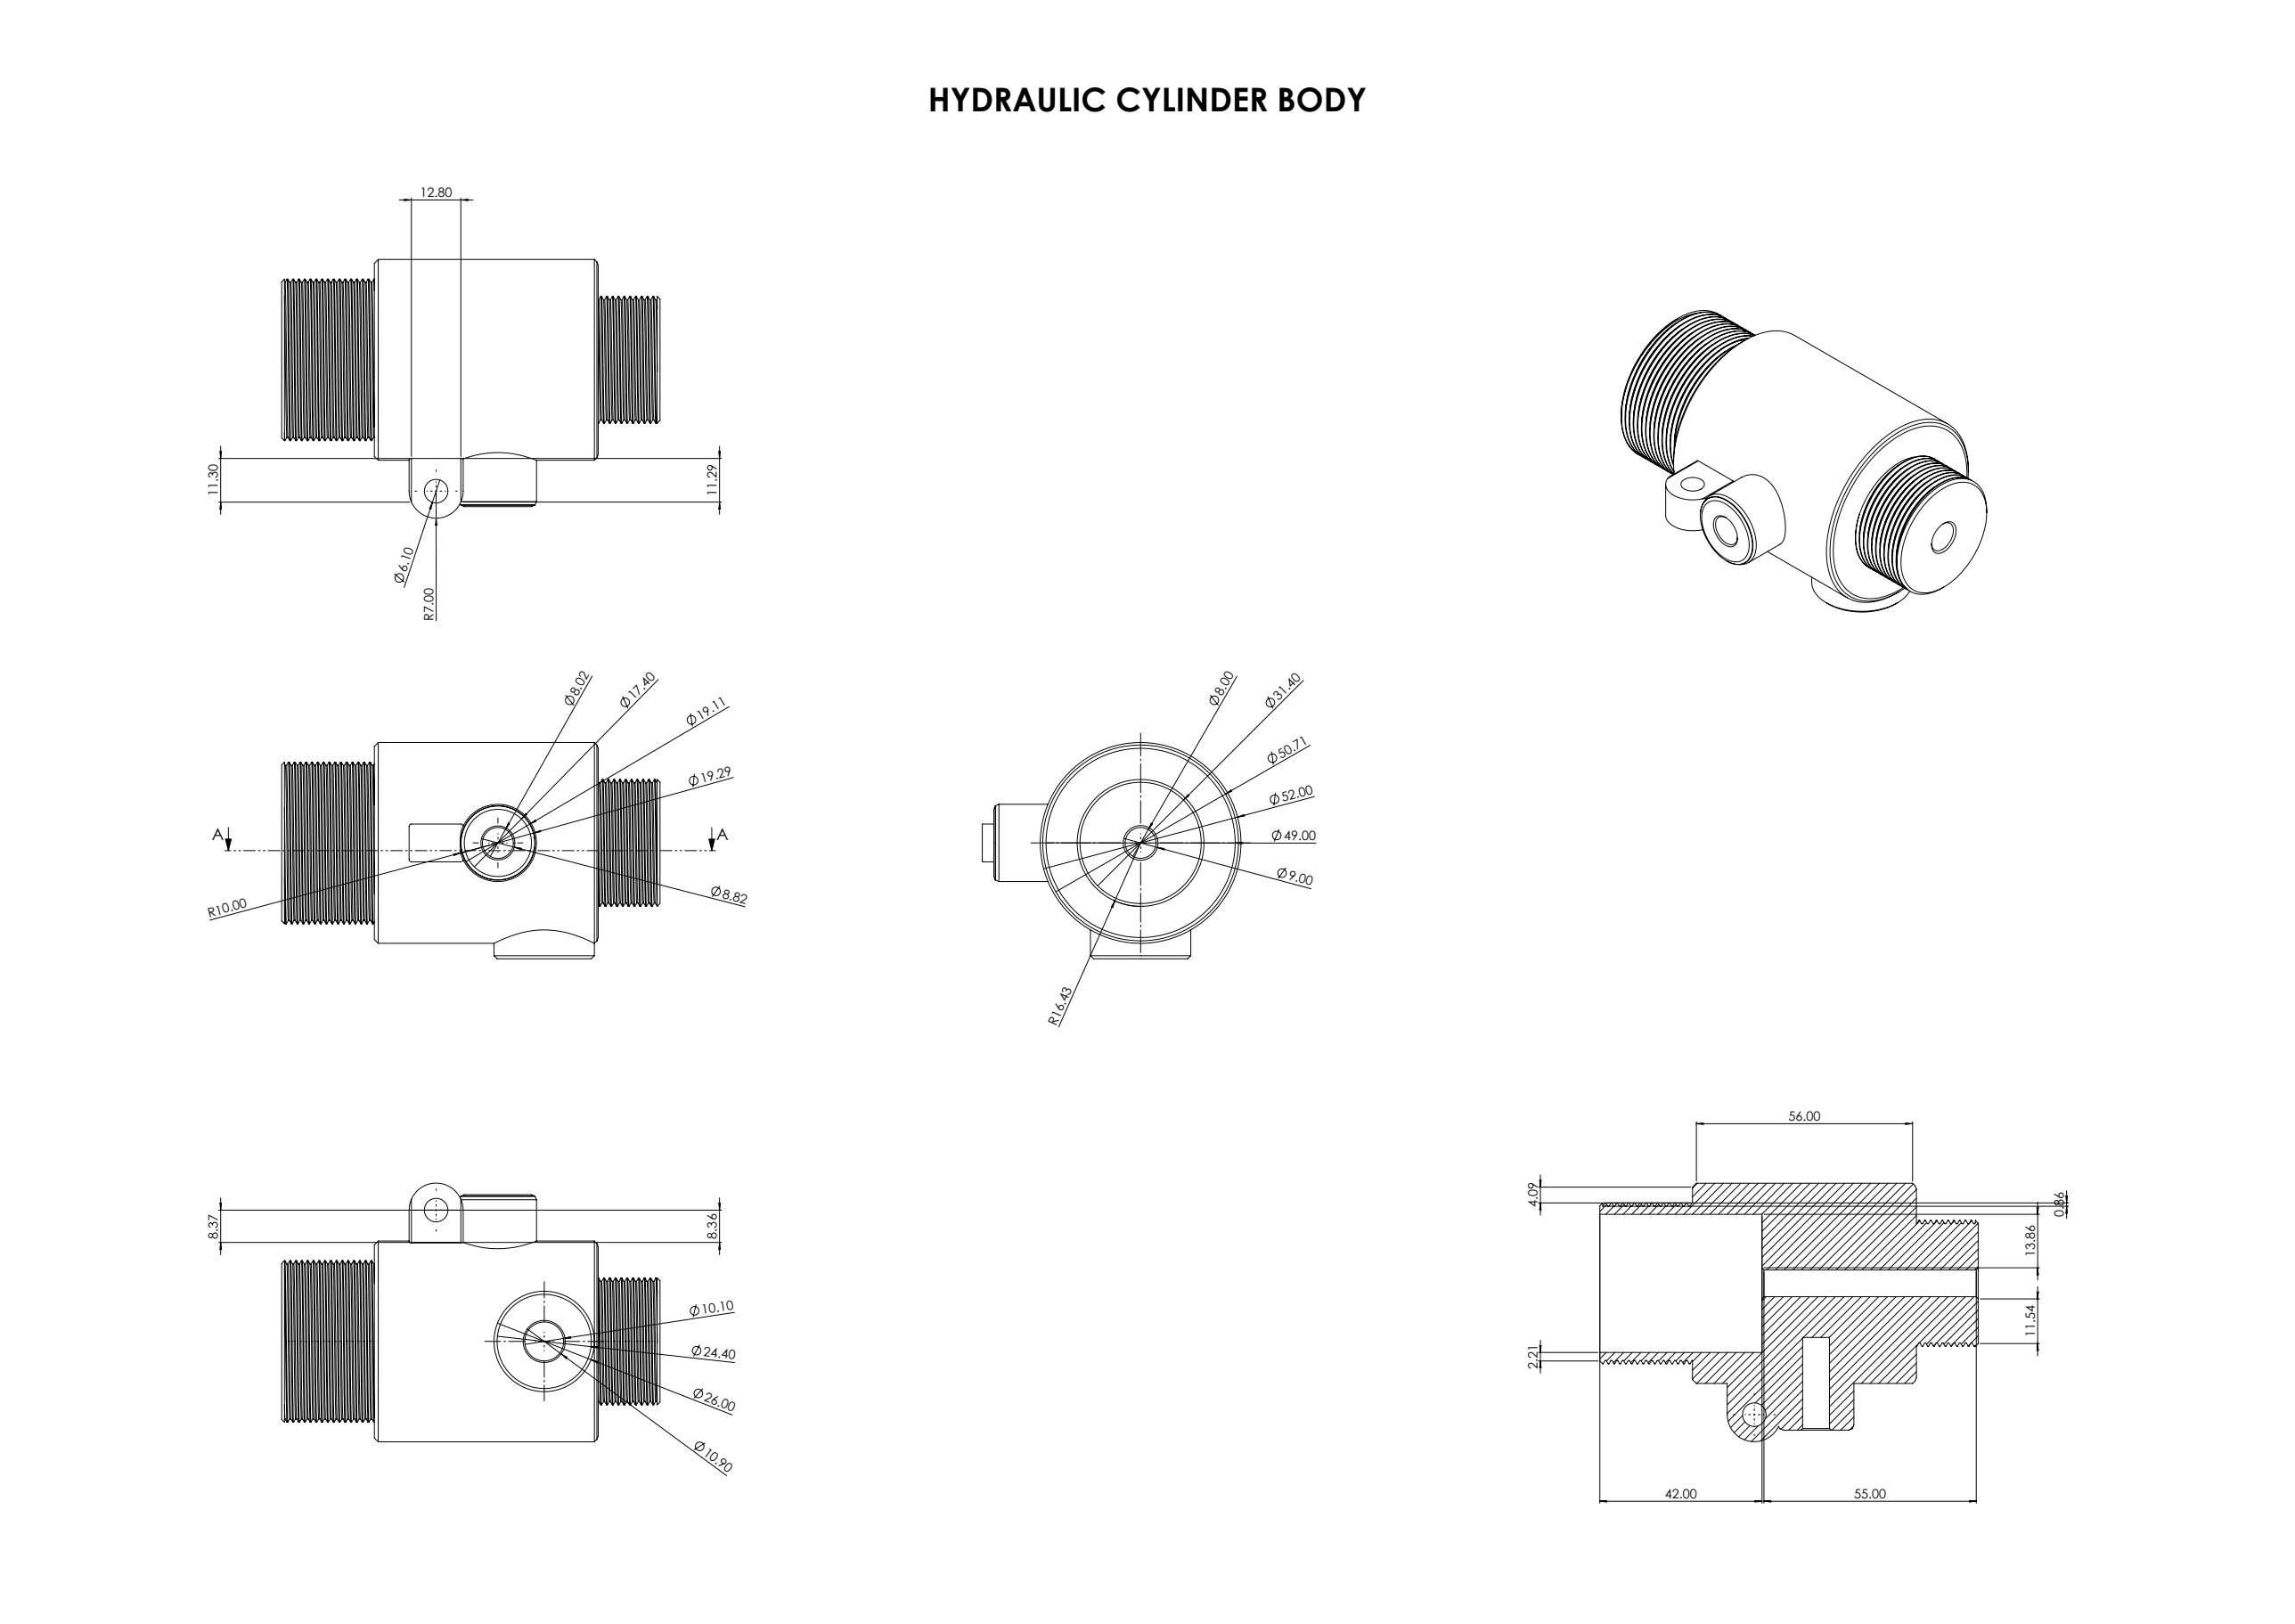
ISO-10303-21;
HEADER;
/* Generated by software containing ST-Developer
 * from STEP Tools, Inc. (www.steptools.com) 
 */

FILE_DESCRIPTION(
/* description */ (''),
/* implementation_level */ '2;1');

FILE_NAME(
/* name */ '02_Hydraulic_Cylinder_Body.step',
/* time_stamp */ '2026-10-26T03:55:20-07:00',
/* author */ (''),
/* organization */ (''),
/* preprocessor_version */ 'ST-DEVELOPER v20.2',
/* originating_system */ 'Autodesk Translation Framework v15.15.0.0',
/* authorisation */ '');

FILE_SCHEMA (('AUTOMOTIVE_DESIGN { 1 0 10303 214 3 1 1 }'));
ENDSEC;

DATA;
#10=MECHANICAL_DESIGN_GEOMETRIC_PRESENTATION_REPRESENTATION('',(#176),#45236);
#136=SHAPE_REPRESENTATION_RELATIONSHIP('SRR','None',#45315,#156);
#156=ADVANCED_BREP_SHAPE_REPRESENTATION('',(#196),#45217);
#176=STYLED_ITEM('',(#45463),#196);
#196=MANIFOLD_SOLID_BREP('Body1',#16518);
#350=B_SPLINE_CURVE_WITH_KNOTS('',3,(#23915,#23916,#23917,#23918,#23919,
#23920,#23921,#23922,#23923,#23924,#23925,#23926,#23927,#23928,#23929,#23930),
 .UNSPECIFIED.,.F.,.F.,(4,3,3,3,3,4),(-4.09299088010945,-3.98286471232789,
-3.4850066232869,-2.98714853424591,-2.48929044520493,-2.07752579179387),
 .UNSPECIFIED.);
#351=B_SPLINE_CURVE_WITH_KNOTS('',3,(#23933,#23934,#23935,#23936,#23937,
#23938,#23939,#23940,#23941,#23942),.UNSPECIFIED.,.F.,.F.,(4,3,3,4),(0.,
0.497858089040978,0.99571617808196,1.12612756527411),.UNSPECIFIED.);
#352=B_SPLINE_CURVE_WITH_KNOTS('',3,(#23947,#23948,#23949,#23950,#23951,
#23952,#23953,#23954,#23955,#23956,#23957,#23958,#23959,#23960,#23961,#23962,
#23963,#23964,#23965,#23966,#23967,#23968,#23969,#23970,#23971,#23972,#23973,
#23974,#23975,#23976,#23977,#23978,#23979,#23980,#23981,#23982,#23983,#23984,
#23985,#23986),.UNSPECIFIED.,.F.,.F.,(4,3,3,3,3,3,3,3,3,3,3,3,3,4),(-10.376176187289,
-9.95716178081971,-9.45930369177872,-8.96144560273774,-8.46358751369675,
-7.96572942465577,-7.46787133561478,-6.9700132465738,-6.47215515753281,
-5.97429706849183,-5.47643897945084,-4.97858089040986,-4.48072280136887,
-4.09299088010945),.UNSPECIFIED.);
#353=B_SPLINE_CURVE_WITH_KNOTS('',3,(#23987,#23988,#23989,#23990,#23991,
#23992,#23993,#23994,#23995,#23996,#23997,#23998,#23999,#24000,#24001,#24002,
#24003,#24004,#24005,#24006,#24007,#24008,#24009,#24010,#24011,#24012,#24013,
#24014,#24015,#24016,#24017,#24018,#24019,#24020,#24021,#24022,#24023,#24024,
#24025,#24026),.UNSPECIFIED.,.F.,.F.,(4,3,3,3,3,3,3,3,3,3,3,3,3,4),(1.12612756527411,
1.49357426712295,1.99143235616393,2.48929044520492,2.98714853424591,3.48500662328689,
3.98286471232788,4.48072280136887,4.97858089040986,5.47643897945084,5.97429706849183,
6.47215515753282,6.9700132465738,7.40931287245371),.UNSPECIFIED.);
#354=B_SPLINE_CURVE_WITH_KNOTS('',3,(#24031,#24032,#24033,#24034,#24035,
#24036,#24037,#24038,#24039,#24040,#24041,#24042,#24043,#24044,#24045,#24046,
#24047,#24048,#24049,#24050,#24051,#24052,#24053,#24054,#24055,#24056,#24057,
#24058,#24059,#24060,#24061,#24062,#24063,#24064,#24065,#24066,#24067,#24068,
#24069,#24070,#24071,#24072,#24073),.UNSPECIFIED.,.F.,.F.,(4,3,3,3,3,3,
3,3,3,3,3,3,3,3,4),(-16.6593614944686,-16.4293169383525,-15.9314588493115,
-15.4336007602705,-14.9357426712296,-14.4378845821886,-13.9400264931476,
-13.4421684041066,-12.9443103150656,-12.4464522260246,-11.9485941369836,
-11.4507360479427,-10.9528779589017,-10.4550198698607,-10.376176187289),
 .UNSPECIFIED.);
#355=B_SPLINE_CURVE_WITH_KNOTS('',3,(#24074,#24075,#24076,#24077,#24078,
#24079,#24080,#24081,#24082,#24083,#24084,#24085,#24086,#24087,#24088,#24089,
#24090,#24091,#24092,#24093,#24094,#24095,#24096,#24097,#24098,#24099,#24100,
#24101,#24102,#24103,#24104,#24105,#24106,#24107,#24108,#24109,#24110,#24111,
#24112,#24113,#24114,#24115,#24116),.UNSPECIFIED.,.F.,.F.,(4,3,3,3,3,3,
3,3,3,3,3,3,3,3,4),(7.40931287245371,7.46787133561479,7.96572942465578,
8.46358751369676,8.96144560273774,9.45930369177873,9.95716178081971,10.4550198698607,
10.9528779589017,11.4507360479427,11.9485941369836,12.4464522260246,12.9443103150656,
13.4421684041066,13.6924981796333),.UNSPECIFIED.);
#356=B_SPLINE_CURVE_WITH_KNOTS('',3,(#24121,#24122,#24123,#24124,#24125,
#24126,#24127,#24128,#24129,#24130,#24131,#24132,#24133,#24134,#24135,#24136,
#24137,#24138,#24139,#24140,#24141,#24142,#24143,#24144,#24145,#24146,#24147,
#24148,#24149,#24150,#24151,#24152,#24153,#24154,#24155,#24156,#24157,#24158,
#24159,#24160,#24161,#24162,#24163),.UNSPECIFIED.,.F.,.F.,(4,3,3,3,3,3,
3,3,3,3,3,3,3,3,4),(-22.9425468016482,-22.9014720958853,-22.4036140068443,
-21.9057559178034,-21.4078978287624,-20.9100397397214,-20.4121816506804,
-19.9143235616394,-19.4164654725984,-18.9186073835574,-18.4207492945165,
-17.9228912054755,-17.4250331164345,-16.9271750273935,-16.6593614944686),
 .UNSPECIFIED.);
#357=B_SPLINE_CURVE_WITH_KNOTS('',3,(#24164,#24165,#24166,#24167,#24168,
#24169,#24170,#24171,#24172,#24173,#24174,#24175,#24176,#24177,#24178,#24179,
#24180,#24181,#24182,#24183,#24184,#24185,#24186,#24187,#24188,#24189,#24190,
#24191,#24192,#24193,#24194,#24195,#24196,#24197,#24198,#24199,#24200,#24201,
#24202,#24203,#24204,#24205,#24206),.UNSPECIFIED.,.F.,.F.,(4,3,3,3,3,3,
3,3,3,3,3,3,3,3,4),(13.6924981796333,13.9400264931476,14.4378845821886,
14.9357426712296,15.4336007602705,15.9314588493115,16.4293169383525,16.9271750273935,
17.4250331164345,17.9228912054755,18.4207492945165,18.9186073835575,19.4164654725984,
19.9143235616394,19.9756834868129),.UNSPECIFIED.);
#358=B_SPLINE_CURVE_WITH_KNOTS('',3,(#24211,#24212,#24213,#24214,#24215,
#24216,#24217,#24218,#24219,#24220,#24221,#24222,#24223,#24224,#24225,#24226,
#24227,#24228,#24229,#24230,#24231,#24232,#24233,#24234,#24235,#24236,#24237,
#24238,#24239,#24240,#24241,#24242,#24243,#24244,#24245,#24246,#24247,#24248,
#24249,#24250),.UNSPECIFIED.,.F.,.F.,(4,3,3,3,3,3,3,3,3,3,3,3,3,4),(-29.2257321088278,
-28.8757691643771,-28.3779110753362,-27.8800529862952,-27.3821948972542,
-26.8843368082132,-26.3864787191722,-25.8886206301312,-25.3907625410903,
-24.8929044520493,-24.3950463630083,-23.8971882739673,-23.3993301849263,
-22.9425468016482),.UNSPECIFIED.);
#359=B_SPLINE_CURVE_WITH_KNOTS('',3,(#24251,#24252,#24253,#24254,#24255,
#24256,#24257,#24258,#24259,#24260,#24261,#24262,#24263,#24264,#24265,#24266,
#24267,#24268,#24269,#24270,#24271,#24272,#24273,#24274,#24275,#24276,#24277,
#24278,#24279,#24280,#24281,#24282,#24283,#24284,#24285,#24286,#24287,#24288,
#24289,#24290),.UNSPECIFIED.,.F.,.F.,(4,3,3,3,3,3,3,3,3,3,3,3,3,4),(19.9756834868129,
20.4121816506804,20.9100397397214,21.4078978287624,21.9057559178034,22.4036140068443,
22.9014720958853,23.3993301849263,23.8971882739673,24.3950463630083,24.8929044520493,
25.3907625410903,25.8886206301312,26.2588687939925),.UNSPECIFIED.);
#360=B_SPLINE_CURVE_WITH_KNOTS('',3,(#24295,#24296,#24297,#24298,#24299,
#24300,#24301,#24302,#24303,#24304,#24305,#24306,#24307,#24308,#24309,#24310,
#24311,#24312,#24313,#24314,#24315,#24316,#24317,#24318,#24319,#24320,#24321,
#24322,#24323,#24324,#24325,#24326,#24327,#24328,#24329,#24330,#24331,#24332,
#24333,#24334,#24335,#24336,#24337),.UNSPECIFIED.,.F.,.F.,(4,3,3,3,3,3,
3,3,3,3,3,3,3,3,4),(-35.5089174160074,-35.34792432191,-34.850066232869,
-34.352208143828,-33.854350054787,-33.356491965746,-32.858633876705,-32.3607757876641,
-31.8629176986231,-31.3650596095821,-30.8672015205411,-30.3693434315001,
-29.8714853424591,-29.3736272534181,-29.2257321088278),.UNSPECIFIED.);
#361=B_SPLINE_CURVE_WITH_KNOTS('',3,(#24338,#24339,#24340,#24341,#24342,
#24343,#24344,#24345,#24346,#24347,#24348,#24349,#24350,#24351,#24352,#24353,
#24354,#24355,#24356,#24357,#24358,#24359,#24360,#24361,#24362,#24363,#24364,
#24365,#24366,#24367,#24368,#24369,#24370,#24371,#24372,#24373,#24374,#24375,
#24376,#24377,#24378,#24379,#24380),.UNSPECIFIED.,.F.,.F.,(4,3,3,3,3,3,
3,3,3,3,3,3,3,3,4),(26.2588687939925,26.3864787191722,26.8843368082132,
27.3821948972542,27.8800529862952,28.3779110753362,28.8757691643771,29.3736272534181,
29.8714853424591,30.3693434315001,30.8672015205411,31.3650596095821,31.8629176986231,
32.3607757876641,32.542054101172),.UNSPECIFIED.);
#362=B_SPLINE_CURVE_WITH_KNOTS('',3,(#24385,#24386,#24387,#24388,#24389,
#24390,#24391,#24392,#24393,#24394,#24395,#24396,#24397,#24398,#24399,#24400,
#24401,#24402,#24403,#24404,#24405,#24406,#24407,#24408,#24409,#24410,#24411,
#24412,#24413,#24414,#24415,#24416,#24417,#24418,#24419,#24420,#24421,#24422,
#24423,#24424),.UNSPECIFIED.,.F.,.F.,(4,3,3,3,3,3,3,3,3,3,3,3,3,4),(-41.792102723187,
-41.3222213904018,-40.8243633013608,-40.3265052123198,-39.8286471232788,
-39.3307890342378,-38.8329309451969,-38.3350728561559,-37.8372147671149,
-37.3393566780739,-36.8414985890329,-36.3436404999919,-35.8457824109509,
-35.5089174160074),.UNSPECIFIED.);
#363=B_SPLINE_CURVE_WITH_KNOTS('',3,(#24425,#24426,#24427,#24428,#24429,
#24430,#24431,#24432,#24433,#24434,#24435,#24436,#24437,#24438,#24439,#24440,
#24441,#24442,#24443,#24444,#24445,#24446,#24447,#24448,#24449,#24450,#24451,
#24452,#24453,#24454,#24455,#24456,#24457,#24458,#24459,#24460,#24461,#24462,
#24463,#24464),.UNSPECIFIED.,.F.,.F.,(4,3,3,3,3,3,3,3,3,3,3,3,3,4),(32.542054101172,
32.858633876705,33.356491965746,33.854350054787,34.352208143828,34.850066232869,
35.34792432191,35.845782410951,36.3436404999919,36.8414985890329,37.3393566780739,
37.8372147671149,38.3350728561559,38.8252394083516),.UNSPECIFIED.);
#364=B_SPLINE_CURVE_WITH_KNOTS('',3,(#24469,#24470,#24471,#24472,#24473,
#24474,#24475,#24476,#24477,#24478,#24479,#24480,#24481,#24482,#24483,#24484,
#24485,#24486,#24487,#24488,#24489,#24490,#24491,#24492,#24493,#24494,#24495,
#24496,#24497,#24498,#24499,#24500,#24501,#24502,#24503,#24504,#24505,#24506,
#24507,#24508,#24509,#24510,#24511),.UNSPECIFIED.,.F.,.F.,(4,3,3,3,3,3,
3,3,3,3,3,3,3,3,4),(-48.0752880303665,-47.7943765479346,-47.2965184588936,
-46.7986603698526,-46.3008022808116,-45.8029441917706,-45.3050861027297,
-44.8072280136887,-44.3093699246477,-43.8115118356067,-43.3136537465657,
-42.8157956575247,-42.3179375684838,-41.8200794794428,-41.792102723187),
 .UNSPECIFIED.);
#365=B_SPLINE_CURVE_WITH_KNOTS('',3,(#24512,#24513,#24514,#24515,#24516,
#24517,#24518,#24519,#24520,#24521,#24522,#24523,#24524,#24525,#24526,#24527,
#24528,#24529,#24530,#24531,#24532,#24533,#24534,#24535,#24536,#24537,#24538,
#24539,#24540,#24541,#24542,#24543,#24544,#24545,#24546,#24547,#24548,#24549,
#24550,#24551,#24552,#24553,#24554),.UNSPECIFIED.,.F.,.F.,(4,3,3,3,3,3,
3,3,3,3,3,3,3,3,4),(38.8252394083516,38.8329309451969,39.3307890342379,
39.8286471232788,40.3265052123198,40.8243633013608,41.3222213904018,41.8200794794428,
42.3179375684838,42.8157956575247,43.3136537465657,43.8115118356067,44.3093699246477,
44.8072280136887,45.1084247155312),.UNSPECIFIED.);
#366=B_SPLINE_CURVE_WITH_KNOTS('',3,(#24559,#24560,#24561,#24562,#24563,
#24564,#24565,#24566,#24567,#24568,#24569,#24570,#24571,#24572,#24573,#24574,
#24575,#24576,#24577,#24578,#24579,#24580,#24581,#24582,#24583,#24584,#24585,
#24586,#24587,#24588,#24589,#24590,#24591,#24592,#24593,#24594,#24595,#24596,
#24597,#24598,#24599,#24600,#24601),.UNSPECIFIED.,.F.,.F.,(4,3,3,3,3,3,
3,3,3,3,3,3,3,3,4),(-54.3584733375462,-54.2665317054674,-53.7686736164264,
-53.2708155273854,-52.7729574383444,-52.2750993493035,-51.7772412602625,
-51.2793831712215,-50.7815250821805,-50.2836669931395,-49.7858089040985,
-49.2879508150576,-48.7900927260166,-48.2922346369756,-48.0752880303665),
 .UNSPECIFIED.);
#367=B_SPLINE_CURVE_WITH_KNOTS('',3,(#24602,#24603,#24604,#24605,#24606,
#24607,#24608,#24609,#24610,#24611,#24612,#24613,#24614,#24615,#24616,#24617,
#24618,#24619,#24620,#24621,#24622,#24623,#24624,#24625,#24626,#24627,#24628,
#24629,#24630,#24631,#24632,#24633,#24634,#24635,#24636,#24637,#24638,#24639,
#24640,#24641,#24642,#24643,#24644),.UNSPECIFIED.,.F.,.F.,(4,3,3,3,3,3,
3,3,3,3,3,3,3,3,4),(45.1084247155312,45.3050861027297,45.8029441917707,
46.3008022808116,46.7986603698526,47.2965184588936,47.7943765479346,48.2922346369756,
48.7900927260166,49.2879508150575,49.7858089040985,50.2836669931395,50.7815250821805,
51.2793831712215,51.3916100227108),.UNSPECIFIED.);
#368=B_SPLINE_CURVE_WITH_KNOTS('',3,(#24649,#24650,#24651,#24652,#24653,
#24654,#24655,#24656,#24657,#24658,#24659,#24660,#24661,#24662,#24663,#24664,
#24665,#24666,#24667,#24668,#24669,#24670,#24671,#24672,#24673,#24674,#24675,
#24676,#24677,#24678,#24679,#24680,#24681,#24682,#24683,#24684,#24685,#24686,
#24687,#24688),.UNSPECIFIED.,.F.,.F.,(4,3,3,3,3,3,3,3,3,3,3,3,3,4),(-60.6416586447257,
-60.2408287739593,-59.7429706849182,-59.2451125958773,-58.7472545068363,
-58.2493964177953,-57.7515383287543,-57.2536802397133,-56.7558221506723,
-56.2579640616314,-55.7601059725904,-55.2622478835494,-54.7643897945084,
-54.3584733375462),.UNSPECIFIED.);
#369=B_SPLINE_CURVE_WITH_KNOTS('',3,(#24689,#24690,#24691,#24692,#24693,
#24694,#24695,#24696,#24697,#24698,#24699,#24700,#24701,#24702,#24703,#24704,
#24705,#24706,#24707,#24708,#24709,#24710,#24711,#24712,#24713,#24714,#24715,
#24716,#24717,#24718,#24719,#24720,#24721,#24722,#24723,#24724,#24725,#24726,
#24727,#24728),.UNSPECIFIED.,.F.,.F.,(4,3,3,3,3,3,3,3,3,3,3,3,3,4),(51.3916100227108,
51.7772412602625,52.2750993493035,52.7729574383445,53.2708155273854,53.7686736164264,
54.2665317054674,54.7643897945084,55.2622478835494,55.7601059725904,56.2579640616314,
56.7558221506723,57.2536802397133,57.6747953298904),.UNSPECIFIED.);
#370=B_SPLINE_CURVE_WITH_KNOTS('',3,(#24733,#24734,#24735,#24736,#24737,
#24738,#24739,#24740,#24741,#24742,#24743,#24744,#24745,#24746,#24747,#24748,
#24749,#24750,#24751,#24752,#24753,#24754,#24755,#24756,#24757,#24758,#24759,
#24760,#24761,#24762,#24763,#24764,#24765,#24766,#24767,#24768,#24769,#24770,
#24771,#24772,#24773,#24774,#24775),.UNSPECIFIED.,.F.,.F.,(4,3,3,3,3,3,
3,3,3,3,3,3,3,3,4),(-66.9248439519053,-66.712983931492,-66.215125842451,
-65.7172677534101,-65.2194096643691,-64.7215515753281,-64.2236934862871,
-63.7258353972461,-63.2279773082051,-62.7301192191642,-62.2322611301232,
-61.7344030410822,-61.2365449520412,-60.7386868630002,-60.6416586447257),
 .UNSPECIFIED.);
#371=B_SPLINE_CURVE_WITH_KNOTS('',3,(#24776,#24777,#24778,#24779,#24780,
#24781,#24782,#24783,#24784,#24785,#24786,#24787,#24788,#24789,#24790,#24791,
#24792,#24793,#24794,#24795,#24796,#24797,#24798,#24799,#24800,#24801,#24802,
#24803,#24804,#24805,#24806,#24807,#24808,#24809,#24810,#24811,#24812,#24813,
#24814,#24815,#24816,#24817,#24818),.UNSPECIFIED.,.F.,.F.,(4,3,3,3,3,3,
3,3,3,3,3,3,3,3,4),(57.6747953298904,57.7515383287543,58.2493964177953,
58.7472545068363,59.2451125958773,59.7429706849182,60.2408287739592,60.7386868630002,
61.2365449520412,61.7344030410822,62.2322611301232,62.7301192191642,63.2279773082051,
63.7258353972461,63.95798063707),.UNSPECIFIED.);
#372=B_SPLINE_CURVE_WITH_KNOTS('',3,(#24823,#24824,#24825,#24826,#24827,
#24828,#24829,#24830,#24831,#24832,#24833,#24834,#24835,#24836,#24837,#24838,
#24839,#24840,#24841,#24842,#24843,#24844,#24845,#24846,#24847,#24848,#24849,
#24850,#24851,#24852,#24853,#24854,#24855,#24856,#24857,#24858,#24859,#24860,
#24861,#24862,#24863,#24864,#24865),.UNSPECIFIED.,.F.,.F.,(4,3,3,3,3,3,
3,3,3,3,3,3,3,3,4),(-73.2080292590849,-73.1851390890248,-72.6872809999838,
-72.1894229109429,-71.6915648219019,-71.1937067328609,-70.6958486438199,
-70.1979905547789,-69.7001324657379,-69.202274376697,-68.704416287656,-68.206558198615,
-67.708700109574,-67.210842020533,-66.9248439519053),.UNSPECIFIED.);
#373=B_SPLINE_CURVE_WITH_KNOTS('',3,(#24866,#24867,#24868,#24869,#24870,
#24871,#24872,#24873,#24874,#24875,#24876,#24877,#24878,#24879,#24880,#24881,
#24882,#24883,#24884,#24885,#24886,#24887,#24888,#24889,#24890,#24891,#24892,
#24893,#24894,#24895,#24896,#24897,#24898,#24899,#24900,#24901,#24902,#24903,
#24904,#24905,#24906,#24907,#24908),.UNSPECIFIED.,.F.,.F.,(4,3,3,3,3,3,
3,3,3,3,3,3,3,3,4),(63.95798063707,64.2236934862871,64.7215515753281,65.2194096643691,
65.7172677534101,66.2151258424511,66.712983931492,67.210842020533,67.708700109574,
68.206558198615,68.704416287656,69.202274376697,69.700132465738,70.1979905547789,
70.2411659442496),.UNSPECIFIED.);
#374=B_SPLINE_CURVE_WITH_KNOTS('',3,(#24913,#24914,#24915,#24916,#24917,
#24918,#24919,#24920,#24921,#24922,#24923,#24924,#24925,#24926,#24927,#24928,
#24929,#24930,#24931,#24932,#24933,#24934,#24935,#24936,#24937,#24938,#24939,
#24940,#24941,#24942,#24943,#24944,#24945,#24946,#24947,#24948,#24949,#24950,
#24951,#24952),.UNSPECIFIED.,.F.,.F.,(4,3,3,3,3,3,3,3,3,3,3,3,3,4),(-79.4912145662645,
-79.1594361575167,-78.6615780684757,-78.1637199794347,-77.6658618903937,
-77.1680038013527,-76.6701457123117,-76.1722876232708,-75.6744295342298,
-75.1765714451888,-74.6787133561478,-74.1808552671068,-73.6829971780658,
-73.2080292590849),.UNSPECIFIED.);
#375=B_SPLINE_CURVE_WITH_KNOTS('',3,(#24953,#24954,#24955,#24956,#24957,
#24958,#24959,#24960,#24961,#24962,#24963,#24964,#24965,#24966,#24967,#24968,
#24969,#24970,#24971,#24972,#24973,#24974,#24975,#24976,#24977,#24978,#24979,
#24980,#24981,#24982,#24983,#24984,#24985,#24986,#24987,#24988,#24989,#24990,
#24991,#24992),.UNSPECIFIED.,.F.,.F.,(4,3,3,3,3,3,3,3,3,3,3,3,3,4),(70.2411659442496,
70.6958486438199,71.1937067328609,71.6915648219019,72.1894229109429,72.6872809999839,
73.1851390890248,73.6829971780658,74.1808552671068,74.6787133561478,75.1765714451888,
75.6744295342298,76.1722876232707,76.5243512514292),.UNSPECIFIED.);
#376=B_SPLINE_CURVE_WITH_KNOTS('',3,(#24997,#24998,#24999,#25000,#25001,
#25002,#25003,#25004,#25005,#25006,#25007,#25008,#25009,#25010,#25011,#25012,
#25013,#25014,#25015,#25016,#25017,#25018,#25019,#25020,#25021,#25022,#25023,
#25024,#25025,#25026,#25027,#25028,#25029,#25030,#25031,#25032,#25033,#25034,
#25035,#25036,#25037,#25038,#25039),.UNSPECIFIED.,.F.,.F.,(4,3,3,3,3,3,
3,3,3,3,3,3,3,3,4),(-85.7743998734441,-85.6315913150495,-85.1337332260085,
-84.6358751369675,-84.1380170479265,-83.6401589588856,-83.1423008698446,
-82.6444427808036,-82.1465846917626,-81.6487266027216,-81.1508685136806,
-80.6530104246396,-80.1551523355986,-79.6572942465577,-79.4912145662645),
 .UNSPECIFIED.);
#377=B_SPLINE_CURVE_WITH_KNOTS('',3,(#25040,#25041,#25042,#25043,#25044,
#25045,#25046,#25047,#25048,#25049,#25050,#25051,#25052,#25053,#25054,#25055,
#25056,#25057,#25058,#25059,#25060,#25061,#25062,#25063,#25064,#25065,#25066,
#25067,#25068,#25069,#25070,#25071,#25072,#25073,#25074,#25075,#25076,#25077,
#25078,#25079,#25080,#25081,#25082),.UNSPECIFIED.,.F.,.F.,(4,3,3,3,3,3,
3,3,3,3,3,3,3,3,4),(76.5243512514292,76.6701457123117,77.1680038013527,
77.6658618903937,78.1637199794347,78.6615780684757,79.1594361575167,79.6572942465577,
80.1551523355986,80.6530104246396,81.1508685136806,81.6487266027216,82.1465846917626,
82.6444427808036,82.8075365586088),.UNSPECIFIED.);
#378=B_SPLINE_CURVE_WITH_KNOTS('',3,(#25087,#25088,#25089,#25090,#25091,
#25092,#25093,#25094,#25095,#25096,#25097,#25098,#25099,#25100,#25101,#25102,
#25103,#25104,#25105,#25106,#25107,#25108,#25109,#25110,#25111,#25112,#25113,
#25114,#25115,#25116,#25117,#25118,#25119,#25120,#25121,#25122,#25123,#25124,
#25125,#25126),.UNSPECIFIED.,.F.,.F.,(4,3,3,3,3,3,3,3,3,3,3,3,3,4),(-92.0575851806237,
-91.6058883835413,-91.1080302945003,-90.6101722054593,-90.1123141164184,
-89.6144560273774,-89.1165979383364,-88.6187398492954,-88.1208817602544,
-87.6230236712134,-87.1251655821724,-86.6273074931315,-86.1294494040905,
-85.7743998734441),.UNSPECIFIED.);
#379=B_SPLINE_CURVE_WITH_KNOTS('',3,(#25127,#25128,#25129,#25130,#25131,
#25132,#25133,#25134,#25135,#25136,#25137,#25138,#25139,#25140,#25141,#25142,
#25143,#25144,#25145,#25146,#25147,#25148,#25149,#25150,#25151,#25152,#25153,
#25154,#25155,#25156,#25157,#25158,#25159,#25160,#25161,#25162,#25163,#25164,
#25165,#25166),.UNSPECIFIED.,.F.,.F.,(4,3,3,3,3,3,3,3,3,3,3,3,3,4),(82.8075365586088,
83.1423008698446,83.6401589588855,84.1380170479265,84.6358751369675,85.1337332260085,
85.6315913150495,86.1294494040905,86.6273074931315,87.1251655821725,87.6230236712134,
88.1208817602544,88.6187398492954,89.0907218657884),.UNSPECIFIED.);
#380=B_SPLINE_CURVE_WITH_KNOTS('',3,(#25171,#25172,#25173,#25174,#25175,
#25176,#25177,#25178,#25179,#25180,#25181,#25182,#25183,#25184,#25185,#25186,
#25187,#25188,#25189,#25190,#25191,#25192,#25193,#25194,#25195,#25196,#25197,
#25198,#25199,#25200,#25201,#25202,#25203,#25204,#25205,#25206,#25207,#25208,
#25209,#25210,#25211,#25212,#25213),.UNSPECIFIED.,.F.,.F.,(4,3,3,3,3,3,
3,3,3,3,3,3,3,3,4),(-98.3407704878033,-98.0780435410741,-97.5801854520331,
-97.0823273629921,-96.5844692739512,-96.0866111849102,-95.5887530958692,
-95.0908950068282,-94.5930369177872,-94.0951788287462,-93.5973207397052,
-93.0994626506643,-92.6016045616233,-92.1037464725823,-92.0575851806237),
 .UNSPECIFIED.);
#381=B_SPLINE_CURVE_WITH_KNOTS('',3,(#25214,#25215,#25216,#25217,#25218,
#25219,#25220,#25221,#25222,#25223,#25224,#25225,#25226,#25227,#25228,#25229,
#25230,#25231,#25232,#25233,#25234,#25235,#25236,#25237,#25238,#25239,#25240,
#25241,#25242,#25243,#25244,#25245,#25246,#25247,#25248,#25249,#25250,#25251,
#25252,#25253,#25254,#25255,#25256),.UNSPECIFIED.,.F.,.F.,(4,3,3,3,3,3,
3,3,3,3,3,3,3,3,4),(89.0907218657884,89.1165979383364,89.6144560273774,
90.1123141164184,90.6101722054593,91.1080302945003,91.6058883835413,92.1037464725823,
92.6016045616233,93.0994626506643,93.5973207397052,94.0951788287462,94.5930369177872,
95.0908950068282,95.373907172968),.UNSPECIFIED.);
#382=B_SPLINE_CURVE_WITH_KNOTS('',3,(#25262,#25263,#25264,#25265,#25266,
#25267,#25268,#25269,#25270,#25271,#25272,#25273,#25274,#25275,#25276),
 .UNSPECIFIED.,.F.,.F.,(4,1,1,1,1,1,1,1,1,1,1,1,4),(103.672557568463,103.718718860422,
104.216576949463,104.714435038504,105.212293127545,105.710151216586,106.208009305627,
106.705867394668,107.203725483709,107.70158357275,108.199441661791,108.697299750832,
109.109064404243),.UNSPECIFIED.);
#383=B_SPLINE_CURVE_WITH_KNOTS('',3,(#25279,#25280,#25281,#25282,#25283,
#25284,#25285,#25286,#25287,#25288,#25289,#25290),.UNSPECIFIED.,.F.,.F.,
(4,1,1,1,1,1,1,1,1,4),(103.672557568463,103.887403491364,104.385261580405,
104.883119669446,105.380977758487,105.878835847528,106.376693936569,106.87455202561,
107.372410114651,107.870268203692),.UNSPECIFIED.);
#384=B_SPLINE_CURVE_WITH_KNOTS('',3,(#25295,#25296,#25297,#25298,#25299,
#25300,#25301,#25302,#25303,#25304,#25305,#25306,#25307,#25308,#25309,#25310),
 .UNSPECIFIED.,.F.,.F.,(4,1,1,1,1,1,1,1,1,1,1,1,1,4),(97.3893722612836,
97.7444217919299,98.2422798809709,98.7401379700119,99.2379960590529,99.7358541480939,
100.233712237135,100.731570326176,101.229428415217,101.727286504258,102.225144593299,
102.72300268234,103.220860771381,103.672557568463),.UNSPECIFIED.);
#385=B_SPLINE_CURVE_WITH_KNOTS('',3,(#25311,#25312,#25313,#25314,#25315,
#25316,#25317,#25318,#25319,#25320,#25321,#25322,#25323,#25324,#25325,#25326,
#25327),.UNSPECIFIED.,.F.,.F.,(4,1,1,1,1,1,1,1,1,1,1,1,1,1,4),(97.3893722612836,
97.4152483338315,97.9131064228725,98.4109645119134,98.9088226009544,99.4066806899954,
99.9045387790364,100.402396868077,100.900254957118,101.398113046159,101.8959711352,
102.393829224241,102.891687313282,103.389545402323,103.672557568463),
 .UNSPECIFIED.);
#386=B_SPLINE_CURVE_WITH_KNOTS('',3,(#25332,#25333,#25334,#25335,#25336,
#25337,#25338,#25339,#25340,#25341,#25342,#25343,#25344,#25345,#25346,#25347,
#25348),.UNSPECIFIED.,.F.,.F.,(4,1,1,1,1,1,1,1,1,1,1,1,1,1,4),(91.106186954104,
91.2722666343971,91.7701247234381,92.2679828124791,92.7658409015201,93.2636989905611,
93.761557079602,94.259415168643,94.757273257684,95.255131346725,95.752989435766,
96.250847524807,96.7487056138479,97.2465637028889,97.3893722612836),
 .UNSPECIFIED.);
#387=B_SPLINE_CURVE_WITH_KNOTS('',3,(#25349,#25350,#25351,#25352,#25353,
#25354,#25355,#25356,#25357,#25358,#25359,#25360,#25361,#25362,#25363,#25364),
 .UNSPECIFIED.,.F.,.F.,(4,1,1,1,1,1,1,1,1,1,1,1,1,4),(91.106186954104,91.4409512653396,
91.9388093543806,92.4366674434216,92.9345255324626,93.4323836215036,93.9302417105446,
94.4280997995856,94.9259578886266,95.4238159776675,95.9216740667085,96.4195321557495,
96.9173902447905,97.3893722612836),.UNSPECIFIED.);
#388=B_SPLINE_CURVE_WITH_KNOTS('',3,(#25369,#25370,#25371,#25372,#25373,
#25374,#25375,#25376,#25377,#25378,#25379,#25380,#25381,#25382,#25383,#25384),
 .UNSPECIFIED.,.F.,.F.,(4,1,1,1,1,1,1,1,1,1,1,1,1,4),(84.8230016469244,
85.2979695659053,85.7958276549463,86.2936857439873,86.7915438330282,87.2894019220692,
87.7872600111102,88.2851181001512,88.7829761891922,89.2808342782332,89.7786923672741,
90.2765504563151,90.7744085453561,91.106186954104),.UNSPECIFIED.);
#389=B_SPLINE_CURVE_WITH_KNOTS('',3,(#25385,#25386,#25387,#25388,#25389,
#25390,#25391,#25392,#25393,#25394,#25395,#25396,#25397,#25398,#25399,#25400,
#25401),.UNSPECIFIED.,.F.,.F.,(4,1,1,1,1,1,1,1,1,1,1,1,1,1,4),(84.8230016469244,
84.9687961078068,85.4666541968478,85.9645122858888,86.4623703749298,86.9602284639708,
87.4580865530118,87.9559446420528,88.4538027310937,88.9516608201347,89.4495189091757,
89.9473769982167,90.4452350872577,90.9430931762987,91.106186954104),
 .UNSPECIFIED.);
#390=B_SPLINE_CURVE_WITH_KNOTS('',3,(#25406,#25407,#25408,#25409,#25410,
#25411,#25412,#25413,#25414,#25415,#25416,#25417,#25418,#25419,#25420,#25421,
#25422),.UNSPECIFIED.,.F.,.F.,(4,1,1,1,1,1,1,1,1,1,1,1,1,1,4),(78.5398163397448,
78.8258144083725,79.3236724974135,79.8215305864545,80.3193886754954,80.8172467645364,
81.3151048535774,81.8129629426184,82.3108210316594,82.8086791207004,83.3065372097414,
83.8043952987823,84.3022533878233,84.8001114768643,84.8230016469244),
 .UNSPECIFIED.);
#391=B_SPLINE_CURVE_WITH_KNOTS('',3,(#25423,#25424,#25425,#25426,#25427,
#25428,#25429,#25430,#25431,#25432,#25433,#25434,#25435,#25436,#25437,#25438),
 .UNSPECIFIED.,.F.,.F.,(4,1,1,1,1,1,1,1,1,1,1,1,1,4),(78.5398163397448,
78.994499039315,79.492357128356,79.990215217397,80.488073306438,80.985931395479,
81.4837894845199,81.9816475735609,82.4795056626019,82.9773637516429,83.4752218406839,
83.9730799297249,84.4709380187658,84.8230016469244),.UNSPECIFIED.);
#392=B_SPLINE_CURVE_WITH_KNOTS('',3,(#25443,#25444,#25445,#25446,#25447,
#25448,#25449,#25450,#25451,#25452,#25453,#25454,#25455,#25456,#25457,#25458,
#25459),.UNSPECIFIED.,.F.,.F.,(4,1,1,1,1,1,1,1,1,1,1,1,1,1,4),(72.2566310325652,
72.3536592508397,72.8515173398807,73.3493754289216,73.8472335179626,74.3450916070036,
74.8429496960446,75.3408077850856,75.8386658741266,76.3365239631676,76.8343820522085,
77.3322401412495,77.8300982302905,78.3279563193315,78.5398163397448),
 .UNSPECIFIED.);
#393=B_SPLINE_CURVE_WITH_KNOTS('',3,(#25460,#25461,#25462,#25463,#25464,
#25465,#25466,#25467,#25468,#25469,#25470,#25471,#25472,#25473,#25474,#25475,
#25476),.UNSPECIFIED.,.F.,.F.,(4,1,1,1,1,1,1,1,1,1,1,1,1,1,4),(72.2566310325652,
72.5223438817822,73.0202019708232,73.5180600598642,74.0159181489052,74.5137762379462,
75.0116343269871,75.5094924160281,76.0073505050691,76.5052085941101,77.0030666831511,
77.5009247721921,77.9987828612331,78.496640950274,78.5398163397448),
 .UNSPECIFIED.);
#394=B_SPLINE_CURVE_WITH_KNOTS('',3,(#25481,#25482,#25483,#25484,#25485,
#25486,#25487,#25488,#25489,#25490,#25491,#25492,#25493,#25494,#25495,#25496),
 .UNSPECIFIED.,.F.,.F.,(4,1,1,1,1,1,1,1,1,1,1,1,1,4),(65.9734457253856,
66.3793621823478,66.8772202713888,67.3750783604298,67.8729364494708,68.3707945385118,
68.8686526275528,69.3665107165938,69.8643688056347,70.3622268946757,70.8600849837167,
71.3579430727577,71.8558011617987,72.2566310325652),.UNSPECIFIED.);
#395=B_SPLINE_CURVE_WITH_KNOTS('',3,(#25497,#25498,#25499,#25500,#25501,
#25502,#25503,#25504,#25505,#25506,#25507,#25508,#25509,#25510,#25511,#25512,
#25513),.UNSPECIFIED.,.F.,.F.,(4,1,1,1,1,1,1,1,1,1,1,1,1,1,4),(65.9734457253856,
66.0501887242494,66.5480468132904,67.0459049023314,67.5437629913723,68.0416210804133,
68.5394791694543,69.0373372584953,69.5351953475363,70.0330534365773,70.5309115256183,
71.0287696146593,71.5266277037002,72.0244857927412,72.2566310325652),
 .UNSPECIFIED.);
#396=B_SPLINE_CURVE_WITH_KNOTS('',3,(#25518,#25519,#25520,#25521,#25522,
#25523,#25524,#25525,#25526,#25527,#25528,#25529,#25530,#25531,#25532,#25533,
#25534),.UNSPECIFIED.,.F.,.F.,(4,1,1,1,1,1,1,1,1,1,1,1,1,1,4),(59.6902604182061,
59.907207024815,60.405065113856,60.902923202897,61.400781291938,61.898639380979,
62.39649747002,62.8943555590609,63.3922136481019,63.8900717371429,64.3879298261839,
64.8857879152249,65.3836460042659,65.8815040933069,65.9734457253856),
 .UNSPECIFIED.);
#397=B_SPLINE_CURVE_WITH_KNOTS('',3,(#25535,#25536,#25537,#25538,#25539,
#25540,#25541,#25542,#25543,#25544,#25545,#25546,#25547,#25548,#25549,#25550),
 .UNSPECIFIED.,.F.,.F.,(4,1,1,1,1,1,1,1,1,1,1,1,1,4),(59.690260418206,60.0758916557576,
60.5737497447986,61.0716078338395,61.5694659228805,62.0673240119215,62.5651821009625,
63.0630401900035,63.5608982790445,64.0587563680855,64.5566144571264,65.0544725461674,
65.5523306352084,65.9734457253856),.UNSPECIFIED.);
#398=B_SPLINE_CURVE_WITH_KNOTS('',3,(#25555,#25556,#25557,#25558,#25559,
#25560,#25561,#25562,#25563,#25564,#25565,#25566,#25567,#25568,#25569,#25570,
#25571),.UNSPECIFIED.,.F.,.F.,(4,1,1,1,1,1,1,1,1,1,1,1,1,1,4),(53.4070751110264,
53.4350518672822,53.9329099563232,54.4307680453642,54.9286261344052,55.4264842234462,
55.9243423124872,56.4222004015281,56.9200584905691,57.4179165796101,57.9157746686511,
58.4136327576921,58.9114908467331,59.409348935774,59.6902604182061),
 .UNSPECIFIED.);
#399=B_SPLINE_CURVE_WITH_KNOTS('',3,(#25572,#25573,#25574,#25575,#25576,
#25577,#25578,#25579,#25580,#25581,#25582,#25583,#25584,#25585,#25586,#25587,
#25588),.UNSPECIFIED.,.F.,.F.,(4,1,1,1,1,1,1,1,1,1,1,1,1,1,4),(53.4070751110264,
53.6037364982248,54.1015945872658,54.5994526763067,55.0973107653477,55.5951688543887,
56.0930269434297,56.5908850324707,57.0887431215117,57.5866012105526,58.0844592995936,
58.5823173886346,59.0801754776756,59.5780335667166,59.690260418206),
 .UNSPECIFIED.);
#400=B_SPLINE_CURVE_WITH_KNOTS('',3,(#25593,#25594,#25595,#25596,#25597,
#25598,#25599,#25600,#25601,#25602,#25603,#25604,#25605,#25606,#25607,#25608),
 .UNSPECIFIED.,.F.,.F.,(4,1,1,1,1,1,1,1,1,1,1,1,1,4),(47.1238898038469,
47.4607547987904,47.9586128878314,48.4564709768724,48.9543290659134,49.4521871549543,
49.9500452439953,50.4479033330363,50.9457614220773,51.4436195111183,51.9414776001593,
52.4393356892003,52.9371937782412,53.4070751110264),.UNSPECIFIED.);
#401=B_SPLINE_CURVE_WITH_KNOTS('',3,(#25609,#25610,#25611,#25612,#25613,
#25614,#25615,#25616,#25617,#25618,#25619,#25620,#25621,#25622,#25623,#25624,
#25625),.UNSPECIFIED.,.F.,.F.,(4,1,1,1,1,1,1,1,1,1,1,1,1,1,4),(47.1238898038469,
47.131581340692,47.6294394297329,48.1272975187739,48.6251556078149,49.1230136968559,
49.6208717858969,50.1187298749379,50.6165879639789,51.1144460530198,51.6123041420608,
52.1101622311018,52.6080203201428,53.1058784091838,53.4070751110264),
 .UNSPECIFIED.);
#402=B_SPLINE_CURVE_WITH_KNOTS('',3,(#25630,#25631,#25632,#25633,#25634,
#25635,#25636,#25637,#25638,#25639,#25640,#25641,#25642,#25643,#25644,#25645,
#25646),.UNSPECIFIED.,.F.,.F.,(4,1,1,1,1,1,1,1,1,1,1,1,1,1,4),(40.8407044966673,
40.9885996412576,41.4864577302986,41.9843158193396,42.4821739083806,42.9800319974215,
43.4778900864625,43.9757481755035,44.4736062645445,44.9714643535855,45.4693224426265,
45.9671805316675,46.4650386207084,46.9628967097494,47.1238898038469),
 .UNSPECIFIED.);
#403=B_SPLINE_CURVE_WITH_KNOTS('',3,(#25647,#25648,#25649,#25650,#25651,
#25652,#25653,#25654,#25655,#25656,#25657,#25658,#25659,#25660,#25661,#25662),
 .UNSPECIFIED.,.F.,.F.,(4,1,1,1,1,1,1,1,1,1,1,1,1,4),(40.8407044966673,
41.1572842722001,41.6551423612411,42.1530004502821,42.6508585393231,43.1487166283641,
43.6465747174051,44.144432806446,44.642290895487,45.140148984528,45.638007073569,
46.13586516261,46.633723251651,47.1238898038469),.UNSPECIFIED.);
#404=B_SPLINE_CURVE_WITH_KNOTS('',3,(#25667,#25668,#25669,#25670,#25671,
#25672,#25673,#25674,#25675,#25676,#25677,#25678,#25679,#25680,#25681,#25682),
 .UNSPECIFIED.,.F.,.F.,(4,1,1,1,1,1,1,1,1,1,1,1,1,4),(34.5575191894876,
35.0143025727658,35.5121606618068,36.0100187508477,36.5078768398887,37.0057349289297,
37.5035930179707,38.0014511070117,38.4993091960527,38.9971672850937,39.4950253741346,
39.9928834631756,40.4907415522166,40.8407044966673),.UNSPECIFIED.);
#405=B_SPLINE_CURVE_WITH_KNOTS('',3,(#25683,#25684,#25685,#25686,#25687,
#25688,#25689,#25690,#25691,#25692,#25693,#25694,#25695,#25696,#25697,#25698,
#25699),.UNSPECIFIED.,.F.,.F.,(4,1,1,1,1,1,1,1,1,1,1,1,1,1,4),(34.5575191894876,
34.6851291146673,35.1829872037083,35.6808452927493,36.1787033817903,36.6765614708313,
37.1744195598722,37.6722776489132,38.1701357379542,38.6679938269952,39.1658519160362,
39.6637100050772,40.1615680941182,40.6594261831592,40.8407044966673),
 .UNSPECIFIED.);
#406=B_SPLINE_CURVE_WITH_KNOTS('',3,(#25704,#25705,#25706,#25707,#25708,
#25709,#25710,#25711,#25712,#25713,#25714,#25715,#25716,#25717,#25718,#25719,
#25720),.UNSPECIFIED.,.F.,.F.,(4,1,1,1,1,1,1,1,1,1,1,1,1,1,4),(28.274333882308,
28.542147415233,29.0400055042739,29.5378635933149,30.0357216823559,30.5335797713969,
31.0314378604379,31.5292959494789,32.0271540385199,32.5250121275608,33.0228702166018,
33.5207283056428,34.0185863946838,34.5164444837248,34.5575191894876),
 .UNSPECIFIED.);
#407=B_SPLINE_CURVE_WITH_KNOTS('',3,(#25721,#25722,#25723,#25724,#25725,
#25726,#25727,#25728,#25729,#25730,#25731,#25732,#25733,#25734,#25735,#25736),
 .UNSPECIFIED.,.F.,.F.,(4,1,1,1,1,1,1,1,1,1,1,1,1,4),(28.274333882308,28.7108320461755,
29.2086901352165,29.7065482242575,30.2044063132985,30.7022644023394,31.2001224913804,
31.6979805804214,32.1958386694624,32.6936967585034,33.1915548475444,33.6894129365854,
34.1872710256263,34.5575191894876),.UNSPECIFIED.);
#408=B_SPLINE_CURVE_WITH_KNOTS('',3,(#25741,#25742,#25743,#25744,#25745,
#25746,#25747,#25748,#25749,#25750,#25751,#25752,#25753,#25754,#25755,#25756,
#25757),.UNSPECIFIED.,.F.,.F.,(4,1,1,1,1,1,1,1,1,1,1,1,1,1,4),(21.9911485751285,
22.0699922577002,22.5678503467411,23.0657084357821,23.5635665248231,24.0614246138641,
24.5592827029051,25.0571407919461,25.554998880987,26.052856970028,26.550715059069,
27.04857314811,27.546431237151,28.044289326192,28.274333882308),
 .UNSPECIFIED.);
#409=B_SPLINE_CURVE_WITH_KNOTS('',3,(#25758,#25759,#25760,#25761,#25762,
#25763,#25764,#25765,#25766,#25767,#25768,#25769,#25770,#25771,#25772,#25773,
#25774),.UNSPECIFIED.,.F.,.F.,(4,1,1,1,1,1,1,1,1,1,1,1,1,1,4),(21.9911485751285,
22.2386768886427,22.7365349776837,23.2343930667247,23.7322511557656,24.2301092448066,
24.7279673338476,25.2258254228886,25.7236835119296,26.2215416009706,26.7193996900116,
27.2172577790525,27.7151158680935,28.2129739571345,28.274333882308),
 .UNSPECIFIED.);
#410=B_SPLINE_CURVE_WITH_KNOTS('',3,(#25779,#25780,#25781,#25782,#25783,
#25784,#25785,#25786,#25787,#25788,#25789,#25790,#25791,#25792,#25793,#25794),
 .UNSPECIFIED.,.F.,.F.,(4,1,1,1,1,1,1,1,1,1,1,1,1,4),(15.7079632679489,
16.0956951892083,16.5935532782493,17.0914113672903,17.5892694563313,18.0871275453723,
18.5849856344133,19.0828437234542,19.5807018124952,20.0785599015362,20.5764179905772,
21.0742760796182,21.5721341686592,21.9911485751285),.UNSPECIFIED.);
#411=B_SPLINE_CURVE_WITH_KNOTS('',3,(#25795,#25796,#25797,#25798,#25799,
#25800,#25801,#25802,#25803,#25804,#25805,#25806,#25807,#25808,#25809,#25810,
#25811),.UNSPECIFIED.,.F.,.F.,(4,1,1,1,1,1,1,1,1,1,1,1,1,1,4),(15.7079632679489,
15.7665217311099,16.2643798201509,16.7622379091919,17.2600959982328,17.7579540872738,
18.2558121763148,18.7536702653558,19.2515283543968,19.7493864434378,20.2472445324787,
20.7451026215197,21.2429607105607,21.7408187996017,21.9911485751285),
 .UNSPECIFIED.);
#412=B_SPLINE_CURVE_WITH_KNOTS('',3,(#25817,#25818,#25819,#25820,#25821,
#25822,#25823,#25824,#25825,#25826,#25827,#25828,#25829,#25830,#25831,#25832),
 .UNSPECIFIED.,.F.,.F.,(4,3,3,3,3,4),(-4.09299088010945,-3.9439579802929,
-3.45096323275628,-2.95796848521967,-2.46497373768306,-2.07752579179387),
 .UNSPECIFIED.);
#413=B_SPLINE_CURVE_WITH_KNOTS('',3,(#25835,#25836,#25837,#25838,#25839,
#25840,#25841,#25842,#25843,#25844),.UNSPECIFIED.,.F.,.F.,(4,3,3,4),(0.,
0.492994747536612,0.985989495073225,1.12612756527419),.UNSPECIFIED.);
#414=B_SPLINE_CURVE_WITH_KNOTS('',3,(#25849,#25850,#25851,#25852,#25853,
#25854,#25855,#25856,#25857,#25858,#25859,#25860,#25861,#25862,#25863,#25864,
#25865,#25866,#25867,#25868,#25869,#25870,#25871,#25872,#25873,#25874,#25875,
#25876,#25877,#25878,#25879,#25880,#25881,#25882,#25883,#25884,#25885,#25886,
#25887,#25888,#25889,#25890,#25891),.UNSPECIFIED.,.F.,.F.,(4,3,3,3,3,3,
3,3,3,3,3,3,3,3,4),(-10.3761761872891,-10.3528896982689,-9.85989495073224,
-9.36690020319563,-8.87390545565902,-8.38091070812241,-7.88791596058579,
-7.39492121304918,-6.90192646551257,-6.40893171797596,-5.91593697043935,
-5.42294222290273,-4.92994747536612,-4.43695272782951,-4.09299088010945),
 .UNSPECIFIED.);
#415=B_SPLINE_CURVE_WITH_KNOTS('',3,(#25892,#25893,#25894,#25895,#25896,
#25897,#25898,#25899,#25900,#25901,#25902,#25903,#25904,#25905,#25906,#25907,
#25908,#25909,#25910,#25911,#25912,#25913,#25914,#25915,#25916,#25917,#25918,
#25919,#25920,#25921,#25922,#25923,#25924,#25925,#25926,#25927,#25928,#25929,
#25930,#25931,#25932,#25933,#25934),.UNSPECIFIED.,.F.,.F.,(4,3,3,3,3,3,
3,3,3,3,3,3,3,3,4),(1.12612756527419,1.47898424260984,1.97197899014645,
2.46497373768306,2.95796848521968,3.45096323275629,3.9439579802929,4.43695272782951,
4.92994747536613,5.42294222290274,5.91593697043935,6.40893171797596,6.90192646551257,
7.39492121304918,7.40931287245371),.UNSPECIFIED.);
#416=B_SPLINE_CURVE_WITH_KNOTS('',3,(#25939,#25940,#25941,#25942,#25943,
#25944,#25945,#25946,#25947,#25948,#25949,#25950,#25951,#25952,#25953,#25954,
#25955,#25956,#25957,#25958,#25959,#25960,#25961,#25962,#25963,#25964,#25965,
#25966,#25967,#25968,#25969,#25970,#25971,#25972,#25973,#25974,#25975,#25976,
#25977,#25978),.UNSPECIFIED.,.F.,.F.,(4,3,3,3,3,3,3,3,3,3,3,3,3,4),(-16.6593614944687,
-16.2688266687082,-15.7758319211716,-15.282837173635,-14.7898424260984,
-14.2968476785617,-13.8038529310251,-13.3108581834885,-12.8178634359519,
-12.3248686884153,-11.8318739408787,-11.3388791933421,-10.8458844458055,
-10.3761761872891),.UNSPECIFIED.);
#417=B_SPLINE_CURVE_WITH_KNOTS('',3,(#25979,#25980,#25981,#25982,#25983,
#25984,#25985,#25986,#25987,#25988,#25989,#25990,#25991,#25992,#25993,#25994,
#25995,#25996,#25997,#25998,#25999,#26000,#26001,#26002,#26003,#26004,#26005,
#26006,#26007,#26008,#26009,#26010,#26011,#26012,#26013,#26014,#26015,#26016,
#26017,#26018),.UNSPECIFIED.,.F.,.F.,(4,3,3,3,3,3,3,3,3,3,3,3,3,4),(7.40931287245371,
7.8879159605858,8.38091070812241,8.87390545565902,9.36690020319563,9.85989495073224,
10.3528896982689,10.8458844458055,11.3388791933421,11.8318739408787,12.3248686884153,
12.8178634359519,13.3108581834885,13.6924981796333),.UNSPECIFIED.);
#418=B_SPLINE_CURVE_WITH_KNOTS('',3,(#26023,#26024,#26025,#26026,#26027,
#26028,#26029,#26030,#26031,#26032,#26033,#26034,#26035,#26036,#26037,#26038,
#26039,#26040,#26041,#26042,#26043,#26044,#26045,#26046,#26047,#26048,#26049,
#26050,#26051,#26052,#26053,#26054,#26055,#26056,#26057,#26058,#26059,#26060,
#26061,#26062,#26063,#26064,#26065),.UNSPECIFIED.,.F.,.F.,(4,3,3,3,3,3,
3,3,3,3,3,3,3,3,4),(-22.9425468016483,-22.6777583866842,-22.1847636391475,
-21.6917688916109,-21.1987741440743,-20.7057793965377,-20.2127846490011,
-19.7197899014645,-19.2267951539279,-18.7338004063913,-18.2408056588546,
-17.747810911318,-17.2548161637814,-16.7618214162448,-16.6593614944687),
 .UNSPECIFIED.);
#419=B_SPLINE_CURVE_WITH_KNOTS('',3,(#26066,#26067,#26068,#26069,#26070,
#26071,#26072,#26073,#26074,#26075,#26076,#26077,#26078,#26079,#26080,#26081,
#26082,#26083,#26084,#26085,#26086,#26087,#26088,#26089,#26090,#26091,#26092,
#26093,#26094,#26095,#26096,#26097,#26098,#26099,#26100,#26101,#26102,#26103,
#26104,#26105,#26106,#26107,#26108),.UNSPECIFIED.,.F.,.F.,(4,3,3,3,3,3,
3,3,3,3,3,3,3,3,4),(13.6924981796333,13.8038529310251,14.2968476785617,
14.7898424260984,15.282837173635,15.7758319211716,16.2688266687082,16.7618214162448,
17.2548161637814,17.747810911318,18.2408056588546,18.7338004063913,19.2267951539279,
19.7197899014645,19.9756834868129),.UNSPECIFIED.);
#420=B_SPLINE_CURVE_WITH_KNOTS('',3,(#26113,#26114,#26115,#26116,#26117,
#26118,#26119,#26120,#26121,#26122,#26123,#26124,#26125,#26126,#26127,#26128,
#26129,#26130,#26131,#26132,#26133,#26134,#26135,#26136,#26137,#26138,#26139,
#26140,#26141,#26142,#26143,#26144,#26145,#26146,#26147,#26148,#26149,#26150,
#26151,#26152,#26153,#26154,#26155),.UNSPECIFIED.,.F.,.F.,(4,3,3,3,3,3,
3,3,3,3,3,3,3,3,4),(-29.2257321088278,-29.0866901046601,-28.5936953571235,
-28.1007006095869,-27.6077058620503,-27.1147111145137,-26.621716366977,
-26.1287216194404,-25.6357268719038,-25.1427321243672,-24.6497373768306,
-24.156742629294,-23.6637478817574,-23.1707531342208,-22.9425468016483),
 .UNSPECIFIED.);
#421=B_SPLINE_CURVE_WITH_KNOTS('',3,(#26156,#26157,#26158,#26159,#26160,
#26161,#26162,#26163,#26164,#26165,#26166,#26167,#26168,#26169,#26170,#26171,
#26172,#26173,#26174,#26175,#26176,#26177,#26178,#26179,#26180,#26181,#26182,
#26183,#26184,#26185,#26186,#26187,#26188,#26189,#26190,#26191,#26192,#26193,
#26194,#26195,#26196,#26197,#26198),.UNSPECIFIED.,.F.,.F.,(4,3,3,3,3,3,
3,3,3,3,3,3,3,3,4),(19.9756834868129,20.2127846490011,20.7057793965377,
21.1987741440743,21.6917688916109,22.1847636391475,22.6777583866842,23.1707531342208,
23.6637478817574,24.156742629294,24.6497373768306,25.1427321243672,25.6357268719038,
26.1287216194404,26.2588687939925),.UNSPECIFIED.);
#422=B_SPLINE_CURVE_WITH_KNOTS('',3,(#26203,#26204,#26205,#26206,#26207,
#26208,#26209,#26210,#26211,#26212,#26213,#26214,#26215,#26216,#26217,#26218,
#26219,#26220,#26221,#26222,#26223,#26224,#26225,#26226,#26227,#26228,#26229,
#26230,#26231,#26232,#26233,#26234,#26235,#26236,#26237,#26238,#26239,#26240,
#26241,#26242,#26243,#26244,#26245),.UNSPECIFIED.,.F.,.F.,(4,3,3,3,3,3,
3,3,3,3,3,3,3,3,4),(-35.5089174160074,-35.4956218226361,-35.0026270750994,
-34.5096323275628,-34.0166375800262,-33.5236428324896,-33.030648084953,
-32.5376533374164,-32.0446585898798,-31.5516638423432,-31.0586690948066,
-30.5656743472699,-30.0726795997333,-29.5796848521967,-29.2257321088278),
 .UNSPECIFIED.);
#423=B_SPLINE_CURVE_WITH_KNOTS('',3,(#26246,#26247,#26248,#26249,#26250,
#26251,#26252,#26253,#26254,#26255,#26256,#26257,#26258,#26259,#26260,#26261,
#26262,#26263,#26264,#26265,#26266,#26267,#26268,#26269,#26270,#26271,#26272,
#26273,#26274,#26275,#26276,#26277,#26278,#26279,#26280,#26281,#26282,#26283,
#26284,#26285,#26286,#26287,#26288),.UNSPECIFIED.,.F.,.F.,(4,3,3,3,3,3,
3,3,3,3,3,3,3,3,4),(26.2588687939925,26.621716366977,27.1147111145136,27.6077058620503,
28.1007006095869,28.5936953571235,29.0866901046601,29.5796848521967,30.0726795997333,
30.5656743472699,31.0586690948066,31.5516638423432,32.0446585898798,32.5376533374164,
32.5420541011721),.UNSPECIFIED.);
#424=B_SPLINE_CURVE_WITH_KNOTS('',3,(#26293,#26294,#26295,#26296,#26297,
#26298,#26299,#26300,#26301,#26302,#26303,#26304,#26305,#26306,#26307,#26308,
#26309,#26310,#26311,#26312,#26313,#26314,#26315,#26316,#26317,#26318,#26319,
#26320,#26321,#26322,#26323,#26324,#26325,#26326,#26327,#26328,#26329,#26330,
#26331,#26332),.UNSPECIFIED.,.F.,.F.,(4,3,3,3,3,3,3,3,3,3,3,3,3,4),(-41.792102723187,
-41.4115587930754,-40.9185640455388,-40.4255692980022,-39.9325745504656,
-39.439579802929,-38.9465850553923,-38.4535903078557,-37.9605955603191,
-37.4676008127825,-36.9746060652459,-36.4816113177093,-35.9886165701727,
-35.5089174160074),.UNSPECIFIED.);
#425=B_SPLINE_CURVE_WITH_KNOTS('',3,(#26333,#26334,#26335,#26336,#26337,
#26338,#26339,#26340,#26341,#26342,#26343,#26344,#26345,#26346,#26347,#26348,
#26349,#26350,#26351,#26352,#26353,#26354,#26355,#26356,#26357,#26358,#26359,
#26360,#26361,#26362,#26363,#26364,#26365,#26366,#26367,#26368,#26369,#26370,
#26371,#26372),.UNSPECIFIED.,.F.,.F.,(4,3,3,3,3,3,3,3,3,3,3,3,3,4),(32.5420541011721,
33.030648084953,33.5236428324896,34.0166375800262,34.5096323275628,35.0026270750995,
35.4956218226361,35.9886165701727,36.4816113177093,36.9746060652459,37.4676008127825,
37.9605955603191,38.4535903078557,38.8252394083517),.UNSPECIFIED.);
#426=B_SPLINE_CURVE_WITH_KNOTS('',3,(#26377,#26378,#26379,#26380,#26381,
#26382,#26383,#26384,#26385,#26386,#26387,#26388,#26389,#26390,#26391,#26392,
#26393,#26394,#26395,#26396,#26397,#26398,#26399,#26400,#26401,#26402,#26403,
#26404,#26405,#26406,#26407,#26408,#26409,#26410,#26411,#26412,#26413,#26414,
#26415,#26416,#26417,#26418,#26419),.UNSPECIFIED.,.F.,.F.,(4,3,3,3,3,3,
3,3,3,3,3,3,3,3,4),(-48.0752880303666,-47.8204905110514,-47.3274957635147,
-46.8345010159781,-46.3415062684415,-45.8485115209049,-45.3555167733683,
-44.8625220258317,-44.3695272782951,-43.8765325307585,-43.3835377832218,
-42.8905430356852,-42.3975482881486,-41.904553540612,-41.792102723187),
 .UNSPECIFIED.);
#427=B_SPLINE_CURVE_WITH_KNOTS('',3,(#26420,#26421,#26422,#26423,#26424,
#26425,#26426,#26427,#26428,#26429,#26430,#26431,#26432,#26433,#26434,#26435,
#26436,#26437,#26438,#26439,#26440,#26441,#26442,#26443,#26444,#26445,#26446,
#26447,#26448,#26449,#26450,#26451,#26452,#26453,#26454,#26455,#26456,#26457,
#26458,#26459,#26460,#26461,#26462),.UNSPECIFIED.,.F.,.F.,(4,3,3,3,3,3,
3,3,3,3,3,3,3,3,4),(38.8252394083517,38.9465850553923,39.439579802929,39.9325745504656,
40.4255692980022,40.9185640455388,41.4115587930754,41.904553540612,42.3975482881486,
42.8905430356852,43.3835377832219,43.8765325307585,44.3695272782951,44.8625220258317,
45.1084247155313),.UNSPECIFIED.);
#428=B_SPLINE_CURVE_WITH_KNOTS('',3,(#26467,#26468,#26469,#26470,#26471,
#26472,#26473,#26474,#26475,#26476,#26477,#26478,#26479,#26480,#26481,#26482,
#26483,#26484,#26485,#26486,#26487,#26488,#26489,#26490,#26491,#26492,#26493,
#26494,#26495,#26496,#26497,#26498,#26499,#26500,#26501,#26502,#26503,#26504,
#26505,#26506,#26507,#26508,#26509),.UNSPECIFIED.,.F.,.F.,(4,3,3,3,3,3,
3,3,3,3,3,3,3,3,4),(-54.3584733375463,-54.2294222290273,-53.7364274814907,
-53.2434327339541,-52.7504379864175,-52.2574432388809,-51.7644484913443,
-51.2714537438076,-50.778458996271,-50.2854642487344,-49.7924695011978,
-49.2994747536612,-48.8064800061246,-48.313485258588,-48.0752880303666),
 .UNSPECIFIED.);
#429=B_SPLINE_CURVE_WITH_KNOTS('',3,(#26510,#26511,#26512,#26513,#26514,
#26515,#26516,#26517,#26518,#26519,#26520,#26521,#26522,#26523,#26524,#26525,
#26526,#26527,#26528,#26529,#26530,#26531,#26532,#26533,#26534,#26535,#26536,
#26537,#26538,#26539,#26540,#26541,#26542,#26543,#26544,#26545,#26546,#26547,
#26548,#26549,#26550,#26551,#26552),.UNSPECIFIED.,.F.,.F.,(4,3,3,3,3,3,
3,3,3,3,3,3,3,3,4),(45.1084247155313,45.3555167733683,45.8485115209049,
46.3415062684415,46.8345010159781,47.3274957635147,47.8204905110514,48.313485258588,
48.8064800061246,49.2994747536612,49.7924695011978,50.2854642487344,50.778458996271,
51.2714537438076,51.3916100227108),.UNSPECIFIED.);
#430=B_SPLINE_CURVE_WITH_KNOTS('',3,(#26557,#26558,#26559,#26560,#26561,
#26562,#26563,#26564,#26565,#26566,#26567,#26568,#26569,#26570,#26571,#26572,
#26573,#26574,#26575,#26576,#26577,#26578,#26579,#26580,#26581,#26582,#26583,
#26584,#26585,#26586,#26587,#26588,#26589,#26590,#26591,#26592,#26593,#26594,
#26595,#26596,#26597,#26598,#26599),.UNSPECIFIED.,.F.,.F.,(4,3,3,3,3,3,
3,3,3,3,3,3,3,3,4),(-60.6416586447258,-60.6383539470033,-60.1453591994667,
-59.6523644519301,-59.1593697043935,-58.6663749568568,-58.1733802093202,
-57.6803854617836,-57.187390714247,-56.6943959667104,-56.2014012191738,
-55.7084064716372,-55.2154117241005,-54.7224169765639,-54.3584733375463),
 .UNSPECIFIED.);
#431=B_SPLINE_CURVE_WITH_KNOTS('',3,(#26600,#26601,#26602,#26603,#26604,
#26605,#26606,#26607,#26608,#26609,#26610,#26611,#26612,#26613,#26614,#26615,
#26616,#26617,#26618,#26619,#26620,#26621,#26622,#26623,#26624,#26625,#26626,
#26627,#26628,#26629,#26630,#26631,#26632,#26633,#26634,#26635,#26636,#26637,
#26638,#26639),.UNSPECIFIED.,.F.,.F.,(4,3,3,3,3,3,3,3,3,3,3,3,3,4),(51.3916100227108,
51.7644484913443,52.2574432388809,52.7504379864175,53.2434327339541,53.7364274814907,
54.2294222290273,54.7224169765639,55.2154117241005,55.7084064716371,56.2014012191738,
56.6943959667104,57.187390714247,57.6747953298905),.UNSPECIFIED.);
#432=B_SPLINE_CURVE_WITH_KNOTS('',3,(#26646,#26647,#26648,#26649,#26650,
#26651,#26652,#26653,#26654,#26655,#26656,#26657,#26658,#26659,#26660,#26661,
#26662,#26663,#26664,#26665,#26666,#26667,#26668,#26669,#26670,#26671,#26672,
#26673,#26674,#26675,#26676,#26677,#26678,#26679),.UNSPECIFIED.,.F.,.F.,
(4,3,3,3,3,3,3,3,3,3,3,4),(-66.061296169906,-65.5683014223694,-65.0753066748328,
-64.5823119272962,-64.0893171797595,-63.5963224322229,-63.1033276846864,
-62.6103329371497,-62.1173381896131,-61.6243434420765,-61.1313486945399,
-60.6416586447258),.UNSPECIFIED.);
#433=B_SPLINE_CURVE_WITH_KNOTS('',3,(#26680,#26681,#26682,#26683,#26684,
#26685,#26686,#26687,#26688,#26689,#26690,#26691,#26692,#26693,#26694,#26695,
#26696,#26697,#26698,#26699,#26700,#26701,#26702,#26703,#26704,#26705,#26706,
#26707,#26708,#26709,#26710,#26711,#26712,#26713,#26714,#26715,#26716,#26717,
#26718,#26719,#26720,#26721,#26722),.UNSPECIFIED.,.F.,.F.,(4,3,3,3,3,3,
3,3,3,3,3,3,3,3,4),(57.6747953298905,57.6803854617836,58.1733802093202,
58.6663749568568,59.1593697043934,59.65236445193,60.1453591994666,60.6383539470033,
61.1313486945399,61.6243434420765,62.1173381896131,62.6103329371497,63.1033276846863,
63.5963224322229,63.95798063707),.UNSPECIFIED.);
#434=B_SPLINE_CURVE_WITH_KNOTS('',3,(#26728,#26729,#26730,#26731,#26732,
#26733,#26734,#26735,#26736,#26737),.UNSPECIFIED.,.F.,.F.,(4,1,1,1,1,1,
1,4),(72.2566310325652,72.7463210823793,73.2393158299159,73.7323105774525,
74.2253053249892,74.7183000725258,75.2112948200624,75.5987427659515),
 .UNSPECIFIED.);
#435=B_SPLINE_CURVE_WITH_KNOTS('',3,(#26740,#26741,#26742,#26743,#26744,
#26745,#26746,#26747),.UNSPECIFIED.,.F.,.F.,(4,1,1,1,1,4),(72.2566310325652,
72.3879675752547,72.8809623227913,73.3739570703279,73.8669518178645,74.3599465654011),
 .UNSPECIFIED.);
#436=B_SPLINE_CURVE_WITH_KNOTS('',3,(#26752,#26753,#26754,#26755,#26756,
#26757,#26758,#26759,#26760,#26761,#26762,#26763,#26764,#26765,#26766,#26767,
#26768),.UNSPECIFIED.,.F.,.F.,(4,1,1,1,1,1,1,1,1,1,1,1,1,1,4),(65.9734457253857,
66.3373893644034,66.83038411194,67.3233788594766,67.8163736070132,68.3093683545498,
68.8023631020864,69.295357849623,69.7883525971596,70.2813473446963,70.7743420922329,
71.2673368397695,71.7603315873061,72.2533263348427,72.2566310325652),
 .UNSPECIFIED.);
#437=B_SPLINE_CURVE_WITH_KNOTS('',3,(#26769,#26770,#26771,#26772,#26773,
#26774,#26775,#26776,#26777,#26778,#26779,#26780,#26781,#26782,#26783,#26784,
#26785),.UNSPECIFIED.,.F.,.F.,(4,1,1,1,1,1,1,1,1,1,1,1,1,1,4),(65.9734457253857,
65.9790358572787,66.4720306048154,66.965025352352,67.4580200998886,67.9510148474252,
68.4440095949618,68.9370043424984,69.429999090035,69.9229938375716,70.4159885851083,
70.9089833326449,71.4019780801815,71.8949728277181,72.2566310325652),
 .UNSPECIFIED.);
#438=B_SPLINE_CURVE_WITH_KNOTS('',3,(#26790,#26791,#26792,#26793,#26794,
#26795,#26796,#26797,#26798,#26799,#26800,#26801,#26802,#26803,#26804,#26805,
#26806),.UNSPECIFIED.,.F.,.F.,(4,1,1,1,1,1,1,1,1,1,1,1,1,1,4),(59.690260418206,
59.9284576464274,60.421452393964,60.9144471415006,61.4074418890372,61.9004366365738,
62.3934313841105,62.8864261316471,63.3794208791837,63.8724156267203,64.3654103742569,
64.8584051217935,65.3513998693301,65.8443946168668,65.9734457253857),
 .UNSPECIFIED.);
#439=B_SPLINE_CURVE_WITH_KNOTS('',3,(#26807,#26808,#26809,#26810,#26811,
#26812,#26813,#26814,#26815,#26816,#26817,#26818,#26819,#26820,#26821,#26822),
 .UNSPECIFIED.,.F.,.F.,(4,1,1,1,1,1,1,1,1,1,1,1,1,4),(59.690260418206,60.0630988868394,
60.556093634376,61.0490883819126,61.5420831294492,62.0350778769859,62.5280726245225,
63.0210673720591,63.5140621195957,64.0070568671323,64.5000516146689,64.9930463622055,
65.4860411097421,65.9734457253857),.UNSPECIFIED.);
#440=B_SPLINE_CURVE_WITH_KNOTS('',3,(#26827,#26828,#26829,#26830,#26831,
#26832,#26833,#26834,#26835,#26836,#26837,#26838,#26839,#26840,#26841,#26842,
#26843),.UNSPECIFIED.,.F.,.F.,(4,1,1,1,1,1,1,1,1,1,1,1,1,1,4),(53.4070751110265,
53.5195259284514,54.0125206759881,54.5055154235247,54.9985101710613,55.4915049185979,
55.9844996661345,56.4774944136711,56.9704891612077,57.4634839087443,57.956478656281,
58.4494734038176,58.9424681513542,59.4354628988908,59.690260418206),
 .UNSPECIFIED.);
#441=B_SPLINE_CURVE_WITH_KNOTS('',3,(#26844,#26845,#26846,#26847,#26848,
#26849,#26850,#26851,#26852,#26853,#26854,#26855,#26856,#26857,#26858,#26859,
#26860),.UNSPECIFIED.,.F.,.F.,(4,1,1,1,1,1,1,1,1,1,1,1,1,1,4),(53.4070751110265,
53.6541671688635,54.1471619164001,54.6401566639367,55.1331514114733,55.6261461590099,
56.1191409065465,56.6121356540831,57.1051304016197,57.5981251491563,58.091119896693,
58.5841146442296,59.0771093917662,59.5701041393028,59.690260418206),
 .UNSPECIFIED.);
#442=B_SPLINE_CURVE_WITH_KNOTS('',3,(#26865,#26866,#26867,#26868,#26869,
#26870,#26871,#26872,#26873,#26874,#26875,#26876,#26877,#26878,#26879,#26880),
 .UNSPECIFIED.,.F.,.F.,(4,1,1,1,1,1,1,1,1,1,1,1,1,4),(47.1238898038469,
47.6035889580121,48.0965837055487,48.5895784530853,49.0825732006219,49.5755679481586,
50.0685626956952,50.5615574432318,51.0545521907684,51.547546938305,52.0405416858416,
52.5335364333782,53.0265311809148,53.4070751110265),.UNSPECIFIED.);
#443=B_SPLINE_CURVE_WITH_KNOTS('',3,(#26881,#26882,#26883,#26884,#26885,
#26886,#26887,#26888,#26889,#26890,#26891,#26892,#26893,#26894,#26895,#26896,
#26897),.UNSPECIFIED.,.F.,.F.,(4,1,1,1,1,1,1,1,1,1,1,1,1,1,4),(47.1238898038469,
47.2452354508875,47.7382301984241,48.2312249459607,48.7242196934973,49.2172144410339,
49.7102091885705,50.2032039361072,50.6961986836438,51.1891934311804,51.682188178717,
52.1751829262536,52.6681776737902,53.1611724213268,53.4070751110265),
 .UNSPECIFIED.);
#444=B_SPLINE_CURVE_WITH_KNOTS('',3,(#26902,#26903,#26904,#26905,#26906,
#26907,#26908,#26909,#26910,#26911,#26912,#26913,#26914,#26915,#26916,#26917,
#26918),.UNSPECIFIED.,.F.,.F.,(4,1,1,1,1,1,1,1,1,1,1,1,1,1,4),(40.8407044966673,
41.1946572400362,41.6876519875728,42.1806467351094,42.673641482646,43.1666362301826,
43.6596309777192,44.1526257252558,44.6456204727924,45.138615220329,45.6316099678657,
46.1246047154023,46.6175994629389,47.1105942104755,47.1238898038469),
 .UNSPECIFIED.);
#445=B_SPLINE_CURVE_WITH_KNOTS('',3,(#26919,#26920,#26921,#26922,#26923,
#26924,#26925,#26926,#26927,#26928,#26929,#26930,#26931,#26932,#26933,#26934),
 .UNSPECIFIED.,.F.,.F.,(4,1,1,1,1,1,1,1,1,1,1,1,1,4),(40.8407044966673,
41.3292984804481,41.8222932279848,42.3152879755214,42.808282723058,43.3012774705946,
43.7942722181312,44.2872669656678,44.7802617132044,45.273256460741,45.7662512082777,
46.2592459558143,46.7522407033509,47.1238898038469),.UNSPECIFIED.);
#446=B_SPLINE_CURVE_WITH_KNOTS('',3,(#26939,#26940,#26941,#26942,#26943,
#26944,#26945,#26946,#26947,#26948,#26949,#26950,#26951,#26952,#26953,#26954,
#26955),.UNSPECIFIED.,.F.,.F.,(4,1,1,1,1,1,1,1,1,1,1,1,1,1,4),(34.5575191894877,
34.7857255220602,35.2787202695968,35.7717150171334,36.26470976467,36.7577045122066,
37.2506992597433,37.7436940072799,38.2366887548165,38.7296835023531,39.2226782498897,
39.7156729974263,40.2086677449629,40.7016624924995,40.8407044966673),
 .UNSPECIFIED.);
#447=B_SPLINE_CURVE_WITH_KNOTS('',3,(#26956,#26957,#26958,#26959,#26960,
#26961,#26962,#26963,#26964,#26965,#26966,#26967,#26968,#26969,#26970,#26971,
#26972),.UNSPECIFIED.,.F.,.F.,(4,1,1,1,1,1,1,1,1,1,1,1,1,1,4),(34.5575191894877,
34.9203667624722,35.4133615100088,35.9063562575454,36.399351005082,36.8923457526186,
37.3853405001553,37.8783352476919,38.3713299952285,38.8643247427651,39.3573194903017,
39.8503142378383,40.3433089853749,40.8363037329115,40.8407044966673),
 .UNSPECIFIED.);
#448=B_SPLINE_CURVE_WITH_KNOTS('',3,(#26977,#26978,#26979,#26980,#26981,
#26982,#26983,#26984,#26985,#26986,#26987,#26988,#26989,#26990,#26991,#26992,
#26993),.UNSPECIFIED.,.F.,.F.,(4,1,1,1,1,1,1,1,1,1,1,1,1,1,4),(28.2743338823081,
28.3767938040842,28.8697885516209,29.3627832991575,29.8557780466941,30.3487727942307,
30.8417675417673,31.3347622893039,31.8277570368405,32.3207517843771,32.8137465319137,
33.3067412794504,33.799736026987,34.2927307745236,34.5575191894877),
 .UNSPECIFIED.);
#449=B_SPLINE_CURVE_WITH_KNOTS('',3,(#26994,#26995,#26996,#26997,#26998,
#26999,#27000,#27001,#27002,#27003,#27004,#27005,#27006,#27007,#27008,#27009,
#27010),.UNSPECIFIED.,.F.,.F.,(4,1,1,1,1,1,1,1,1,1,1,1,1,1,4),(28.2743338823081,
28.5114350444962,29.0044297920328,29.4974245395695,29.9904192871061,30.4834140346427,
30.9764087821793,31.4694035297159,31.9623982772525,32.4553930247891,32.9483877723257,
33.4413825198624,33.934377267399,34.4273720149356,34.5575191894877),
 .UNSPECIFIED.);
#450=B_SPLINE_CURVE_WITH_KNOTS('',3,(#27015,#27016,#27017,#27018,#27019,
#27020,#27021,#27022,#27023,#27024,#27025,#27026,#27027,#27028,#27029,#27030),
 .UNSPECIFIED.,.F.,.F.,(4,1,1,1,1,1,1,1,1,1,1,1,1,4),(21.9911485751285,
22.4608568336449,22.9538515811815,23.4468463287181,23.9398410762547,24.4328358237913,
24.925830571328,25.4188253188646,25.9118200664012,26.4048148139378,26.8978095614744,
27.390804309011,27.8837990565476,28.2743338823081),.UNSPECIFIED.);
#451=B_SPLINE_CURVE_WITH_KNOTS('',3,(#27031,#27032,#27033,#27034,#27035,
#27036,#27037,#27038,#27039,#27040,#27041,#27042,#27043,#27044,#27045,#27046,
#27047),.UNSPECIFIED.,.F.,.F.,(4,1,1,1,1,1,1,1,1,1,1,1,1,1,4),(21.9911485751285,
22.1025033265203,22.5954980740569,23.0884928215935,23.5814875691301,24.0744823166667,
24.5674770642033,25.06047181174,25.5534665592766,26.0464613068132,26.5394560543498,
27.0324508018864,27.525445549423,28.0184402969596,28.2743338823081),
 .UNSPECIFIED.);
#452=B_SPLINE_CURVE_WITH_KNOTS('',3,(#27052,#27053,#27054,#27055,#27056,
#27057,#27058,#27059,#27060,#27061,#27062,#27063,#27064,#27065,#27066,#27067,
#27068),.UNSPECIFIED.,.F.,.F.,(4,1,1,1,1,1,1,1,1,1,1,1,1,1,4),(15.7079632679489,
16.0519251156689,16.5449198632055,17.0379146107422,17.5309093582788,18.0239041058154,
18.516898853352,19.0098936008886,19.5028883484252,19.9958830959618,20.4888778434984,
20.9818725910351,21.4748673385717,21.9678620861083,21.9911485751285),
 .UNSPECIFIED.);
#453=B_SPLINE_CURVE_WITH_KNOTS('',3,(#27069,#27070,#27071,#27072,#27073,
#27074,#27075,#27076,#27077,#27078,#27079,#27080,#27081,#27082,#27083,#27084),
 .UNSPECIFIED.,.F.,.F.,(4,1,1,1,1,1,1,1,1,1,1,1,1,4),(15.7079632679489,
16.1865663560809,16.6795611036176,17.1725558511542,17.6655505986908,18.1585453462274,
18.651540093764,19.1445348413006,19.6375295888372,20.1305243363738,20.6235190839104,
21.1165138314471,21.6095085789837,21.9911485751285),.UNSPECIFIED.);
#454=B_SPLINE_CURVE_WITH_KNOTS('',3,(#27123,#27124,#27125,#27126,#27127,
#27128,#27129,#27130,#27131,#27132,#27133,#27134,#27135,#27136,#27137,#27138,
#27139,#27140,#27141,#27142,#27143,#27144,#27145,#27146,#27147,#27148,#27149,
#27150,#27151,#27152,#27153,#27154,#27155,#27156,#27157,#27158,#27159,#27160,
#27161,#27162,#27163,#27164,#27165,#27166,#27167,#27168,#27169,#27170,#27171,
#27172,#27173,#27174,#27175,#27176,#27177,#27178,#27179,#27180,#27181,#27182,
#27183,#27184,#27185,#27186,#27187,#27188,#27189,#27190,#27191,#27192,#27193,
#27194,#27195,#27196,#27197,#27198,#27199,#27200,#27201,#27202,#27203,#27204,
#27205,#27206,#27207,#27208,#27209,#27210,#27211,#27212,#27213,#27214,#27215,
#27216,#27217,#27218,#27219,#27220,#27221,#27222,#27223,#27224,#27225,#27226,
#27227,#27228,#27229,#27230,#27231,#27232,#27233,#27234,#27235,#27236,#27237,
#27238,#27239,#27240,#27241,#27242,#27243,#27244,#27245,#27246,#27247,#27248,
#27249,#27250,#27251,#27252,#27253,#27254,#27255,#27256,#27257,#27258,#27259,
#27260,#27261),.UNSPECIFIED.,.F.,.F.,(4,3,3,3,3,3,3,3,3,3,3,3,3,3,3,3,3,
3,3,3,3,3,3,3,3,3,3,3,3,3,3,3,3,3,3,3,3,3,3,3,3,3,3,3,3,3,4),(-3.33140537618017,
-3.22326787461695,-3.15817079917648,-3.049853301467,-2.96298085620029,-2.9249741613961,
-2.90862147149683,-2.89605517458874,-2.78842365923039,-2.68003617925612,
-2.57290868632918,-2.51839994958021,-2.48953284996429,-2.47285249228237,
-2.36566522894994,-2.35487373933332,-2.24815410350468,-2.14082940646807,
-2.03352875005321,-1.92687843487524,-1.88101360087459,-1.8578477981616,
-1.84418934496722,-1.73779564851565,-1.63148467619083,-1.55995976287002,
-1.45341767338637,-1.34699981245266,-1.27548160451177,-1.24419238853763,
-1.23174198713026,-1.22128582434211,-1.1161023209359,-1.01033276551643,
-0.904839743637061,-0.80044976709345,-0.774854148925534,-0.677997380309842,
-0.635622544040477,-0.618977051328633,-0.603748925809969,-0.49973180882737,
-0.394912479224905,-0.290040790477003,-0.18575703861591,-0.0831547939216665,
0.),.UNSPECIFIED.);
#455=B_SPLINE_CURVE_WITH_KNOTS('',3,(#27264,#27265,#27266,#27267,#27268,
#27269,#27270,#27271,#27272,#27273,#27274,#27275,#27276,#27277,#27278,#27279,
#27280,#27281,#27282,#27283,#27284,#27285,#27286,#27287,#27288,#27289,#27290,
#27291,#27292,#27293,#27294,#27295,#27296,#27297,#27298,#27299,#27300,#27301,
#27302,#27303,#27304,#27305,#27306,#27307,#27308,#27309,#27310,#27311,#27312,
#27313,#27314,#27315,#27316,#27317,#27318,#27319,#27320,#27321,#27322,#27323,
#27324,#27325,#27326,#27327,#27328,#27329,#27330,#27331,#27332,#27333,#27334,
#27335,#27336,#27337,#27338,#27339,#27340,#27341,#27342,#27343,#27344,#27345,
#27346,#27347,#27348,#27349,#27350,#27351,#27352,#27353,#27354,#27355,#27356,
#27357,#27358,#27359,#27360,#27361,#27362,#27363,#27364,#27365,#27366,#27367,
#27368,#27369,#27370,#27371,#27372,#27373,#27374,#27375,#27376,#27377,#27378,
#27379,#27380,#27381,#27382,#27383,#27384,#27385,#27386,#27387,#27388,#27389,
#27390,#27391,#27392,#27393,#27394,#27395,#27396,#27397,#27398,#27399,#27400,
#27401,#27402),.UNSPECIFIED.,.F.,.F.,(4,3,3,3,3,3,3,3,3,3,3,3,3,3,3,3,3,
3,3,3,3,3,3,3,3,3,3,3,3,3,3,3,3,3,3,3,3,3,3,3,3,3,3,3,3,3,4),(-3.3351521949513,
-3.23035412220627,-3.17020330978756,-3.06579909218576,-2.98176387938634,
-2.9449984737866,-2.92915657616349,-2.91720620520155,-2.81251162890031,
-2.7071228788428,-2.60200290909517,-2.54988152926899,-2.52416540839213,
-2.50878246245602,-2.40282819474695,-2.39351738979045,-2.28862560733202,
-2.18281471664314,-2.07663992389392,-1.97072839078126,-1.92506933135162,
-1.90124417079794,-1.8893117349777,-1.78281482245468,-1.67586957667813,
-1.60545591534413,-1.49883052806521,-1.39193067774417,-1.31887193544069,
-1.28690873568292,-1.27388989384833,-1.26361386894611,-1.15708585888843,
-1.04940938788384,-0.941663866948425,-0.834628763436338,-0.807460739316361,
-0.706528146901816,-0.662370137720452,-0.64258228962385,-0.631550073319128,
-0.524780997969994,-0.416884173936585,-0.308312901558949,-0.200010753330189,
-0.0930669769078746,0.),.UNSPECIFIED.);
#456=B_SPLINE_CURVE_WITH_KNOTS('',3,(#27409,#27410,#27411,#27412,#27413,
#27414),.UNSPECIFIED.,.F.,.F.,(4,2,4),(2.90070768857401,3.00706665159486,
3.1886726077324),.UNSPECIFIED.);
#457=B_SPLINE_CURVE_WITH_KNOTS('',3,(#27417,#27418,#27419,#27420,#27421,
#27422),.UNSPECIFIED.,.F.,.F.,(4,2,4),(3.1886726077324,3.37027856386994,
3.4766375268908),.UNSPECIFIED.);
#458=B_SPLINE_CURVE_WITH_KNOTS('',3,(#27435,#27436,#27437,#27438,#27439,
#27440,#27441,#27442,#27443,#27444,#27445,#27446,#27447,#27448,#27449,#27450,
#27451,#27452,#27453,#27454,#27455,#27456,#27457,#27458,#27459,#27460,#27461,
#27462,#27463,#27464,#27465,#27466,#27467,#27468,#27469,#27470,#27471,#27472,
#27473,#27474,#27475,#27476,#27477,#27478,#27479,#27480,#27481,#27482,#27483,
#27484,#27485,#27486,#27487,#27488,#27489,#27490,#27491,#27492,#27493,#27494,
#27495,#27496,#27497,#27498,#27499,#27500,#27501,#27502,#27503,#27504,#27505,
#27506,#27507,#27508,#27509,#27510,#27511,#27512,#27513,#27514,#27515,#27516,
#27517,#27518,#27519,#27520,#27521,#27522,#27523,#27524,#27525,#27526,#27527,
#27528,#27529,#27530,#27531,#27532,#27533,#27534,#27535,#27536,#27537,#27538,
#27539,#27540,#27541,#27542,#27543,#27544,#27545,#27546,#27547,#27548,#27549,
#27550,#27551,#27552,#27553,#27554,#27555,#27556,#27557,#27558,#27559,#27560,
#27561,#27562,#27563,#27564,#27565,#27566,#27567,#27568,#27569,#27570,#27571,
#27572,#27573),.UNSPECIFIED.,.F.,.F.,(4,3,3,3,3,3,3,3,3,3,3,3,3,3,3,3,3,
3,3,3,3,3,3,3,3,3,3,3,3,3,3,3,3,3,3,3,3,3,3,3,3,3,3,3,3,3,4),(-3.3351521949513,
-3.23035412240041,-3.17020330978753,-3.06579909250646,-2.98176387966696,
-2.94499847404967,-2.92915657746123,-2.9172062091037,-2.81251163327298,
-2.70712288308388,-2.60200291309312,-2.54988153226745,-2.52416540972209,
-2.50878246249469,-2.40282819474078,-2.39351738979045,-2.28862560698356,
-2.18281471621706,-2.07663992322332,-1.97072838921362,-1.92506932997993,
-1.90124416858194,-1.88931173446478,-1.78281482187671,-1.67586957561123,
-1.60545591534413,-1.49883052685415,-1.39193067699312,-1.31887193478353,
-1.28690873506683,-1.27388989154254,-1.26361386703925,-1.15708585497168,
-1.04940938370439,-0.941663864345138,-0.834628765543497,-0.807460739316348,
-0.706528146901805,-0.662370137720442,-0.642582289491659,-0.631550074280081,
-0.524781005409625,-0.41688418584941,-0.308312912995514,-0.200010761086136,
-0.0930669761911965,0.),.UNSPECIFIED.);
#459=B_SPLINE_CURVE_WITH_KNOTS('',3,(#27576,#27577,#27578,#27579,#27580,
#27581,#27582,#27583,#27584,#27585,#27586,#27587,#27588,#27589,#27590,#27591,
#27592,#27593,#27594,#27595,#27596,#27597,#27598,#27599,#27600,#27601,#27602,
#27603,#27604,#27605,#27606,#27607,#27608,#27609,#27610,#27611,#27612,#27613,
#27614,#27615,#27616,#27617,#27618,#27619,#27620,#27621,#27622,#27623,#27624,
#27625,#27626,#27627,#27628,#27629,#27630,#27631,#27632,#27633,#27634,#27635,
#27636,#27637,#27638,#27639,#27640,#27641,#27642,#27643,#27644,#27645,#27646,
#27647,#27648,#27649,#27650,#27651,#27652,#27653,#27654,#27655,#27656,#27657,
#27658,#27659,#27660,#27661,#27662,#27663,#27664,#27665,#27666,#27667,#27668,
#27669,#27670,#27671,#27672,#27673,#27674,#27675,#27676,#27677,#27678,#27679,
#27680,#27681,#27682,#27683,#27684,#27685,#27686,#27687,#27688,#27689,#27690,
#27691,#27692,#27693,#27694,#27695,#27696,#27697,#27698,#27699,#27700,#27701,
#27702,#27703,#27704,#27705,#27706,#27707,#27708,#27709,#27710,#27711,#27712,
#27713,#27714),.UNSPECIFIED.,.F.,.F.,(4,3,3,3,3,3,3,3,3,3,3,3,3,3,3,3,3,
3,3,3,3,3,3,3,3,3,3,3,3,3,3,3,3,3,3,3,3,3,3,3,3,3,3,3,3,3,4),(-3.33140537617985,
-3.22326787425814,-3.15817079917634,-3.0498533014283,-2.96298085616642,
-2.92497416136434,-2.90862147116675,-2.8960551743525,-2.78842365887399,
-2.6800361789888,-2.5729086860616,-2.51839994937951,-2.48953284992468,-2.47285249229225,
-2.36566522904863,-2.35487373933324,-2.24815410347614,-2.14082940659152,
-2.03352875103554,-1.92687843770874,-1.88101360335389,-1.85784780192153,
-1.84418934498894,-1.73779564875492,-1.63148467770906,-1.55995976286992,
-1.45341767352125,-1.34699981034086,-1.27548160266394,-1.24419238680529,
-1.23174197960383,-1.22128582242241,-1.11610232056299,-1.01033276385257,
-0.904839738472552,-0.800449755260466,-0.774854148925471,-0.677997380309787,
-0.635622544040425,-0.618977051412567,-0.603748926550004,-0.49973180431923,
-0.394912472330862,-0.290040786684448,-0.18575704090222,-0.0831548060731709,
0.),.UNSPECIFIED.);
#460=B_SPLINE_CURVE_WITH_KNOTS('',3,(#28263,#28264,#28265,#28266),
 .UNSPECIFIED.,.F.,.F.,(4,4),(63.95798063707,63.9837703781121),
 .UNSPECIFIED.);
#461=B_SPLINE_CURVE_WITH_KNOTS('',3,(#28267,#28268,#28269,#28270,#28271,
#28272,#28273,#28274,#28275,#28276,#28277,#28278,#28279,#28280,#28281),
 .UNSPECIFIED.,.F.,.F.,(4,1,1,1,1,1,1,1,1,1,1,1,4),(10.376176187289,10.7636241331782,
11.2566188807148,11.7496136282514,12.242608375788,12.7356031233247,13.2285978708613,
13.7215926183979,14.2145873659345,14.7075821134711,15.2005768610077,15.6935716085443,
15.7079632679489),.UNSPECIFIED.);
#462=B_SPLINE_CURVE_WITH_KNOTS('',3,(#28283,#28284,#28285,#28286,#28287,
#28288,#28289,#28290,#28291,#28292,#28293,#28294),.UNSPECIFIED.,.F.,.F.,
(4,1,1,1,1,1,1,1,1,4),(11.6149723878394,12.107967135376,12.6009618829127,
13.0939566304493,13.5869513779859,14.0799461255225,14.5729408730591,15.0659356205957,
15.5589303681323,15.7079632679489),.UNSPECIFIED.);
#463=B_SPLINE_CURVE_WITH_KNOTS('',3,(#29658,#29659,#29660,#29661,#29662,
#29663,#29664,#29665,#29666,#29667,#29668,#29669,#29670,#29671,#29672,#29673,
#29674,#29675,#29676,#29677,#29678,#29679,#29680,#29681,#29682,#29683,#29684,
#29685,#29686,#29687,#29688,#29689,#29690,#29691,#29692,#29693,#29694,#29695,
#29696,#29697,#29698,#29699,#29700,#29701,#29702,#29703,#29704,#29705,#29706,
#29707,#29708,#29709,#29710,#29711,#29712,#29713,#29714,#29715,#29716,#29717,
#29718,#29719,#29720,#29721,#29722,#29723,#29724,#29725,#29726,#29727,#29728,
#29729,#29730,#29731,#29732,#29733,#29734,#29735,#29736,#29737,#29738,#29739,
#29740,#29741,#29742,#29743,#29744,#29745,#29746,#29747,#29748,#29749,#29750,
#29751,#29752,#29753,#29754,#29755,#29756,#29757,#29758,#29759,#29760,#29761,
#29762,#29763,#29764,#29765,#29766,#29767,#29768,#29769,#29770,#29771,#29772,
#29773,#29774,#29775,#29776,#29777,#29778,#29779,#29780,#29781,#29782,#29783,
#29784,#29785,#29786,#29787,#29788,#29789,#29790,#29791,#29792,#29793),
 .UNSPECIFIED.,.F.,.F.,(4,3,3,3,3,3,3,3,3,3,3,3,3,3,3,3,3,3,3,3,3,3,3,3,
3,3,3,3,3,3,3,3,3,3,3,3,3,3,3,3,3,3,3,3,3,4),(-4.26859401472304,-4.13873007688789,
-4.08850162055165,-3.95858584619281,-3.82847709951256,-3.73149748136453,
-3.71631594412289,-3.58696529636488,-3.45338401085574,-3.32450556188697,
-3.19666996642904,-3.18303474098074,-3.05264015432834,-2.92417890259064,
-2.79512825168043,-2.6658735005123,-2.53709505709189,-2.4090588279256,-2.39050563042798,
-2.3791326398393,-2.36740010056182,-2.23913691627976,-2.11091291541336,
-2.0249501404267,-1.89655785726426,-1.76815488394767,-1.67303375966788,
-1.58980277592306,-1.57904949215431,-1.45212314108153,-1.32439228312005,
-1.19687411471462,-1.07054011091882,-1.00718588970934,-0.881287653495677,
-0.826207175152197,-0.798981472708049,-0.78720874403541,-0.775317236286388,
-0.649547843460037,-0.522822362146257,-0.392116771609693,-0.26578478676463,
-0.140456274469436,-0.0170309231504542,0.),.UNSPECIFIED.);
#464=B_SPLINE_CURVE_WITH_KNOTS('',3,(#29794,#29795,#29796,#29797,#29798,
#29799,#29800,#29801,#29802,#29803,#29804,#29805,#29806,#29807,#29808,#29809),
 .UNSPECIFIED.,.F.,.F.,(4,3,3,3,3,4),(95.373907172968,95.5887530958692,
96.0866111849102,96.5844692739512,97.0823273629921,97.4940920164032),
 .UNSPECIFIED.);
#465=B_SPLINE_CURVE_WITH_KNOTS('',3,(#29811,#29812,#29813,#29814,#29815,
#29816,#29817,#29818,#29819,#29820,#29821,#29822,#29823,#29824,#29825,#29826,
#29827,#29828,#29829,#29830,#29831,#29832,#29833,#29834,#29835,#29836,#29837,
#29838,#29839,#29840,#29841,#29842,#29843,#29844,#29845,#29846,#29847,#29848,
#29849,#29850,#29851,#29852,#29853,#29854,#29855,#29856,#29857,#29858,#29859,
#29860,#29861,#29862,#29863,#29864,#29865,#29866,#29867,#29868,#29869,#29870,
#29871,#29872,#29873,#29874,#29875,#29876,#29877,#29878,#29879,#29880,#29881,
#29882,#29883,#29884,#29885,#29886,#29887,#29888,#29889,#29890,#29891,#29892,
#29893,#29894,#29895,#29896,#29897,#29898,#29899,#29900,#29901,#29902,#29903,
#29904,#29905,#29906,#29907,#29908,#29909,#29910,#29911,#29912,#29913,#29914,
#29915,#29916,#29917,#29918,#29919,#29920,#29921,#29922,#29923,#29924,#29925,
#29926,#29927,#29928,#29929,#29930,#29931,#29932,#29933,#29934,#29935,#29936,
#29937,#29938,#29939,#29940),.UNSPECIFIED.,.F.,.F.,(4,3,3,3,3,3,3,3,3,3,
3,3,3,3,3,3,3,3,3,3,3,3,3,3,3,3,3,3,3,3,3,3,3,3,3,3,3,3,3,3,3,3,3,4),(-4.27233968854161,
-4.14561602726014,-4.09907448469013,-3.97290709741126,-3.84621089191813,
-3.749773654366,-3.73627839431146,-3.60966162132612,-3.47994220953063,-3.35296282839602,
-3.22187340127008,-3.20970027001722,-3.09078397414414,-2.96324940449412,
-2.83568998921265,-2.70759606171859,-2.57963130546553,-2.45235033333514,
-2.43126259133011,-2.41607773241749,-2.28771734257599,-2.15890271920814,
-2.07050741694398,-1.94169654380679,-1.81290382296933,-1.71629339907897,
-1.63175927817491,-1.62010485283798,-1.49191166190089,-1.36241267866765,
-1.23282152109643,-1.10403428197821,-1.04002043184644,-0.910017877865636,
-0.853141760499034,-0.824352398485974,-0.813502334414714,-0.685266483128497,
-0.555745255190819,-0.425490911420356,-0.295356067993986,-0.165943780746531,
-0.0382708826685432,0.),.UNSPECIFIED.);
#466=B_SPLINE_CURVE_WITH_KNOTS('',3,(#29941,#29942,#29943,#29944,#29945,
#29946,#29947,#29948,#29949,#29950,#29951,#29952,#29953,#29954),
 .UNSPECIFIED.,.F.,.F.,(4,1,1,1,1,1,1,1,1,1,1,4),(10.376176187289,10.7879408407,
11.285798929741,11.783657018782,12.281515107823,12.779373196864,13.277231285905,
13.7750893749459,14.2729474639869,14.7708055530279,15.2686636420689,15.7079632679489),
 .UNSPECIFIED.);
#467=B_SPLINE_CURVE_WITH_KNOTS('',3,(#29960,#29961,#29962,#29963,#29964,
#29965,#29966,#29967,#29968,#29969,#29970,#29971,#29972,#29973,#29974,#29975,
#29976,#29977,#29978,#29979,#29980,#29981,#29982,#29983,#29984,#29985,#29986,
#29987,#29988,#29989,#29990,#29991,#29992,#29993,#29994,#29995,#29996,#29997,
#29998,#29999,#30000,#30001,#30002,#30003,#30004,#30005,#30006,#30007,#30008,
#30009,#30010,#30011,#30012,#30013,#30014,#30015,#30016,#30017,#30018,#30019,
#30020,#30021,#30022,#30023,#30024,#30025,#30026,#30027,#30028,#30029,#30030,
#30031,#30032,#30033,#30034,#30035,#30036,#30037,#30038,#30039,#30040,#30041,
#30042,#30043,#30044,#30045,#30046,#30047,#30048,#30049,#30050,#30051,#30052,
#30053,#30054,#30055,#30056,#30057,#30058,#30059,#30060,#30061,#30062,#30063,
#30064,#30065,#30066,#30067,#30068,#30069,#30070,#30071,#30072,#30073,#30074,
#30075,#30076,#30077,#30078,#30079,#30080,#30081,#30082,#30083,#30084,#30085,
#30086,#30087,#30088,#30089,#30090,#30091,#30092,#30093,#30094,#30095),
 .UNSPECIFIED.,.F.,.F.,(4,3,3,3,3,3,3,3,3,3,3,3,3,3,3,3,3,3,3,3,3,3,3,3,
3,3,3,3,3,3,3,3,3,3,3,3,3,3,3,3,3,3,3,3,3,4),(-4.26859401472303,-4.13873007862848,
-4.08850162055171,-3.95858584686358,-3.82847709974972,-3.73149748157205,
-3.71631594239557,-3.58696529527702,-3.45338401003986,-3.32450556087226,
-3.19666996624169,-3.18303474029221,-3.05264015432835,-2.92417890259064,
-2.7951282517208,-2.66587349878086,-2.53709505009457,-2.4090588226776,-2.39050561977311,
-2.37913262630794,-2.36740009695194,-2.23913691213895,-2.11091290702005,
-2.02495014042667,-1.89655785461699,-1.76815488608368,-1.67303376153689,
-1.58980277755845,-1.57904949311201,-1.4521231353151,-1.32439227972488,
-1.19687412089341,-1.07054013824695,-1.00718588970937,-0.881287653495698,
-0.826207175152217,-0.798981472541323,-0.78720874864497,-0.775317237411105,
-0.64954786276476,-0.522822391081097,-0.392116793310822,-0.265784790792495,
-0.140456252484584,-0.0170308663221606,0.),.UNSPECIFIED.);
#468=B_SPLINE_CURVE_WITH_KNOTS('',3,(#30098,#30099,#30100,#30101,#30102,
#30103,#30104,#30105,#30106,#30107,#30108,#30109),.UNSPECIFIED.,.F.,.F.,
(4,1,1,1,1,1,1,1,1,4),(11.6149723878395,12.1128304768804,12.6106885659214,
13.1085466549624,13.6064047440034,14.1042628330444,14.6021209220854,15.0999790111264,
15.5978371001673,15.7079632679489),.UNSPECIFIED.);
#469=B_SPLINE_CURVE_WITH_KNOTS('',3,(#30923,#30924,#30925,#30926,#30927,
#30928,#30929,#30930,#30931,#30932,#30933,#30934,#30935,#30936,#30937,#30938,
#30939,#30940,#30941,#30942,#30943,#30944,#30945,#30946,#30947,#30948,#30949,
#30950,#30951,#30952,#30953,#30954,#30955,#30956,#30957,#30958,#30959,#30960,
#30961,#30962,#30963,#30964,#30965,#30966,#30967,#30968,#30969,#30970,#30971,
#30972,#30973,#30974,#30975,#30976,#30977,#30978,#30979,#30980,#30981,#30982,
#30983,#30984,#30985,#30986,#30987,#30988,#30989,#30990,#30991,#30992,#30993,
#30994,#30995,#30996,#30997,#30998,#30999,#31000,#31001,#31002,#31003,#31004,
#31005,#31006,#31007,#31008,#31009,#31010,#31011,#31012,#31013,#31014,#31015,
#31016,#31017,#31018,#31019,#31020,#31021,#31022,#31023,#31024,#31025,#31026,
#31027,#31028,#31029,#31030,#31031,#31032,#31033,#31034,#31035,#31036,#31037,
#31038,#31039,#31040,#31041,#31042,#31043,#31044,#31045,#31046,#31047,#31048,
#31049,#31050,#31051,#31052),.UNSPECIFIED.,.F.,.F.,(4,3,3,3,3,3,3,3,3,3,
3,3,3,3,3,3,3,3,3,3,3,3,3,3,3,3,3,3,3,3,3,3,3,3,3,3,3,3,3,3,3,3,3,4),(-4.27233968854153,
-4.14561602839147,-4.09907448469005,-3.97290709931656,-3.84621089389475,
-3.74977366118721,-3.73627840644343,-3.60966163550516,-3.47994222016488,
-3.35296283800287,-3.22187340607345,-3.2097002822526,-3.09078397414404,
-2.96324940449404,-2.83568998898437,-2.70759606104771,-2.57963130228954,
-2.45235033095315,-2.43126258472487,-2.41607773095023,-2.28771734093045,
-2.15890271577605,-2.07050741694398,-1.94169654380679,-1.81290382315168,
-1.71629339923853,-1.63175927831451,-1.62010485805667,-1.49191165955653,
-1.36241267466591,-1.2328215214719,-1.10403429784844,-1.04002043184644,
-0.910017877865632,-0.85314176049903,-0.824352398286953,-0.813502334914016,
-0.685266505329869,-0.555745292861926,-0.425490955509816,-0.295356101878412,
-0.165943794724452,-0.0382708649850161,0.),.UNSPECIFIED.);
#470=B_SPLINE_CURVE_WITH_KNOTS('',3,(#31053,#31054,#31055,#31056,#31057,
#31058,#31059,#31060,#31061,#31062),.UNSPECIFIED.,.F.,.F.,(4,3,3,4),(-99.571617808197,
-99.0737597191561,-98.5759016301151,-98.3407704878033),.UNSPECIFIED.);
#471=B_SPLINE_CURVE_WITH_KNOTS('',3,(#31066,#31067,#31068,#31069,#31070,
#31071),.UNSPECIFIED.,.F.,.F.,(4,2,4),(0.,0.152964636529855,0.281059164612023),
 .UNSPECIFIED.);
#472=B_SPLINE_CURVE_WITH_KNOTS('',3,(#31075,#31076,#31077,#31078,#31079,
#31080,#31081,#31082,#31083,#31084),.UNSPECIFIED.,.F.,.F.,(4,2,2,2,4),(0.0909639115113299,
0.113933562624914,0.136903213738499,0.159492703061009,0.182082192383519),
 .UNSPECIFIED.);
#473=B_SPLINE_CURVE_WITH_KNOTS('',3,(#31090,#31091,#31092,#31093,#31094,
#31095),.UNSPECIFIED.,.F.,.F.,(4,2,4),(0.57279622617395,0.700890754256119,
0.853855390785973),.UNSPECIFIED.);
#474=B_SPLINE_CURVE_WITH_KNOTS('',3,(#31099,#31100,#31101,#31102,#31103,
#31104,#31105,#31106,#31107,#31108),.UNSPECIFIED.,.F.,.F.,(4,2,2,2,4),(0.,
0.036890778159456,0.073781556318912,0.147563112637824,0.287928080070797),
 .UNSPECIFIED.);
#475=B_SPLINE_CURVE_WITH_KNOTS('',3,(#31109,#31110,#31111,#31112,#31113,
#31114,#31115,#31116),.UNSPECIFIED.,.F.,.F.,(4,2,2,4),(-1.22072109304768,
-1.09399903701061,-0.96727698097355,-0.914517589488587),.UNSPECIFIED.);
#476=B_SPLINE_CURVE_WITH_KNOTS('',3,(#31118,#31119,#31120,#31121,#31122,
#31123,#31124,#31125),.UNSPECIFIED.,.F.,.F.,(4,2,2,4),(-0.306203503559089,
-0.253444112074126,-0.126722056037063,0.),.UNSPECIFIED.);
#477=B_SPLINE_CURVE_WITH_KNOTS('',3,(#31127,#31128,#31129,#31130,#31131,
#31132,#31133,#31134,#31135,#31136),.UNSPECIFIED.,.F.,.F.,(4,2,2,2,4),(-0.287928080070797,
-0.147563112637824,-0.0737815563189121,-0.0368907781594561,0.),
 .UNSPECIFIED.);
#478=B_SPLINE_CURVE_WITH_KNOTS('',3,(#31144,#31145,#31146,#31147,#31148,
#31149,#31150,#31151,#31152,#31153),.UNSPECIFIED.,.F.,.F.,(4,2,2,2,4),(0.182082136548056,
0.204671625870566,0.227261115193076,0.25023076630666,0.273200417420245),
 .UNSPECIFIED.);
#479=B_SPLINE_CURVE_WITH_KNOTS('',3,(#31158,#31159,#31160,#31161,#31162,
#31163,#31164,#31165,#31166,#31167),.UNSPECIFIED.,.F.,.F.,(4,2,2,2,4),(0.182082136548057,
0.204766091123424,0.22745004569879,0.250325299199413,0.267311238580278),
 .UNSPECIFIED.);
#480=B_SPLINE_CURVE_WITH_KNOTS('',3,(#31174,#31175,#31176,#31177,#31178,
#31179,#31180,#31181,#31182,#31183),.UNSPECIFIED.,.F.,.F.,(4,2,2,2,4),(0.0968538675768226,
0.113933506789453,0.136903157903037,0.159492647225547,0.182082136548057),
 .UNSPECIFIED.);
#481=B_SPLINE_CURVE_WITH_KNOTS('',3,(#31213,#31214,#31215,#31216,#31217,
#31218,#31219,#31220,#31221,#31222,#31223,#31224,#31225,#31226,#31227,#31228,
#31229,#31230,#31231,#31232,#31233,#31234,#31235,#31236,#31237,#31238,#31239),
 .UNSPECIFIED.,.F.,.F.,(4,2,2,2,2,2,3,2,2,2,2,2,4),(5.99649261281881,6.24600544998076,
6.4955182871427,6.99454396146659,7.4949337226125,7.74512860318546,7.99532348375842,
8.24551836433138,8.49571324490433,8.99610300605025,9.49512868037414,9.74464151753608,
9.99415435469802),.UNSPECIFIED.);
#482=B_SPLINE_CURVE_WITH_KNOTS('',3,(#31240,#31241,#31242,#31243,#31244,
#31245,#31246,#31247,#31248,#31249,#31250,#31251,#31252,#31253,#31254,#31255,
#31256,#31257,#31258,#31259,#31260,#31261,#31262,#31263,#31264,#31265),
 .UNSPECIFIED.,.F.,.F.,(4,2,2,2,2,2,2,2,2,2,2,2,4),(9.99415435469802,10.24366719186,
10.4931800290219,10.9922057033458,11.4925954644917,11.7427903450647,11.9929852256376,
12.2431801062106,12.4933749867835,12.9937647479295,13.4927904222533,13.7423032594153,
13.9918160965772),.UNSPECIFIED.);
#483=B_SPLINE_CURVE_WITH_KNOTS('',3,(#31267,#31268,#31269,#31270,#31271,
#31272,#31273,#31274,#31275,#31276,#31277,#31278,#31279,#31280,#31281,#31282,
#31283,#31284,#31285,#31286,#31287,#31288,#31289,#31290,#31291,#31292,#31293,
#31294,#31295,#31296,#31297),.UNSPECIFIED.,.F.,.F.,(4,2,2,2,2,2,2,2,2,2,
2,3,2,2,4),(1.95850633937799,2.2855721728953,2.6667178301167,3.04786348733809,
3.42900914455948,3.81015480178088,4.19097501639401,4.57179523100713,4.95261544562026,
5.33343566023339,5.71458131745479,6.09572697467618,6.47687263189757,6.85801828911897,
7.18508412263628),.UNSPECIFIED.);
#853=B_SPLINE_SURFACE_WITH_KNOTS('',3,3,((#27715,#27716,#27717,#27718,#27719,
#27720,#27721,#27722,#27723,#27724,#27725,#27726,#27727,#27728,#27729,#27730,
#27731,#27732,#27733,#27734,#27735,#27736,#27737,#27738,#27739,#27740,#27741,
#27742,#27743,#27744,#27745,#27746,#27747,#27748,#27749,#27750,#27751,#27752,
#27753,#27754,#27755,#27756,#27757,#27758,#27759,#27760,#27761,#27762,#27763,
#27764,#27765,#27766,#27767,#27768,#27769,#27770,#27771,#27772,#27773,#27774,
#27775,#27776,#27777,#27778,#27779,#27780,#27781,#27782,#27783,#27784,#27785,
#27786,#27787,#27788,#27789,#27790,#27791,#27792,#27793,#27794,#27795,#27796,
#27797,#27798,#27799,#27800,#27801,#27802,#27803,#27804,#27805,#27806,#27807,
#27808,#27809,#27810,#27811,#27812,#27813,#27814,#27815,#27816,#27817,#27818,
#27819,#27820,#27821,#27822,#27823,#27824,#27825,#27826,#27827,#27828,#27829,
#27830,#27831,#27832,#27833,#27834,#27835,#27836,#27837,#27838,#27839,#27840,
#27841,#27842,#27843,#27844,#27845,#27846,#27847,#27848,#27849,#27850,#27851),
(#27852,#27853,#27854,#27855,#27856,#27857,#27858,#27859,#27860,#27861,
#27862,#27863,#27864,#27865,#27866,#27867,#27868,#27869,#27870,#27871,#27872,
#27873,#27874,#27875,#27876,#27877,#27878,#27879,#27880,#27881,#27882,#27883,
#27884,#27885,#27886,#27887,#27888,#27889,#27890,#27891,#27892,#27893,#27894,
#27895,#27896,#27897,#27898,#27899,#27900,#27901,#27902,#27903,#27904,#27905,
#27906,#27907,#27908,#27909,#27910,#27911,#27912,#27913,#27914,#27915,#27916,
#27917,#27918,#27919,#27920,#27921,#27922,#27923,#27924,#27925,#27926,#27927,
#27928,#27929,#27930,#27931,#27932,#27933,#27934,#27935,#27936,#27937,#27938,
#27939,#27940,#27941,#27942,#27943,#27944,#27945,#27946,#27947,#27948,#27949,
#27950,#27951,#27952,#27953,#27954,#27955,#27956,#27957,#27958,#27959,#27960,
#27961,#27962,#27963,#27964,#27965,#27966,#27967,#27968,#27969,#27970,#27971,
#27972,#27973,#27974,#27975,#27976,#27977,#27978,#27979,#27980,#27981,#27982,
#27983,#27984,#27985,#27986,#27987,#27988),(#27989,#27990,#27991,#27992,
#27993,#27994,#27995,#27996,#27997,#27998,#27999,#28000,#28001,#28002,#28003,
#28004,#28005,#28006,#28007,#28008,#28009,#28010,#28011,#28012,#28013,#28014,
#28015,#28016,#28017,#28018,#28019,#28020,#28021,#28022,#28023,#28024,#28025,
#28026,#28027,#28028,#28029,#28030,#28031,#28032,#28033,#28034,#28035,#28036,
#28037,#28038,#28039,#28040,#28041,#28042,#28043,#28044,#28045,#28046,#28047,
#28048,#28049,#28050,#28051,#28052,#28053,#28054,#28055,#28056,#28057,#28058,
#28059,#28060,#28061,#28062,#28063,#28064,#28065,#28066,#28067,#28068,#28069,
#28070,#28071,#28072,#28073,#28074,#28075,#28076,#28077,#28078,#28079,#28080,
#28081,#28082,#28083,#28084,#28085,#28086,#28087,#28088,#28089,#28090,#28091,
#28092,#28093,#28094,#28095,#28096,#28097,#28098,#28099,#28100,#28101,#28102,
#28103,#28104,#28105,#28106,#28107,#28108,#28109,#28110,#28111,#28112,#28113,
#28114,#28115,#28116,#28117,#28118,#28119,#28120,#28121,#28122,#28123,#28124,
#28125),(#28126,#28127,#28128,#28129,#28130,#28131,#28132,#28133,#28134,
#28135,#28136,#28137,#28138,#28139,#28140,#28141,#28142,#28143,#28144,#28145,
#28146,#28147,#28148,#28149,#28150,#28151,#28152,#28153,#28154,#28155,#28156,
#28157,#28158,#28159,#28160,#28161,#28162,#28163,#28164,#28165,#28166,#28167,
#28168,#28169,#28170,#28171,#28172,#28173,#28174,#28175,#28176,#28177,#28178,
#28179,#28180,#28181,#28182,#28183,#28184,#28185,#28186,#28187,#28188,#28189,
#28190,#28191,#28192,#28193,#28194,#28195,#28196,#28197,#28198,#28199,#28200,
#28201,#28202,#28203,#28204,#28205,#28206,#28207,#28208,#28209,#28210,#28211,
#28212,#28213,#28214,#28215,#28216,#28217,#28218,#28219,#28220,#28221,#28222,
#28223,#28224,#28225,#28226,#28227,#28228,#28229,#28230,#28231,#28232,#28233,
#28234,#28235,#28236,#28237,#28238,#28239,#28240,#28241,#28242,#28243,#28244,
#28245,#28246,#28247,#28248,#28249,#28250,#28251,#28252,#28253,#28254,#28255,
#28256,#28257,#28258,#28259,#28260,#28261,#28262)),.UNSPECIFIED.,.F.,.F.,
 .F.,(4,4),(4,1,1,1,1,1,1,1,1,1,1,1,1,1,1,1,1,1,1,1,1,1,1,1,1,1,1,1,1,1,
1,1,1,1,1,1,1,1,1,1,1,1,1,1,1,1,1,1,1,1,1,1,1,1,1,1,1,1,1,1,1,1,1,1,1,1,
1,1,1,1,1,1,1,1,1,1,1,1,1,1,1,1,1,1,1,1,1,1,1,1,1,1,1,1,1,1,1,1,1,1,1,1,
1,1,1,1,1,1,1,1,1,1,1,1,1,1,1,1,1,1,1,1,1,1,1,1,1,1,1,1,1,1,1,1,4),(0.,
0.0991945497494695),(8.29865039549515,8.79164514303176,9.28463989056837,
9.77763463810498,10.2706293856416,10.7636241331782,11.2566188807148,11.7496136282514,
12.242608375788,12.7356031233247,13.2285978708613,13.7215926183979,14.2145873659345,
14.7075821134711,15.2005768610077,15.6935716085443,16.1865663560809,16.6795611036176,
17.1725558511542,17.6655505986908,18.1585453462274,18.651540093764,19.1445348413006,
19.6375295888372,20.1305243363738,20.6235190839104,21.1165138314471,21.6095085789837,
22.1025033265203,22.5954980740569,23.0884928215935,23.5814875691301,24.0744823166667,
24.5674770642033,25.06047181174,25.5534665592766,26.0464613068132,26.5394560543498,
27.0324508018864,27.525445549423,28.0184402969596,28.5114350444962,29.0044297920328,
29.4974245395695,29.9904192871061,30.4834140346427,30.9764087821793,31.4694035297159,
31.9623982772525,32.4553930247891,32.9483877723257,33.4413825198624,33.934377267399,
34.4273720149356,34.9203667624722,35.4133615100088,35.9063562575454,36.399351005082,
36.8923457526186,37.3853405001553,37.8783352476919,38.3713299952285,38.8643247427651,
39.3573194903017,39.8503142378383,40.3433089853749,40.8363037329115,41.3292984804481,
41.8222932279848,42.3152879755214,42.808282723058,43.3012774705946,43.7942722181312,
44.2872669656678,44.7802617132044,45.273256460741,45.7662512082777,46.2592459558143,
46.7522407033509,47.2452354508875,47.7382301984241,48.2312249459607,48.7242196934973,
49.2172144410339,49.7102091885705,50.2032039361072,50.6961986836438,51.1891934311804,
51.682188178717,52.1751829262536,52.6681776737902,53.1611724213268,53.6541671688635,
54.1471619164001,54.6401566639367,55.1331514114733,55.6261461590099,56.1191409065465,
56.6121356540831,57.1051304016197,57.5981251491563,58.091119896693,58.5841146442296,
59.0771093917662,59.5701041393028,60.0630988868394,60.556093634376,61.0490883819126,
61.5420831294492,62.0350778769859,62.5280726245225,63.0210673720591,63.5140621195957,
64.0070568671323,64.5000516146689,64.9930463622055,65.4860411097421,65.9790358572787,
66.4720306048154,66.965025352352,67.4580200998886,67.9510148474252,68.4440095949618,
68.9370043424984,69.429999090035,69.9229938375716,70.4159885851083,70.9089833326449,
71.4019780801815,71.8949728277181,72.3879675752547,72.8809623227913,73.3739570703279,
73.8669518178645,74.3599465654011),.UNSPECIFIED.);
#854=B_SPLINE_SURFACE_WITH_KNOTS('',3,3,((#28295,#28296,#28297,#28298,#28299,
#28300,#28301,#28302,#28303,#28304,#28305,#28306,#28307,#28308,#28309,#28310,
#28311,#28312,#28313,#28314,#28315,#28316,#28317,#28318,#28319,#28320,#28321,
#28322,#28323,#28324,#28325,#28326,#28327,#28328,#28329,#28330,#28331,#28332,
#28333,#28334,#28335,#28336,#28337,#28338,#28339,#28340,#28341,#28342,#28343,
#28344,#28345,#28346,#28347,#28348,#28349,#28350,#28351,#28352,#28353,#28354,
#28355,#28356,#28357,#28358,#28359,#28360,#28361,#28362,#28363,#28364,#28365,
#28366,#28367,#28368,#28369,#28370,#28371,#28372,#28373,#28374,#28375,#28376,
#28377,#28378,#28379,#28380,#28381,#28382,#28383,#28384,#28385,#28386,#28387,
#28388,#28389,#28390,#28391,#28392,#28393,#28394,#28395,#28396,#28397,#28398,
#28399,#28400,#28401,#28402,#28403,#28404,#28405,#28406,#28407,#28408,#28409,
#28410,#28411,#28412,#28413,#28414,#28415,#28416,#28417,#28418,#28419,#28420,
#28421,#28422,#28423,#28424,#28425,#28426,#28427,#28428,#28429,#28430,#28431),
(#28432,#28433,#28434,#28435,#28436,#28437,#28438,#28439,#28440,#28441,
#28442,#28443,#28444,#28445,#28446,#28447,#28448,#28449,#28450,#28451,#28452,
#28453,#28454,#28455,#28456,#28457,#28458,#28459,#28460,#28461,#28462,#28463,
#28464,#28465,#28466,#28467,#28468,#28469,#28470,#28471,#28472,#28473,#28474,
#28475,#28476,#28477,#28478,#28479,#28480,#28481,#28482,#28483,#28484,#28485,
#28486,#28487,#28488,#28489,#28490,#28491,#28492,#28493,#28494,#28495,#28496,
#28497,#28498,#28499,#28500,#28501,#28502,#28503,#28504,#28505,#28506,#28507,
#28508,#28509,#28510,#28511,#28512,#28513,#28514,#28515,#28516,#28517,#28518,
#28519,#28520,#28521,#28522,#28523,#28524,#28525,#28526,#28527,#28528,#28529,
#28530,#28531,#28532,#28533,#28534,#28535,#28536,#28537,#28538,#28539,#28540,
#28541,#28542,#28543,#28544,#28545,#28546,#28547,#28548,#28549,#28550,#28551,
#28552,#28553,#28554,#28555,#28556,#28557,#28558,#28559,#28560,#28561,#28562,
#28563,#28564,#28565,#28566,#28567,#28568),(#28569,#28570,#28571,#28572,
#28573,#28574,#28575,#28576,#28577,#28578,#28579,#28580,#28581,#28582,#28583,
#28584,#28585,#28586,#28587,#28588,#28589,#28590,#28591,#28592,#28593,#28594,
#28595,#28596,#28597,#28598,#28599,#28600,#28601,#28602,#28603,#28604,#28605,
#28606,#28607,#28608,#28609,#28610,#28611,#28612,#28613,#28614,#28615,#28616,
#28617,#28618,#28619,#28620,#28621,#28622,#28623,#28624,#28625,#28626,#28627,
#28628,#28629,#28630,#28631,#28632,#28633,#28634,#28635,#28636,#28637,#28638,
#28639,#28640,#28641,#28642,#28643,#28644,#28645,#28646,#28647,#28648,#28649,
#28650,#28651,#28652,#28653,#28654,#28655,#28656,#28657,#28658,#28659,#28660,
#28661,#28662,#28663,#28664,#28665,#28666,#28667,#28668,#28669,#28670,#28671,
#28672,#28673,#28674,#28675,#28676,#28677,#28678,#28679,#28680,#28681,#28682,
#28683,#28684,#28685,#28686,#28687,#28688,#28689,#28690,#28691,#28692,#28693,
#28694,#28695,#28696,#28697,#28698,#28699,#28700,#28701,#28702,#28703,#28704,
#28705),(#28706,#28707,#28708,#28709,#28710,#28711,#28712,#28713,#28714,
#28715,#28716,#28717,#28718,#28719,#28720,#28721,#28722,#28723,#28724,#28725,
#28726,#28727,#28728,#28729,#28730,#28731,#28732,#28733,#28734,#28735,#28736,
#28737,#28738,#28739,#28740,#28741,#28742,#28743,#28744,#28745,#28746,#28747,
#28748,#28749,#28750,#28751,#28752,#28753,#28754,#28755,#28756,#28757,#28758,
#28759,#28760,#28761,#28762,#28763,#28764,#28765,#28766,#28767,#28768,#28769,
#28770,#28771,#28772,#28773,#28774,#28775,#28776,#28777,#28778,#28779,#28780,
#28781,#28782,#28783,#28784,#28785,#28786,#28787,#28788,#28789,#28790,#28791,
#28792,#28793,#28794,#28795,#28796,#28797,#28798,#28799,#28800,#28801,#28802,
#28803,#28804,#28805,#28806,#28807,#28808,#28809,#28810,#28811,#28812,#28813,
#28814,#28815,#28816,#28817,#28818,#28819,#28820,#28821,#28822,#28823,#28824,
#28825,#28826,#28827,#28828,#28829,#28830,#28831,#28832,#28833,#28834,#28835,
#28836,#28837,#28838,#28839,#28840,#28841,#28842)),.UNSPECIFIED.,.F.,.F.,
 .F.,(4,4),(4,1,1,1,1,1,1,1,1,1,1,1,1,1,1,1,1,1,1,1,1,1,1,1,1,1,1,1,1,1,
1,1,1,1,1,1,1,1,1,1,1,1,1,1,1,1,1,1,1,1,1,1,1,1,1,1,1,1,1,1,1,1,1,1,1,1,
1,1,1,1,1,1,1,1,1,1,1,1,1,1,1,1,1,1,1,1,1,1,1,1,1,1,1,1,1,1,1,1,1,1,1,1,
1,1,1,1,1,1,1,1,1,1,1,1,1,1,1,1,1,1,1,1,1,1,1,1,1,1,1,1,1,1,1,1,4),(0.,
0.0991945497494695),(11.6149723878394,12.107967135376,12.6009618829127,
13.0939566304493,13.5869513779859,14.0799461255225,14.5729408730591,15.0659356205957,
15.5589303681323,16.0519251156689,16.5449198632055,17.0379146107422,17.5309093582788,
18.0239041058154,18.516898853352,19.0098936008886,19.5028883484252,19.9958830959618,
20.4888778434984,20.9818725910351,21.4748673385717,21.9678620861083,22.4608568336449,
22.9538515811815,23.4468463287181,23.9398410762547,24.4328358237913,24.925830571328,
25.4188253188646,25.9118200664012,26.4048148139378,26.8978095614744,27.390804309011,
27.8837990565476,28.3767938040842,28.8697885516209,29.3627832991575,29.8557780466941,
30.3487727942307,30.8417675417673,31.3347622893039,31.8277570368405,32.3207517843771,
32.8137465319137,33.3067412794504,33.799736026987,34.2927307745236,34.7857255220602,
35.2787202695968,35.7717150171334,36.26470976467,36.7577045122066,37.2506992597433,
37.7436940072799,38.2366887548165,38.7296835023531,39.2226782498897,39.7156729974263,
40.2086677449629,40.7016624924995,41.1946572400362,41.6876519875728,42.1806467351094,
42.673641482646,43.1666362301826,43.6596309777192,44.1526257252558,44.6456204727924,
45.138615220329,45.6316099678657,46.1246047154023,46.6175994629389,47.1105942104755,
47.6035889580121,48.0965837055487,48.5895784530853,49.0825732006219,49.5755679481586,
50.0685626956952,50.5615574432318,51.0545521907684,51.547546938305,52.0405416858416,
52.5335364333782,53.0265311809148,53.5195259284514,54.0125206759881,54.5055154235247,
54.9985101710613,55.4915049185979,55.9844996661345,56.4774944136711,56.9704891612077,
57.4634839087443,57.956478656281,58.4494734038176,58.9424681513542,59.4354628988908,
59.9284576464274,60.421452393964,60.9144471415006,61.4074418890372,61.9004366365738,
62.3934313841105,62.8864261316471,63.3794208791837,63.8724156267203,64.3654103742569,
64.8584051217935,65.3513998693301,65.8443946168668,66.3373893644034,66.83038411194,
67.3233788594766,67.8163736070132,68.3093683545498,68.8023631020864,69.295357849623,
69.7883525971596,70.2813473446963,70.7743420922329,71.2673368397695,71.7603315873061,
72.2533263348427,72.7463210823793,73.2393158299159,73.7323105774525,74.2253053249892,
74.7183000725258,75.2112948200624,75.704289567599,76.1972843151356,76.6902790626722,
77.1832738102088,77.6762685577454),.UNSPECIFIED.);
#855=B_SPLINE_SURFACE_WITH_KNOTS('',3,3,((#28845,#28846,#28847,#28848,#28849,
#28850,#28851,#28852,#28853,#28854,#28855,#28856,#28857,#28858,#28859,#28860,
#28861,#28862,#28863,#28864,#28865,#28866,#28867,#28868,#28869,#28870,#28871,
#28872,#28873,#28874,#28875,#28876,#28877,#28878,#28879,#28880,#28881,#28882,
#28883,#28884,#28885,#28886,#28887,#28888,#28889,#28890,#28891,#28892,#28893,
#28894,#28895,#28896,#28897,#28898,#28899,#28900,#28901,#28902,#28903,#28904,
#28905,#28906,#28907,#28908,#28909,#28910,#28911,#28912,#28913,#28914,#28915,
#28916,#28917,#28918,#28919,#28920,#28921,#28922,#28923,#28924,#28925,#28926,
#28927,#28928,#28929,#28930,#28931,#28932,#28933,#28934,#28935,#28936,#28937,
#28938,#28939,#28940,#28941,#28942,#28943,#28944,#28945,#28946,#28947,#28948,
#28949,#28950,#28951,#28952,#28953,#28954,#28955,#28956,#28957,#28958,#28959,
#28960,#28961,#28962,#28963,#28964,#28965,#28966,#28967,#28968,#28969,#28970,
#28971,#28972,#28973,#28974,#28975,#28976,#28977,#28978,#28979,#28980,#28981,
#28982,#28983,#28984,#28985,#28986,#28987,#28988,#28989,#28990,#28991,#28992,
#28993,#28994,#28995,#28996,#28997,#28998,#28999,#29000,#29001,#29002,#29003,
#29004,#29005,#29006,#29007,#29008,#29009,#29010,#29011,#29012,#29013,#29014,
#29015,#29016,#29017,#29018,#29019,#29020,#29021,#29022,#29023,#29024,#29025,
#29026,#29027,#29028,#29029,#29030,#29031,#29032,#29033,#29034,#29035,#29036,
#29037,#29038,#29039,#29040,#29041,#29042,#29043,#29044,#29045,#29046,#29047),
(#29048,#29049,#29050,#29051,#29052,#29053,#29054,#29055,#29056,#29057,
#29058,#29059,#29060,#29061,#29062,#29063,#29064,#29065,#29066,#29067,#29068,
#29069,#29070,#29071,#29072,#29073,#29074,#29075,#29076,#29077,#29078,#29079,
#29080,#29081,#29082,#29083,#29084,#29085,#29086,#29087,#29088,#29089,#29090,
#29091,#29092,#29093,#29094,#29095,#29096,#29097,#29098,#29099,#29100,#29101,
#29102,#29103,#29104,#29105,#29106,#29107,#29108,#29109,#29110,#29111,#29112,
#29113,#29114,#29115,#29116,#29117,#29118,#29119,#29120,#29121,#29122,#29123,
#29124,#29125,#29126,#29127,#29128,#29129,#29130,#29131,#29132,#29133,#29134,
#29135,#29136,#29137,#29138,#29139,#29140,#29141,#29142,#29143,#29144,#29145,
#29146,#29147,#29148,#29149,#29150,#29151,#29152,#29153,#29154,#29155,#29156,
#29157,#29158,#29159,#29160,#29161,#29162,#29163,#29164,#29165,#29166,#29167,
#29168,#29169,#29170,#29171,#29172,#29173,#29174,#29175,#29176,#29177,#29178,
#29179,#29180,#29181,#29182,#29183,#29184,#29185,#29186,#29187,#29188,#29189,
#29190,#29191,#29192,#29193,#29194,#29195,#29196,#29197,#29198,#29199,#29200,
#29201,#29202,#29203,#29204,#29205,#29206,#29207,#29208,#29209,#29210,#29211,
#29212,#29213,#29214,#29215,#29216,#29217,#29218,#29219,#29220,#29221,#29222,
#29223,#29224,#29225,#29226,#29227,#29228,#29229,#29230,#29231,#29232,#29233,
#29234,#29235,#29236,#29237,#29238,#29239,#29240,#29241,#29242,#29243,#29244,
#29245,#29246,#29247,#29248,#29249,#29250),(#29251,#29252,#29253,#29254,
#29255,#29256,#29257,#29258,#29259,#29260,#29261,#29262,#29263,#29264,#29265,
#29266,#29267,#29268,#29269,#29270,#29271,#29272,#29273,#29274,#29275,#29276,
#29277,#29278,#29279,#29280,#29281,#29282,#29283,#29284,#29285,#29286,#29287,
#29288,#29289,#29290,#29291,#29292,#29293,#29294,#29295,#29296,#29297,#29298,
#29299,#29300,#29301,#29302,#29303,#29304,#29305,#29306,#29307,#29308,#29309,
#29310,#29311,#29312,#29313,#29314,#29315,#29316,#29317,#29318,#29319,#29320,
#29321,#29322,#29323,#29324,#29325,#29326,#29327,#29328,#29329,#29330,#29331,
#29332,#29333,#29334,#29335,#29336,#29337,#29338,#29339,#29340,#29341,#29342,
#29343,#29344,#29345,#29346,#29347,#29348,#29349,#29350,#29351,#29352,#29353,
#29354,#29355,#29356,#29357,#29358,#29359,#29360,#29361,#29362,#29363,#29364,
#29365,#29366,#29367,#29368,#29369,#29370,#29371,#29372,#29373,#29374,#29375,
#29376,#29377,#29378,#29379,#29380,#29381,#29382,#29383,#29384,#29385,#29386,
#29387,#29388,#29389,#29390,#29391,#29392,#29393,#29394,#29395,#29396,#29397,
#29398,#29399,#29400,#29401,#29402,#29403,#29404,#29405,#29406,#29407,#29408,
#29409,#29410,#29411,#29412,#29413,#29414,#29415,#29416,#29417,#29418,#29419,
#29420,#29421,#29422,#29423,#29424,#29425,#29426,#29427,#29428,#29429,#29430,
#29431,#29432,#29433,#29434,#29435,#29436,#29437,#29438,#29439,#29440,#29441,
#29442,#29443,#29444,#29445,#29446,#29447,#29448,#29449,#29450,#29451,#29452,
#29453),(#29454,#29455,#29456,#29457,#29458,#29459,#29460,#29461,#29462,
#29463,#29464,#29465,#29466,#29467,#29468,#29469,#29470,#29471,#29472,#29473,
#29474,#29475,#29476,#29477,#29478,#29479,#29480,#29481,#29482,#29483,#29484,
#29485,#29486,#29487,#29488,#29489,#29490,#29491,#29492,#29493,#29494,#29495,
#29496,#29497,#29498,#29499,#29500,#29501,#29502,#29503,#29504,#29505,#29506,
#29507,#29508,#29509,#29510,#29511,#29512,#29513,#29514,#29515,#29516,#29517,
#29518,#29519,#29520,#29521,#29522,#29523,#29524,#29525,#29526,#29527,#29528,
#29529,#29530,#29531,#29532,#29533,#29534,#29535,#29536,#29537,#29538,#29539,
#29540,#29541,#29542,#29543,#29544,#29545,#29546,#29547,#29548,#29549,#29550,
#29551,#29552,#29553,#29554,#29555,#29556,#29557,#29558,#29559,#29560,#29561,
#29562,#29563,#29564,#29565,#29566,#29567,#29568,#29569,#29570,#29571,#29572,
#29573,#29574,#29575,#29576,#29577,#29578,#29579,#29580,#29581,#29582,#29583,
#29584,#29585,#29586,#29587,#29588,#29589,#29590,#29591,#29592,#29593,#29594,
#29595,#29596,#29597,#29598,#29599,#29600,#29601,#29602,#29603,#29604,#29605,
#29606,#29607,#29608,#29609,#29610,#29611,#29612,#29613,#29614,#29615,#29616,
#29617,#29618,#29619,#29620,#29621,#29622,#29623,#29624,#29625,#29626,#29627,
#29628,#29629,#29630,#29631,#29632,#29633,#29634,#29635,#29636,#29637,#29638,
#29639,#29640,#29641,#29642,#29643,#29644,#29645,#29646,#29647,#29648,#29649,
#29650,#29651,#29652,#29653,#29654,#29655,#29656)),.UNSPECIFIED.,.F.,.F.,
 .F.,(4,4),(4,1,1,1,1,1,1,1,1,1,1,1,1,1,1,1,1,1,1,1,1,1,1,1,1,1,1,1,1,1,
1,1,1,1,1,1,1,1,1,1,1,1,1,1,1,1,1,1,1,1,1,1,1,1,1,1,1,1,1,1,1,1,1,1,1,1,
1,1,1,1,1,1,1,1,1,1,1,1,1,1,1,1,1,1,1,1,1,1,1,1,1,1,1,1,1,1,1,1,1,1,1,1,
1,1,1,1,1,1,1,1,1,1,1,1,1,1,1,1,1,1,1,1,1,1,1,1,1,1,1,1,1,1,1,1,1,1,1,1,
1,1,1,1,1,1,1,1,1,1,1,1,1,1,1,1,1,1,1,1,1,1,1,1,1,1,1,1,1,1,1,1,1,1,1,1,
1,1,1,1,1,1,1,1,1,1,1,1,1,1,1,1,1,1,1,1,1,1,1,1,1,1,4),(0.,0.0991945497494695),
(8.2986503954951,8.79650848453609,9.29436657357707,9.79222466261806,10.290082751659,
10.7879408407,11.285798929741,11.783657018782,12.281515107823,12.779373196864,
13.277231285905,13.7750893749459,14.2729474639869,14.7708055530279,15.2686636420689,
15.7665217311099,16.2643798201509,16.7622379091919,17.2600959982328,17.7579540872738,
18.2558121763148,18.7536702653558,19.2515283543968,19.7493864434378,20.2472445324787,
20.7451026215197,21.2429607105607,21.7408187996017,22.2386768886427,22.7365349776837,
23.2343930667247,23.7322511557656,24.2301092448066,24.7279673338476,25.2258254228886,
25.7236835119296,26.2215416009706,26.7193996900116,27.2172577790525,27.7151158680935,
28.2129739571345,28.7108320461755,29.2086901352165,29.7065482242575,30.2044063132985,
30.7022644023394,31.2001224913804,31.6979805804214,32.1958386694624,32.6936967585034,
33.1915548475444,33.6894129365854,34.1872710256263,34.6851291146673,35.1829872037083,
35.6808452927493,36.1787033817903,36.6765614708313,37.1744195598722,37.6722776489132,
38.1701357379542,38.6679938269952,39.1658519160362,39.6637100050772,40.1615680941182,
40.6594261831592,41.1572842722001,41.6551423612411,42.1530004502821,42.6508585393231,
43.1487166283641,43.6465747174051,44.144432806446,44.642290895487,45.140148984528,
45.638007073569,46.13586516261,46.633723251651,47.131581340692,47.6294394297329,
48.1272975187739,48.6251556078149,49.1230136968559,49.6208717858969,50.1187298749379,
50.6165879639789,51.1144460530198,51.6123041420608,52.1101622311018,52.6080203201428,
53.1058784091838,53.6037364982248,54.1015945872658,54.5994526763067,55.0973107653477,
55.5951688543887,56.0930269434297,56.5908850324707,57.0887431215117,57.5866012105526,
58.0844592995936,58.5823173886346,59.0801754776756,59.5780335667166,60.0758916557576,
60.5737497447986,61.0716078338395,61.5694659228805,62.0673240119215,62.5651821009625,
63.0630401900035,63.5608982790445,64.0587563680855,64.5566144571264,65.0544725461674,
65.5523306352084,66.0501887242494,66.5480468132904,67.0459049023314,67.5437629913723,
68.0416210804133,68.5394791694543,69.0373372584953,69.5351953475363,70.0330534365773,
70.5309115256183,71.0287696146593,71.5266277037002,72.0244857927412,72.5223438817822,
73.0202019708232,73.5180600598642,74.0159181489052,74.5137762379462,75.0116343269871,
75.5094924160281,76.0073505050691,76.5052085941101,77.0030666831511,77.5009247721921,
77.9987828612331,78.496640950274,78.994499039315,79.492357128356,79.990215217397,
80.488073306438,80.985931395479,81.4837894845199,81.9816475735609,82.4795056626019,
82.9773637516429,83.4752218406839,83.9730799297249,84.4709380187658,84.9687961078068,
85.4666541968478,85.9645122858888,86.4623703749298,86.9602284639708,87.4580865530118,
87.9559446420528,88.4538027310937,88.9516608201347,89.4495189091757,89.9473769982167,
90.4452350872577,90.9430931762987,91.4409512653396,91.9388093543806,92.4366674434216,
92.9345255324626,93.4323836215036,93.9302417105446,94.4280997995856,94.9259578886266,
95.4238159776675,95.9216740667085,96.4195321557495,96.9173902447905,97.4152483338315,
97.9131064228725,98.4109645119134,98.9088226009544,99.4066806899954,99.9045387790364,
100.402396868077,100.900254957118,101.398113046159,101.8959711352,102.393829224241,
102.891687313282,103.389545402323,103.887403491364,104.385261580405,104.883119669446,
105.380977758487,105.878835847528,106.376693936569,106.87455202561,107.372410114651,
107.870268203692),.UNSPECIFIED.);
#856=B_SPLINE_SURFACE_WITH_KNOTS('',3,3,((#30110,#30111,#30112,#30113,#30114,
#30115,#30116,#30117,#30118,#30119,#30120,#30121,#30122,#30123,#30124,#30125,
#30126,#30127,#30128,#30129,#30130,#30131,#30132,#30133,#30134,#30135,#30136,
#30137,#30138,#30139,#30140,#30141,#30142,#30143,#30144,#30145,#30146,#30147,
#30148,#30149,#30150,#30151,#30152,#30153,#30154,#30155,#30156,#30157,#30158,
#30159,#30160,#30161,#30162,#30163,#30164,#30165,#30166,#30167,#30168,#30169,
#30170,#30171,#30172,#30173,#30174,#30175,#30176,#30177,#30178,#30179,#30180,
#30181,#30182,#30183,#30184,#30185,#30186,#30187,#30188,#30189,#30190,#30191,
#30192,#30193,#30194,#30195,#30196,#30197,#30198,#30199,#30200,#30201,#30202,
#30203,#30204,#30205,#30206,#30207,#30208,#30209,#30210,#30211,#30212,#30213,
#30214,#30215,#30216,#30217,#30218,#30219,#30220,#30221,#30222,#30223,#30224,
#30225,#30226,#30227,#30228,#30229,#30230,#30231,#30232,#30233,#30234,#30235,
#30236,#30237,#30238,#30239,#30240,#30241,#30242,#30243,#30244,#30245,#30246,
#30247,#30248,#30249,#30250,#30251,#30252,#30253,#30254,#30255,#30256,#30257,
#30258,#30259,#30260,#30261,#30262,#30263,#30264,#30265,#30266,#30267,#30268,
#30269,#30270,#30271,#30272,#30273,#30274,#30275,#30276,#30277,#30278,#30279,
#30280,#30281,#30282,#30283,#30284,#30285,#30286,#30287,#30288,#30289,#30290,
#30291,#30292,#30293,#30294,#30295,#30296,#30297,#30298,#30299,#30300,#30301,
#30302,#30303,#30304,#30305,#30306,#30307,#30308,#30309,#30310,#30311,#30312),
(#30313,#30314,#30315,#30316,#30317,#30318,#30319,#30320,#30321,#30322,
#30323,#30324,#30325,#30326,#30327,#30328,#30329,#30330,#30331,#30332,#30333,
#30334,#30335,#30336,#30337,#30338,#30339,#30340,#30341,#30342,#30343,#30344,
#30345,#30346,#30347,#30348,#30349,#30350,#30351,#30352,#30353,#30354,#30355,
#30356,#30357,#30358,#30359,#30360,#30361,#30362,#30363,#30364,#30365,#30366,
#30367,#30368,#30369,#30370,#30371,#30372,#30373,#30374,#30375,#30376,#30377,
#30378,#30379,#30380,#30381,#30382,#30383,#30384,#30385,#30386,#30387,#30388,
#30389,#30390,#30391,#30392,#30393,#30394,#30395,#30396,#30397,#30398,#30399,
#30400,#30401,#30402,#30403,#30404,#30405,#30406,#30407,#30408,#30409,#30410,
#30411,#30412,#30413,#30414,#30415,#30416,#30417,#30418,#30419,#30420,#30421,
#30422,#30423,#30424,#30425,#30426,#30427,#30428,#30429,#30430,#30431,#30432,
#30433,#30434,#30435,#30436,#30437,#30438,#30439,#30440,#30441,#30442,#30443,
#30444,#30445,#30446,#30447,#30448,#30449,#30450,#30451,#30452,#30453,#30454,
#30455,#30456,#30457,#30458,#30459,#30460,#30461,#30462,#30463,#30464,#30465,
#30466,#30467,#30468,#30469,#30470,#30471,#30472,#30473,#30474,#30475,#30476,
#30477,#30478,#30479,#30480,#30481,#30482,#30483,#30484,#30485,#30486,#30487,
#30488,#30489,#30490,#30491,#30492,#30493,#30494,#30495,#30496,#30497,#30498,
#30499,#30500,#30501,#30502,#30503,#30504,#30505,#30506,#30507,#30508,#30509,
#30510,#30511,#30512,#30513,#30514,#30515),(#30516,#30517,#30518,#30519,
#30520,#30521,#30522,#30523,#30524,#30525,#30526,#30527,#30528,#30529,#30530,
#30531,#30532,#30533,#30534,#30535,#30536,#30537,#30538,#30539,#30540,#30541,
#30542,#30543,#30544,#30545,#30546,#30547,#30548,#30549,#30550,#30551,#30552,
#30553,#30554,#30555,#30556,#30557,#30558,#30559,#30560,#30561,#30562,#30563,
#30564,#30565,#30566,#30567,#30568,#30569,#30570,#30571,#30572,#30573,#30574,
#30575,#30576,#30577,#30578,#30579,#30580,#30581,#30582,#30583,#30584,#30585,
#30586,#30587,#30588,#30589,#30590,#30591,#30592,#30593,#30594,#30595,#30596,
#30597,#30598,#30599,#30600,#30601,#30602,#30603,#30604,#30605,#30606,#30607,
#30608,#30609,#30610,#30611,#30612,#30613,#30614,#30615,#30616,#30617,#30618,
#30619,#30620,#30621,#30622,#30623,#30624,#30625,#30626,#30627,#30628,#30629,
#30630,#30631,#30632,#30633,#30634,#30635,#30636,#30637,#30638,#30639,#30640,
#30641,#30642,#30643,#30644,#30645,#30646,#30647,#30648,#30649,#30650,#30651,
#30652,#30653,#30654,#30655,#30656,#30657,#30658,#30659,#30660,#30661,#30662,
#30663,#30664,#30665,#30666,#30667,#30668,#30669,#30670,#30671,#30672,#30673,
#30674,#30675,#30676,#30677,#30678,#30679,#30680,#30681,#30682,#30683,#30684,
#30685,#30686,#30687,#30688,#30689,#30690,#30691,#30692,#30693,#30694,#30695,
#30696,#30697,#30698,#30699,#30700,#30701,#30702,#30703,#30704,#30705,#30706,
#30707,#30708,#30709,#30710,#30711,#30712,#30713,#30714,#30715,#30716,#30717,
#30718),(#30719,#30720,#30721,#30722,#30723,#30724,#30725,#30726,#30727,
#30728,#30729,#30730,#30731,#30732,#30733,#30734,#30735,#30736,#30737,#30738,
#30739,#30740,#30741,#30742,#30743,#30744,#30745,#30746,#30747,#30748,#30749,
#30750,#30751,#30752,#30753,#30754,#30755,#30756,#30757,#30758,#30759,#30760,
#30761,#30762,#30763,#30764,#30765,#30766,#30767,#30768,#30769,#30770,#30771,
#30772,#30773,#30774,#30775,#30776,#30777,#30778,#30779,#30780,#30781,#30782,
#30783,#30784,#30785,#30786,#30787,#30788,#30789,#30790,#30791,#30792,#30793,
#30794,#30795,#30796,#30797,#30798,#30799,#30800,#30801,#30802,#30803,#30804,
#30805,#30806,#30807,#30808,#30809,#30810,#30811,#30812,#30813,#30814,#30815,
#30816,#30817,#30818,#30819,#30820,#30821,#30822,#30823,#30824,#30825,#30826,
#30827,#30828,#30829,#30830,#30831,#30832,#30833,#30834,#30835,#30836,#30837,
#30838,#30839,#30840,#30841,#30842,#30843,#30844,#30845,#30846,#30847,#30848,
#30849,#30850,#30851,#30852,#30853,#30854,#30855,#30856,#30857,#30858,#30859,
#30860,#30861,#30862,#30863,#30864,#30865,#30866,#30867,#30868,#30869,#30870,
#30871,#30872,#30873,#30874,#30875,#30876,#30877,#30878,#30879,#30880,#30881,
#30882,#30883,#30884,#30885,#30886,#30887,#30888,#30889,#30890,#30891,#30892,
#30893,#30894,#30895,#30896,#30897,#30898,#30899,#30900,#30901,#30902,#30903,
#30904,#30905,#30906,#30907,#30908,#30909,#30910,#30911,#30912,#30913,#30914,
#30915,#30916,#30917,#30918,#30919,#30920,#30921)),.UNSPECIFIED.,.F.,.F.,
 .F.,(4,4),(4,1,1,1,1,1,1,1,1,1,1,1,1,1,1,1,1,1,1,1,1,1,1,1,1,1,1,1,1,1,
1,1,1,1,1,1,1,1,1,1,1,1,1,1,1,1,1,1,1,1,1,1,1,1,1,1,1,1,1,1,1,1,1,1,1,1,
1,1,1,1,1,1,1,1,1,1,1,1,1,1,1,1,1,1,1,1,1,1,1,1,1,1,1,1,1,1,1,1,1,1,1,1,
1,1,1,1,1,1,1,1,1,1,1,1,1,1,1,1,1,1,1,1,1,1,1,1,1,1,1,1,1,1,1,1,1,1,1,1,
1,1,1,1,1,1,1,1,1,1,1,1,1,1,1,1,1,1,1,1,1,1,1,1,1,1,1,1,1,1,1,1,1,1,1,1,
1,1,1,1,1,1,1,1,1,1,1,1,1,1,1,1,1,1,1,1,1,1,1,1,1,1,4),(0.,0.0991945497494695),
(11.6149723878395,12.1128304768804,12.6106885659214,13.1085466549624,13.6064047440034,
14.1042628330444,14.6021209220854,15.0999790111264,15.5978371001673,16.0956951892083,
16.5935532782493,17.0914113672903,17.5892694563313,18.0871275453723,18.5849856344133,
19.0828437234542,19.5807018124952,20.0785599015362,20.5764179905772,21.0742760796182,
21.5721341686592,22.0699922577002,22.5678503467411,23.0657084357821,23.5635665248231,
24.0614246138641,24.5592827029051,25.0571407919461,25.554998880987,26.052856970028,
26.550715059069,27.04857314811,27.546431237151,28.044289326192,28.542147415233,
29.0400055042739,29.5378635933149,30.0357216823559,30.5335797713969,31.0314378604379,
31.5292959494789,32.0271540385199,32.5250121275608,33.0228702166018,33.5207283056428,
34.0185863946838,34.5164444837248,35.0143025727658,35.5121606618068,36.0100187508477,
36.5078768398887,37.0057349289297,37.5035930179707,38.0014511070117,38.4993091960527,
38.9971672850937,39.4950253741346,39.9928834631756,40.4907415522166,40.9885996412576,
41.4864577302986,41.9843158193396,42.4821739083806,42.9800319974215,43.4778900864625,
43.9757481755035,44.4736062645445,44.9714643535855,45.4693224426265,45.9671805316675,
46.4650386207084,46.9628967097494,47.4607547987904,47.9586128878314,48.4564709768724,
48.9543290659134,49.4521871549543,49.9500452439953,50.4479033330363,50.9457614220773,
51.4436195111183,51.9414776001593,52.4393356892003,52.9371937782412,53.4350518672822,
53.9329099563232,54.4307680453642,54.9286261344052,55.4264842234462,55.9243423124872,
56.4222004015281,56.9200584905691,57.4179165796101,57.9157746686511,58.4136327576921,
58.9114908467331,59.409348935774,59.907207024815,60.405065113856,60.902923202897,
61.400781291938,61.898639380979,62.39649747002,62.8943555590609,63.3922136481019,
63.8900717371429,64.3879298261839,64.8857879152249,65.3836460042659,65.8815040933069,
66.3793621823478,66.8772202713888,67.3750783604298,67.8729364494708,68.3707945385118,
68.8686526275528,69.3665107165938,69.8643688056347,70.3622268946757,70.8600849837167,
71.3579430727577,71.8558011617987,72.3536592508397,72.8515173398807,73.3493754289216,
73.8472335179626,74.3450916070036,74.8429496960446,75.3408077850856,75.8386658741266,
76.3365239631676,76.8343820522085,77.3322401412495,77.8300982302905,78.3279563193315,
78.8258144083725,79.3236724974135,79.8215305864545,80.3193886754954,80.8172467645364,
81.3151048535774,81.8129629426184,82.3108210316594,82.8086791207004,83.3065372097414,
83.8043952987823,84.3022533878233,84.8001114768643,85.2979695659053,85.7958276549463,
86.2936857439873,86.7915438330282,87.2894019220692,87.7872600111102,88.2851181001512,
88.7829761891922,89.2808342782332,89.7786923672741,90.2765504563151,90.7744085453561,
91.2722666343971,91.7701247234381,92.2679828124791,92.7658409015201,93.2636989905611,
93.761557079602,94.259415168643,94.757273257684,95.255131346725,95.752989435766,
96.250847524807,96.7487056138479,97.2465637028889,97.7444217919299,98.2422798809709,
98.7401379700119,99.2379960590529,99.7358541480939,100.233712237135,100.731570326176,
101.229428415217,101.727286504258,102.225144593299,102.72300268234,103.220860771381,
103.718718860422,104.216576949463,104.714435038504,105.212293127545,105.710151216586,
106.208009305627,106.705867394668,107.203725483709,107.70158357275,108.199441661791,
108.697299750832,109.195157839873,109.693015928914,110.190874017955,110.688732106996,
111.186590196037),.UNSPECIFIED.);
#947=FACE_BOUND('',#3007,.T.);
#948=FACE_BOUND('',#3010,.T.);
#949=FACE_BOUND('',#3014,.T.);
#950=FACE_BOUND('',#3019,.T.);
#951=FACE_BOUND('',#3037,.T.);
#952=FACE_BOUND('',#3048,.T.);
#953=FACE_BOUND('',#3050,.T.);
#954=FACE_BOUND('',#3052,.T.);
#955=FACE_BOUND('',#3055,.T.);
#956=FACE_BOUND('',#3059,.T.);
#1108=PLANE('',#17034);
#1109=PLANE('',#17038);
#1110=PLANE('',#17046);
#1111=PLANE('',#17055);
#1112=PLANE('',#17057);
#1113=PLANE('',#17062);
#1114=PLANE('',#17071);
#1115=PLANE('',#17079);
#1116=PLANE('',#17091);
#1117=PLANE('',#17092);
#1118=PLANE('',#17098);
#1119=PLANE('',#17099);
#1120=PLANE('',#17102);
#1121=PLANE('',#17107);
#1605=CYLINDRICAL_SURFACE('',#16970,20.925);
#1606=CYLINDRICAL_SURFACE('',#16972,20.925);
#1607=CYLINDRICAL_SURFACE('',#16973,20.925);
#1608=CYLINDRICAL_SURFACE('',#16974,20.925);
#1609=CYLINDRICAL_SURFACE('',#16975,20.925);
#1610=CYLINDRICAL_SURFACE('',#16976,20.925);
#1611=CYLINDRICAL_SURFACE('',#16977,20.925);
#1612=CYLINDRICAL_SURFACE('',#16978,20.925);
#1613=CYLINDRICAL_SURFACE('',#16979,20.925);
#1614=CYLINDRICAL_SURFACE('',#16980,20.925);
#1615=CYLINDRICAL_SURFACE('',#16981,20.925);
#1616=CYLINDRICAL_SURFACE('',#16982,20.925);
#1617=CYLINDRICAL_SURFACE('',#16983,20.925);
#1618=CYLINDRICAL_SURFACE('',#16984,20.925);
#1619=CYLINDRICAL_SURFACE('',#16985,20.925);
#1620=CYLINDRICAL_SURFACE('',#16986,20.925);
#1621=CYLINDRICAL_SURFACE('',#16987,20.06595);
#1622=CYLINDRICAL_SURFACE('',#16989,20.06595);
#1623=CYLINDRICAL_SURFACE('',#16990,20.06595);
#1624=CYLINDRICAL_SURFACE('',#16991,20.06595);
#1625=CYLINDRICAL_SURFACE('',#16992,20.06595);
#1626=CYLINDRICAL_SURFACE('',#16993,20.06595);
#1627=CYLINDRICAL_SURFACE('',#16994,20.06595);
#1628=CYLINDRICAL_SURFACE('',#16995,20.06595);
#1629=CYLINDRICAL_SURFACE('',#16996,20.06595);
#1630=CYLINDRICAL_SURFACE('',#16997,20.06595);
#1631=CYLINDRICAL_SURFACE('',#16998,20.06595);
#1632=CYLINDRICAL_SURFACE('',#16999,20.06595);
#1633=CYLINDRICAL_SURFACE('',#17000,20.06595);
#1634=CYLINDRICAL_SURFACE('',#17001,20.06595);
#1635=CYLINDRICAL_SURFACE('',#17002,20.06595);
#1636=CYLINDRICAL_SURFACE('',#17003,16.425);
#1637=CYLINDRICAL_SURFACE('',#17005,16.425);
#1638=CYLINDRICAL_SURFACE('',#17006,16.425);
#1639=CYLINDRICAL_SURFACE('',#17007,16.425);
#1640=CYLINDRICAL_SURFACE('',#17008,16.425);
#1641=CYLINDRICAL_SURFACE('',#17009,16.425);
#1642=CYLINDRICAL_SURFACE('',#17010,16.425);
#1643=CYLINDRICAL_SURFACE('',#17011,16.425);
#1644=CYLINDRICAL_SURFACE('',#17012,16.425);
#1645=CYLINDRICAL_SURFACE('',#17013,16.425);
#1646=CYLINDRICAL_SURFACE('',#17014,16.425);
#1647=CYLINDRICAL_SURFACE('',#17016,15.56595);
#1648=CYLINDRICAL_SURFACE('',#17018,15.56595);
#1649=CYLINDRICAL_SURFACE('',#17019,15.56595);
#1650=CYLINDRICAL_SURFACE('',#17020,15.56595);
#1651=CYLINDRICAL_SURFACE('',#17021,15.56595);
#1652=CYLINDRICAL_SURFACE('',#17022,15.56595);
#1653=CYLINDRICAL_SURFACE('',#17023,15.56595);
#1654=CYLINDRICAL_SURFACE('',#17024,15.56595);
#1655=CYLINDRICAL_SURFACE('',#17025,15.56595);
#1656=CYLINDRICAL_SURFACE('',#17026,15.56595);
#1657=CYLINDRICAL_SURFACE('',#17031,4.);
#1658=CYLINDRICAL_SURFACE('',#17059,15.56595);
#1659=CYLINDRICAL_SURFACE('',#17060,16.425);
#1660=CYLINDRICAL_SURFACE('',#17066,20.06595);
#1661=CYLINDRICAL_SURFACE('',#17067,0.6);
#1662=CYLINDRICAL_SURFACE('',#17068,6.99999999999999);
#1663=CYLINDRICAL_SURFACE('',#17073,0.6);
#1664=CYLINDRICAL_SURFACE('',#17074,0.600000000000005);
#1665=CYLINDRICAL_SURFACE('',#17075,0.600000000000005);
#1666=CYLINDRICAL_SURFACE('',#17081,5.05000000000001);
#1667=CYLINDRICAL_SURFACE('',#17085,4.01);
#1668=CYLINDRICAL_SURFACE('',#17089,13.);
#1669=CYLINDRICAL_SURFACE('',#17090,10.);
#1670=CYLINDRICAL_SURFACE('',#17093,3.05);
#1671=CYLINDRICAL_SURFACE('',#17096,26.);
#1672=CYLINDRICAL_SURFACE('',#17100,18.);
#1673=CYLINDRICAL_SURFACE('',#17105,20.925);
#1970=FACE_OUTER_BOUND('',#2952,.T.);
#1971=FACE_OUTER_BOUND('',#2953,.T.);
#1972=FACE_OUTER_BOUND('',#2954,.T.);
#1973=FACE_OUTER_BOUND('',#2955,.T.);
#1974=FACE_OUTER_BOUND('',#2956,.T.);
#1975=FACE_OUTER_BOUND('',#2957,.T.);
#1976=FACE_OUTER_BOUND('',#2958,.T.);
#1977=FACE_OUTER_BOUND('',#2959,.T.);
#1978=FACE_OUTER_BOUND('',#2960,.T.);
#1979=FACE_OUTER_BOUND('',#2961,.T.);
#1980=FACE_OUTER_BOUND('',#2962,.T.);
#1981=FACE_OUTER_BOUND('',#2963,.T.);
#1982=FACE_OUTER_BOUND('',#2964,.T.);
#1983=FACE_OUTER_BOUND('',#2965,.T.);
#1984=FACE_OUTER_BOUND('',#2966,.T.);
#1985=FACE_OUTER_BOUND('',#2967,.T.);
#1986=FACE_OUTER_BOUND('',#2968,.T.);
#1987=FACE_OUTER_BOUND('',#2969,.T.);
#1988=FACE_OUTER_BOUND('',#2970,.T.);
#1989=FACE_OUTER_BOUND('',#2971,.T.);
#1990=FACE_OUTER_BOUND('',#2972,.T.);
#1991=FACE_OUTER_BOUND('',#2973,.T.);
#1992=FACE_OUTER_BOUND('',#2974,.T.);
#1993=FACE_OUTER_BOUND('',#2975,.T.);
#1994=FACE_OUTER_BOUND('',#2976,.T.);
#1995=FACE_OUTER_BOUND('',#2977,.T.);
#1996=FACE_OUTER_BOUND('',#2978,.T.);
#1997=FACE_OUTER_BOUND('',#2979,.T.);
#1998=FACE_OUTER_BOUND('',#2980,.T.);
#1999=FACE_OUTER_BOUND('',#2981,.T.);
#2000=FACE_OUTER_BOUND('',#2982,.T.);
#2001=FACE_OUTER_BOUND('',#2983,.T.);
#2002=FACE_OUTER_BOUND('',#2984,.T.);
#2003=FACE_OUTER_BOUND('',#2985,.T.);
#2004=FACE_OUTER_BOUND('',#2986,.T.);
#2005=FACE_OUTER_BOUND('',#2987,.T.);
#2006=FACE_OUTER_BOUND('',#2988,.T.);
#2007=FACE_OUTER_BOUND('',#2989,.T.);
#2008=FACE_OUTER_BOUND('',#2990,.T.);
#2009=FACE_OUTER_BOUND('',#2991,.T.);
#2010=FACE_OUTER_BOUND('',#2992,.T.);
#2011=FACE_OUTER_BOUND('',#2993,.T.);
#2012=FACE_OUTER_BOUND('',#2994,.T.);
#2013=FACE_OUTER_BOUND('',#2995,.T.);
#2014=FACE_OUTER_BOUND('',#2996,.T.);
#2015=FACE_OUTER_BOUND('',#2997,.T.);
#2016=FACE_OUTER_BOUND('',#2998,.T.);
#2017=FACE_OUTER_BOUND('',#2999,.T.);
#2018=FACE_OUTER_BOUND('',#3000,.T.);
#2019=FACE_OUTER_BOUND('',#3001,.T.);
#2020=FACE_OUTER_BOUND('',#3002,.T.);
#2021=FACE_OUTER_BOUND('',#3003,.T.);
#2022=FACE_OUTER_BOUND('',#3004,.T.);
#2023=FACE_OUTER_BOUND('',#3005,.T.);
#2024=FACE_OUTER_BOUND('',#3006,.T.);
#2025=FACE_OUTER_BOUND('',#3008,.T.);
#2026=FACE_OUTER_BOUND('',#3009,.T.);
#2027=FACE_OUTER_BOUND('',#3011,.T.);
#2028=FACE_OUTER_BOUND('',#3012,.T.);
#2029=FACE_OUTER_BOUND('',#3013,.T.);
#2030=FACE_OUTER_BOUND('',#3015,.T.);
#2031=FACE_OUTER_BOUND('',#3016,.T.);
#2032=FACE_OUTER_BOUND('',#3017,.T.);
#2033=FACE_OUTER_BOUND('',#3018,.T.);
#2034=FACE_OUTER_BOUND('',#3020,.T.);
#2035=FACE_OUTER_BOUND('',#3021,.T.);
#2036=FACE_OUTER_BOUND('',#3022,.T.);
#2037=FACE_OUTER_BOUND('',#3023,.T.);
#2038=FACE_OUTER_BOUND('',#3024,.T.);
#2039=FACE_OUTER_BOUND('',#3025,.T.);
#2040=FACE_OUTER_BOUND('',#3026,.T.);
#2041=FACE_OUTER_BOUND('',#3027,.T.);
#2042=FACE_OUTER_BOUND('',#3028,.T.);
#2043=FACE_OUTER_BOUND('',#3029,.T.);
#2044=FACE_OUTER_BOUND('',#3030,.T.);
#2045=FACE_OUTER_BOUND('',#3031,.T.);
#2046=FACE_OUTER_BOUND('',#3032,.T.);
#2047=FACE_OUTER_BOUND('',#3033,.T.);
#2048=FACE_OUTER_BOUND('',#3034,.T.);
#2049=FACE_OUTER_BOUND('',#3035,.T.);
#2050=FACE_OUTER_BOUND('',#3036,.T.);
#2051=FACE_OUTER_BOUND('',#3038,.T.);
#2052=FACE_OUTER_BOUND('',#3039,.T.);
#2053=FACE_OUTER_BOUND('',#3040,.T.);
#2054=FACE_OUTER_BOUND('',#3041,.T.);
#2055=FACE_OUTER_BOUND('',#3042,.T.);
#2056=FACE_OUTER_BOUND('',#3043,.T.);
#2057=FACE_OUTER_BOUND('',#3044,.T.);
#2058=FACE_OUTER_BOUND('',#3045,.T.);
#2059=FACE_OUTER_BOUND('',#3046,.T.);
#2060=FACE_OUTER_BOUND('',#3047,.T.);
#2061=FACE_OUTER_BOUND('',#3049,.T.);
#2062=FACE_OUTER_BOUND('',#3051,.T.);
#2063=FACE_OUTER_BOUND('',#3053,.T.);
#2064=FACE_OUTER_BOUND('',#3054,.T.);
#2065=FACE_OUTER_BOUND('',#3056,.T.);
#2066=FACE_OUTER_BOUND('',#3057,.T.);
#2067=FACE_OUTER_BOUND('',#3058,.T.);
#2068=FACE_OUTER_BOUND('',#3060,.T.);
#2069=FACE_OUTER_BOUND('',#3061,.T.);
#2952=EDGE_LOOP('',(#11550,#11551,#11552,#11553));
#2953=EDGE_LOOP('',(#11554,#11555,#11556,#11557));
#2954=EDGE_LOOP('',(#11558,#11559,#11560,#11561));
#2955=EDGE_LOOP('',(#11562,#11563,#11564,#11565));
#2956=EDGE_LOOP('',(#11566,#11567,#11568,#11569));
#2957=EDGE_LOOP('',(#11570,#11571,#11572,#11573));
#2958=EDGE_LOOP('',(#11574,#11575,#11576,#11577));
#2959=EDGE_LOOP('',(#11578,#11579,#11580,#11581));
#2960=EDGE_LOOP('',(#11582,#11583,#11584,#11585));
#2961=EDGE_LOOP('',(#11586,#11587,#11588,#11589));
#2962=EDGE_LOOP('',(#11590,#11591,#11592,#11593));
#2963=EDGE_LOOP('',(#11594,#11595,#11596,#11597));
#2964=EDGE_LOOP('',(#11598,#11599,#11600,#11601));
#2965=EDGE_LOOP('',(#11602,#11603,#11604,#11605));
#2966=EDGE_LOOP('',(#11606,#11607,#11608,#11609));
#2967=EDGE_LOOP('',(#11610,#11611,#11612,#11613));
#2968=EDGE_LOOP('',(#11614,#11615,#11616,#11617));
#2969=EDGE_LOOP('',(#11618,#11619,#11620,#11621));
#2970=EDGE_LOOP('',(#11622,#11623,#11624,#11625));
#2971=EDGE_LOOP('',(#11626,#11627,#11628,#11629));
#2972=EDGE_LOOP('',(#11630,#11631,#11632,#11633));
#2973=EDGE_LOOP('',(#11634,#11635,#11636,#11637));
#2974=EDGE_LOOP('',(#11638,#11639,#11640,#11641));
#2975=EDGE_LOOP('',(#11642,#11643,#11644,#11645));
#2976=EDGE_LOOP('',(#11646,#11647,#11648,#11649));
#2977=EDGE_LOOP('',(#11650,#11651,#11652,#11653));
#2978=EDGE_LOOP('',(#11654,#11655,#11656,#11657));
#2979=EDGE_LOOP('',(#11658,#11659,#11660,#11661));
#2980=EDGE_LOOP('',(#11662,#11663,#11664,#11665));
#2981=EDGE_LOOP('',(#11666,#11667,#11668,#11669));
#2982=EDGE_LOOP('',(#11670,#11671,#11672,#11673));
#2983=EDGE_LOOP('',(#11674,#11675,#11676,#11677));
#2984=EDGE_LOOP('',(#11678,#11679,#11680,#11681));
#2985=EDGE_LOOP('',(#11682,#11683,#11684,#11685));
#2986=EDGE_LOOP('',(#11686,#11687,#11688,#11689));
#2987=EDGE_LOOP('',(#11690,#11691,#11692,#11693));
#2988=EDGE_LOOP('',(#11694,#11695,#11696,#11697));
#2989=EDGE_LOOP('',(#11698,#11699,#11700,#11701));
#2990=EDGE_LOOP('',(#11702,#11703,#11704,#11705));
#2991=EDGE_LOOP('',(#11706,#11707,#11708,#11709));
#2992=EDGE_LOOP('',(#11710,#11711,#11712,#11713));
#2993=EDGE_LOOP('',(#11714,#11715,#11716,#11717,#11718));
#2994=EDGE_LOOP('',(#11719,#11720,#11721,#11722));
#2995=EDGE_LOOP('',(#11723,#11724,#11725,#11726));
#2996=EDGE_LOOP('',(#11727,#11728,#11729,#11730));
#2997=EDGE_LOOP('',(#11731,#11732,#11733,#11734));
#2998=EDGE_LOOP('',(#11735,#11736,#11737,#11738));
#2999=EDGE_LOOP('',(#11739,#11740,#11741,#11742));
#3000=EDGE_LOOP('',(#11743,#11744,#11745,#11746));
#3001=EDGE_LOOP('',(#11747,#11748,#11749,#11750));
#3002=EDGE_LOOP('',(#11751,#11752,#11753,#11754));
#3003=EDGE_LOOP('',(#11755,#11756,#11757,#11758));
#3004=EDGE_LOOP('',(#11759,#11760,#11761,#11762,#11763));
#3005=EDGE_LOOP('',(#11764,#11765,#11766,#11767,#11768,#11769));
#3006=EDGE_LOOP('',(#11770));
#3007=EDGE_LOOP('',(#11771));
#3008=EDGE_LOOP('',(#11772,#11773,#11774,#11775,#11776));
#3009=EDGE_LOOP('',(#11777));
#3010=EDGE_LOOP('',(#11778));
#3011=EDGE_LOOP('',(#11779,#11780,#11781,#11782,#11783));
#3012=EDGE_LOOP('',(#11784,#11785,#11786,#11787,#11788));
#3013=EDGE_LOOP('',(#11789));
#3014=EDGE_LOOP('',(#11790,#11791,#11792,#11793));
#3015=EDGE_LOOP('',(#11794,#11795,#11796,#11797,#11798,#11799));
#3016=EDGE_LOOP('',(#11800,#11801,#11802,#11803));
#3017=EDGE_LOOP('',(#11804,#11805,#11806,#11807));
#3018=EDGE_LOOP('',(#11808));
#3019=EDGE_LOOP('',(#11809));
#3020=EDGE_LOOP('',(#11810,#11811,#11812,#11813));
#3021=EDGE_LOOP('',(#11814,#11815,#11816,#11817,#11818,#11819,#11820,#11821,
#11822,#11823,#11824,#11825,#11826,#11827,#11828,#11829,#11830,#11831,#11832,
#11833,#11834,#11835,#11836,#11837,#11838));
#3022=EDGE_LOOP('',(#11839,#11840,#11841,#11842));
#3023=EDGE_LOOP('',(#11843,#11844,#11845,#11846,#11847,#11848,#11849,#11850,
#11851,#11852,#11853,#11854,#11855,#11856,#11857,#11858,#11859,#11860,#11861,
#11862,#11863,#11864,#11865,#11866));
#3024=EDGE_LOOP('',(#11867,#11868,#11869));
#3025=EDGE_LOOP('',(#11870,#11871,#11872,#11873,#11874,#11875,#11876,#11877,
#11878,#11879,#11880,#11881,#11882,#11883,#11884,#11885,#11886,#11887,#11888,
#11889,#11890,#11891,#11892,#11893,#11894,#11895,#11896,#11897,#11898,#11899,
#11900,#11901,#11902,#11903,#11904));
#3026=EDGE_LOOP('',(#11905,#11906,#11907,#11908,#11909));
#3027=EDGE_LOOP('',(#11910,#11911,#11912,#11913));
#3028=EDGE_LOOP('',(#11914,#11915,#11916,#11917,#11918,#11919,#11920,#11921,
#11922,#11923,#11924,#11925,#11926,#11927,#11928,#11929,#11930,#11931,#11932,
#11933,#11934,#11935,#11936,#11937,#11938,#11939,#11940,#11941,#11942,#11943,
#11944,#11945,#11946,#11947,#11948));
#3029=EDGE_LOOP('',(#11949,#11950,#11951,#11952));
#3030=EDGE_LOOP('',(#11953,#11954,#11955,#11956,#11957,#11958,#11959,#11960,
#11961,#11962,#11963));
#3031=EDGE_LOOP('',(#11964,#11965,#11966,#11967));
#3032=EDGE_LOOP('',(#11968,#11969,#11970,#11971));
#3033=EDGE_LOOP('',(#11972,#11973,#11974,#11975));
#3034=EDGE_LOOP('',(#11976,#11977,#11978,#11979));
#3035=EDGE_LOOP('',(#11980,#11981,#11982,#11983));
#3036=EDGE_LOOP('',(#11984));
#3037=EDGE_LOOP('',(#11985));
#3038=EDGE_LOOP('',(#11986,#11987,#11988,#11989));
#3039=EDGE_LOOP('',(#11990,#11991,#11992,#11993));
#3040=EDGE_LOOP('',(#11994,#11995,#11996,#11997));
#3041=EDGE_LOOP('',(#11998,#11999,#12000,#12001));
#3042=EDGE_LOOP('',(#12002,#12003,#12004,#12005,#12006));
#3043=EDGE_LOOP('',(#12007,#12008,#12009,#12010,#12011,#12012));
#3044=EDGE_LOOP('',(#12013));
#3045=EDGE_LOOP('',(#12014));
#3046=EDGE_LOOP('',(#12015,#12016,#12017,#12018));
#3047=EDGE_LOOP('',(#12019,#12020,#12021,#12022,#12023,#12024));
#3048=EDGE_LOOP('',(#12025,#12026,#12027,#12028,#12029,#12030,#12031,#12032));
#3049=EDGE_LOOP('',(#12033,#12034,#12035,#12036));
#3050=EDGE_LOOP('',(#12037));
#3051=EDGE_LOOP('',(#12038,#12039,#12040,#12041));
#3052=EDGE_LOOP('',(#12042));
#3053=EDGE_LOOP('',(#12043,#12044,#12045,#12046));
#3054=EDGE_LOOP('',(#12047));
#3055=EDGE_LOOP('',(#12048));
#3056=EDGE_LOOP('',(#12049,#12050,#12051,#12052,#12053,#12054));
#3057=EDGE_LOOP('',(#12055,#12056,#12057,#12058));
#3058=EDGE_LOOP('',(#12059));
#3059=EDGE_LOOP('',(#12060,#12061,#12062,#12063));
#3060=EDGE_LOOP('',(#12064,#12065,#12066,#12067));
#3061=EDGE_LOOP('',(#12068,#12069,#12070,#12071,#12072,#12073));
#4073=LINE('',#23913,#5384);
#4074=LINE('',#23946,#5385);
#4075=LINE('',#24030,#5386);
#4076=LINE('',#24120,#5387);
#4077=LINE('',#24210,#5388);
#4078=LINE('',#24294,#5389);
#4079=LINE('',#24384,#5390);
#4080=LINE('',#24468,#5391);
#4081=LINE('',#24558,#5392);
#4082=LINE('',#24648,#5393);
#4083=LINE('',#24732,#5394);
#4084=LINE('',#24822,#5395);
#4085=LINE('',#24912,#5396);
#4086=LINE('',#24996,#5397);
#4087=LINE('',#25086,#5398);
#4088=LINE('',#25170,#5399);
#4089=LINE('',#25260,#5400);
#4090=LINE('',#25294,#5401);
#4091=LINE('',#25331,#5402);
#4092=LINE('',#25368,#5403);
#4093=LINE('',#25405,#5404);
#4094=LINE('',#25442,#5405);
#4095=LINE('',#25480,#5406);
#4096=LINE('',#25517,#5407);
#4097=LINE('',#25554,#5408);
#4098=LINE('',#25592,#5409);
#4099=LINE('',#25629,#5410);
#4100=LINE('',#25666,#5411);
#4101=LINE('',#25703,#5412);
#4102=LINE('',#25740,#5413);
#4103=LINE('',#25778,#5414);
#4104=LINE('',#25815,#5415);
#4105=LINE('',#25848,#5416);
#4106=LINE('',#25938,#5417);
#4107=LINE('',#26022,#5418);
#4108=LINE('',#26112,#5419);
#4109=LINE('',#26202,#5420);
#4110=LINE('',#26292,#5421);
#4111=LINE('',#26376,#5422);
#4112=LINE('',#26466,#5423);
#4113=LINE('',#26556,#5424);
#4114=LINE('',#26643,#5425);
#4115=LINE('',#26726,#5426);
#4116=LINE('',#26751,#5427);
#4117=LINE('',#26789,#5428);
#4118=LINE('',#26826,#5429);
#4119=LINE('',#26864,#5430);
#4120=LINE('',#26901,#5431);
#4121=LINE('',#26938,#5432);
#4122=LINE('',#26976,#5433);
#4123=LINE('',#27014,#5434);
#4124=LINE('',#27051,#5435);
#4125=LINE('',#27089,#5436);
#4126=LINE('',#27098,#5437);
#4127=LINE('',#27104,#5438);
#4128=LINE('',#27113,#5439);
#4129=LINE('',#27119,#5440);
#4130=LINE('',#27407,#5441);
#4131=LINE('',#27426,#5442);
#4132=LINE('',#27429,#5443);
#4133=LINE('',#31073,#5444);
#4134=LINE('',#31085,#5445);
#4135=LINE('',#31088,#5446);
#4136=LINE('',#31141,#5447);
#4137=LINE('',#31154,#5448);
#4138=LINE('',#31168,#5449);
#4139=LINE('',#31169,#5450);
#4140=LINE('',#31172,#5451);
#4141=LINE('',#31184,#5452);
#4142=LINE('',#31189,#5453);
#4143=LINE('',#31196,#5454);
#4144=LINE('',#31200,#5455);
#4145=LINE('',#31204,#5456);
#4146=LINE('',#31208,#5457);
#4147=LINE('',#31212,#5458);
#4148=LINE('',#31304,#5459);
#4149=LINE('',#31308,#5460);
#4150=LINE('',#31310,#5461);
#4151=LINE('',#31311,#5462);
#4152=LINE('',#31316,#5463);
#4153=LINE('',#31322,#5464);
#4154=LINE('',#31329,#5465);
#4155=LINE('',#31331,#5466);
#5384=VECTOR('',#18736,21.);
#5385=VECTOR('',#18741,21.);
#5386=VECTOR('',#18744,21.);
#5387=VECTOR('',#18747,21.);
#5388=VECTOR('',#18750,21.);
#5389=VECTOR('',#18753,21.);
#5390=VECTOR('',#18756,21.);
#5391=VECTOR('',#18759,21.);
#5392=VECTOR('',#18762,21.);
#5393=VECTOR('',#18765,21.);
#5394=VECTOR('',#18768,21.);
#5395=VECTOR('',#18771,21.);
#5396=VECTOR('',#18774,21.);
#5397=VECTOR('',#18777,21.);
#5398=VECTOR('',#18780,21.);
#5399=VECTOR('',#18783,21.);
#5400=VECTOR('',#18786,20.06595);
#5401=VECTOR('',#18791,20.06595);
#5402=VECTOR('',#18794,20.06595);
#5403=VECTOR('',#18797,20.06595);
#5404=VECTOR('',#18800,20.06595);
#5405=VECTOR('',#18803,20.06595);
#5406=VECTOR('',#18806,20.06595);
#5407=VECTOR('',#18809,20.06595);
#5408=VECTOR('',#18812,20.06595);
#5409=VECTOR('',#18815,20.06595);
#5410=VECTOR('',#18818,20.06595);
#5411=VECTOR('',#18821,20.06595);
#5412=VECTOR('',#18824,20.06595);
#5413=VECTOR('',#18827,20.06595);
#5414=VECTOR('',#18830,20.06595);
#5415=VECTOR('',#18833,16.5);
#5416=VECTOR('',#18838,16.5);
#5417=VECTOR('',#18841,16.5);
#5418=VECTOR('',#18844,16.5);
#5419=VECTOR('',#18847,16.5);
#5420=VECTOR('',#18850,16.5);
#5421=VECTOR('',#18853,16.5);
#5422=VECTOR('',#18856,16.5);
#5423=VECTOR('',#18859,16.5);
#5424=VECTOR('',#18862,16.5);
#5425=VECTOR('',#18865,16.5);
#5426=VECTOR('',#18870,15.56595);
#5427=VECTOR('',#18875,15.56595);
#5428=VECTOR('',#18878,15.56595);
#5429=VECTOR('',#18881,15.56595);
#5430=VECTOR('',#18884,15.56595);
#5431=VECTOR('',#18887,15.56595);
#5432=VECTOR('',#18890,15.56595);
#5433=VECTOR('',#18893,15.56595);
#5434=VECTOR('',#18896,15.56595);
#5435=VECTOR('',#18899,15.56595);
#5436=VECTOR('',#18904,4.25);
#5437=VECTOR('',#18915,4.);
#5438=VECTOR('',#18922,4.25);
#5439=VECTOR('',#18933,24.9267766952966);
#5440=VECTOR('',#18940,25.5);
#5441=VECTOR('',#18951,9.82322330470337);
#5442=VECTOR('',#18958,9.6);
#5443=VECTOR('',#18961,9.12677669529663);
#5444=VECTOR('',#18990,10.);
#5445=VECTOR('',#18991,10.);
#5446=VECTOR('',#18994,10.);
#5447=VECTOR('',#19003,10.);
#5448=VECTOR('',#19006,10.);
#5449=VECTOR('',#19009,0.6);
#5450=VECTOR('',#19010,10.);
#5451=VECTOR('',#19013,0.6);
#5452=VECTOR('',#19014,10.);
#5453=VECTOR('',#19019,5.25);
#5454=VECTOR('',#19028,5.05000000000001);
#5455=VECTOR('',#19033,4.20999999999999);
#5456=VECTOR('',#19038,4.01);
#5457=VECTOR('',#19043,12.6);
#5458=VECTOR('',#19048,13.);
#5459=VECTOR('',#19059,3.05);
#5460=VECTOR('',#19064,26.);
#5461=VECTOR('',#19067,10.);
#5462=VECTOR('',#19068,10.);
#5463=VECTOR('',#19075,18.);
#5464=VECTOR('',#19084,20.6);
#5465=VECTOR('',#19095,25.5);
#5466=VECTOR('',#19098,16.1);
#6599=CIRCLE('',#16971,20.925);
#6600=CIRCLE('',#16988,20.06595);
#6601=CIRCLE('',#17004,16.425);
#6602=CIRCLE('',#17015,16.425);
#6603=CIRCLE('',#17017,15.56595);
#6604=CIRCLE('',#17028,4.5);
#6605=CIRCLE('',#17029,4.);
#6606=CIRCLE('',#17030,4.);
#6607=CIRCLE('',#17032,4.);
#6608=CIRCLE('',#17033,4.);
#6609=CIRCLE('',#17035,18.);
#6610=CIRCLE('',#17037,4.5);
#6611=CIRCLE('',#17039,15.7);
#6612=CIRCLE('',#17041,24.5);
#6613=CIRCLE('',#17042,25.3535533905933);
#6614=CIRCLE('',#17043,25.3535533905933);
#6615=CIRCLE('',#17045,26.);
#6616=CIRCLE('',#17047,15.56595);
#6617=CIRCLE('',#17049,9.64644660940673);
#6618=CIRCLE('',#17050,10.);
#6619=CIRCLE('',#17052,9.55355339059327);
#6620=CIRCLE('',#17054,8.7);
#6621=CIRCLE('',#17056,4.40999999999999);
#6622=CIRCLE('',#17058,16.425);
#6623=CIRCLE('',#17061,16.425);
#6624=CIRCLE('',#17063,20.925);
#6625=CIRCLE('',#17064,20.925);
#6626=CIRCLE('',#17065,20.06595);
#6627=CIRCLE('',#17069,6.99999999999999);
#6628=CIRCLE('',#17070,6.99999999999999);
#6629=CIRCLE('',#17072,26.);
#6630=CIRCLE('',#17077,5.45);
#6631=CIRCLE('',#17078,5.05000000000001);
#6632=CIRCLE('',#17080,12.2);
#6633=CIRCLE('',#17082,5.05000000000001);
#6634=CIRCLE('',#17084,4.01);
#6635=CIRCLE('',#17086,4.01);
#6636=CIRCLE('',#17088,13.);
#6637=CIRCLE('',#17094,3.05);
#6638=CIRCLE('',#17095,3.05);
#6639=CIRCLE('',#17097,26.);
#6640=CIRCLE('',#17101,18.);
#6641=CIRCLE('',#17103,20.2);
#6642=CIRCLE('',#17106,20.925);
#6643=CIRCLE('',#17108,25.);
#7190=VERTEX_POINT('',#23911);
#7191=VERTEX_POINT('',#23912);
#7192=VERTEX_POINT('',#23914);
#7193=VERTEX_POINT('',#23931);
#7194=VERTEX_POINT('',#23944);
#7195=VERTEX_POINT('',#23945);
#7196=VERTEX_POINT('',#24028);
#7197=VERTEX_POINT('',#24029);
#7198=VERTEX_POINT('',#24118);
#7199=VERTEX_POINT('',#24119);
#7200=VERTEX_POINT('',#24208);
#7201=VERTEX_POINT('',#24209);
#7202=VERTEX_POINT('',#24292);
#7203=VERTEX_POINT('',#24293);
#7204=VERTEX_POINT('',#24382);
#7205=VERTEX_POINT('',#24383);
#7206=VERTEX_POINT('',#24466);
#7207=VERTEX_POINT('',#24467);
#7208=VERTEX_POINT('',#24556);
#7209=VERTEX_POINT('',#24557);
#7210=VERTEX_POINT('',#24646);
#7211=VERTEX_POINT('',#24647);
#7212=VERTEX_POINT('',#24730);
#7213=VERTEX_POINT('',#24731);
#7214=VERTEX_POINT('',#24820);
#7215=VERTEX_POINT('',#24821);
#7216=VERTEX_POINT('',#24910);
#7217=VERTEX_POINT('',#24911);
#7218=VERTEX_POINT('',#24994);
#7219=VERTEX_POINT('',#24995);
#7220=VERTEX_POINT('',#25084);
#7221=VERTEX_POINT('',#25085);
#7222=VERTEX_POINT('',#25168);
#7223=VERTEX_POINT('',#25169);
#7224=VERTEX_POINT('',#25258);
#7225=VERTEX_POINT('',#25259);
#7226=VERTEX_POINT('',#25261);
#7227=VERTEX_POINT('',#25277);
#7228=VERTEX_POINT('',#25292);
#7229=VERTEX_POINT('',#25293);
#7230=VERTEX_POINT('',#25329);
#7231=VERTEX_POINT('',#25330);
#7232=VERTEX_POINT('',#25366);
#7233=VERTEX_POINT('',#25367);
#7234=VERTEX_POINT('',#25403);
#7235=VERTEX_POINT('',#25404);
#7236=VERTEX_POINT('',#25440);
#7237=VERTEX_POINT('',#25441);
#7238=VERTEX_POINT('',#25478);
#7239=VERTEX_POINT('',#25479);
#7240=VERTEX_POINT('',#25515);
#7241=VERTEX_POINT('',#25516);
#7242=VERTEX_POINT('',#25552);
#7243=VERTEX_POINT('',#25553);
#7244=VERTEX_POINT('',#25590);
#7245=VERTEX_POINT('',#25591);
#7246=VERTEX_POINT('',#25627);
#7247=VERTEX_POINT('',#25628);
#7248=VERTEX_POINT('',#25664);
#7249=VERTEX_POINT('',#25665);
#7250=VERTEX_POINT('',#25701);
#7251=VERTEX_POINT('',#25702);
#7252=VERTEX_POINT('',#25738);
#7253=VERTEX_POINT('',#25739);
#7254=VERTEX_POINT('',#25776);
#7255=VERTEX_POINT('',#25777);
#7256=VERTEX_POINT('',#25813);
#7257=VERTEX_POINT('',#25814);
#7258=VERTEX_POINT('',#25816);
#7259=VERTEX_POINT('',#25833);
#7260=VERTEX_POINT('',#25846);
#7261=VERTEX_POINT('',#25847);
#7262=VERTEX_POINT('',#25936);
#7263=VERTEX_POINT('',#25937);
#7264=VERTEX_POINT('',#26020);
#7265=VERTEX_POINT('',#26021);
#7266=VERTEX_POINT('',#26110);
#7267=VERTEX_POINT('',#26111);
#7268=VERTEX_POINT('',#26200);
#7269=VERTEX_POINT('',#26201);
#7270=VERTEX_POINT('',#26290);
#7271=VERTEX_POINT('',#26291);
#7272=VERTEX_POINT('',#26374);
#7273=VERTEX_POINT('',#26375);
#7274=VERTEX_POINT('',#26464);
#7275=VERTEX_POINT('',#26465);
#7276=VERTEX_POINT('',#26554);
#7277=VERTEX_POINT('',#26555);
#7278=VERTEX_POINT('',#26641);
#7279=VERTEX_POINT('',#26642);
#7280=VERTEX_POINT('',#26644);
#7281=VERTEX_POINT('',#26724);
#7282=VERTEX_POINT('',#26725);
#7283=VERTEX_POINT('',#26727);
#7284=VERTEX_POINT('',#26738);
#7285=VERTEX_POINT('',#26749);
#7286=VERTEX_POINT('',#26750);
#7287=VERTEX_POINT('',#26787);
#7288=VERTEX_POINT('',#26788);
#7289=VERTEX_POINT('',#26824);
#7290=VERTEX_POINT('',#26825);
#7291=VERTEX_POINT('',#26862);
#7292=VERTEX_POINT('',#26863);
#7293=VERTEX_POINT('',#26899);
#7294=VERTEX_POINT('',#26900);
#7295=VERTEX_POINT('',#26936);
#7296=VERTEX_POINT('',#26937);
#7297=VERTEX_POINT('',#26974);
#7298=VERTEX_POINT('',#26975);
#7299=VERTEX_POINT('',#27012);
#7300=VERTEX_POINT('',#27013);
#7301=VERTEX_POINT('',#27049);
#7302=VERTEX_POINT('',#27050);
#7303=VERTEX_POINT('',#27086);
#7304=VERTEX_POINT('',#27088);
#7305=VERTEX_POINT('',#27090);
#7306=VERTEX_POINT('',#27094);
#7307=VERTEX_POINT('',#27095);
#7308=VERTEX_POINT('',#27100);
#7309=VERTEX_POINT('',#27103);
#7310=VERTEX_POINT('',#27107);
#7311=VERTEX_POINT('',#27110);
#7312=VERTEX_POINT('',#27112);
#7313=VERTEX_POINT('',#27114);
#7314=VERTEX_POINT('',#27118);
#7315=VERTEX_POINT('',#27122);
#7316=VERTEX_POINT('',#27262);
#7317=VERTEX_POINT('',#27404);
#7318=VERTEX_POINT('',#27406);
#7319=VERTEX_POINT('',#27408);
#7320=VERTEX_POINT('',#27415);
#7321=VERTEX_POINT('',#27424);
#7322=VERTEX_POINT('',#27428);
#7323=VERTEX_POINT('',#27432);
#7324=VERTEX_POINT('',#27574);
#7325=VERTEX_POINT('',#29657);
#7326=VERTEX_POINT('',#29810);
#7327=VERTEX_POINT('',#29956);
#7328=VERTEX_POINT('',#29959);
#7329=VERTEX_POINT('',#30922);
#7330=VERTEX_POINT('',#31064);
#7331=VERTEX_POINT('',#31065);
#7332=VERTEX_POINT('',#31072);
#7333=VERTEX_POINT('',#31074);
#7334=VERTEX_POINT('',#31087);
#7335=VERTEX_POINT('',#31089);
#7336=VERTEX_POINT('',#31096);
#7337=VERTEX_POINT('',#31098);
#7338=VERTEX_POINT('',#31117);
#7339=VERTEX_POINT('',#31126);
#7340=VERTEX_POINT('',#31139);
#7341=VERTEX_POINT('',#31143);
#7342=VERTEX_POINT('',#31156);
#7343=VERTEX_POINT('',#31157);
#7344=VERTEX_POINT('',#31171);
#7345=VERTEX_POINT('',#31173);
#7346=VERTEX_POINT('',#31186);
#7347=VERTEX_POINT('',#31188);
#7348=VERTEX_POINT('',#31192);
#7349=VERTEX_POINT('',#31195);
#7350=VERTEX_POINT('',#31199);
#7351=VERTEX_POINT('',#31203);
#7352=VERTEX_POINT('',#31207);
#7353=VERTEX_POINT('',#31211);
#7354=VERTEX_POINT('',#31301);
#7355=VERTEX_POINT('',#31303);
#7356=VERTEX_POINT('',#31307);
#7357=VERTEX_POINT('',#31315);
#7358=VERTEX_POINT('',#31319);
#7359=VERTEX_POINT('',#31326);
#8838=EDGE_CURVE('',#7190,#7191,#4073,.T.);
#8839=EDGE_CURVE('',#7190,#7192,#350,.T.);
#8840=EDGE_CURVE('',#7192,#7193,#6599,.T.);
#8841=EDGE_CURVE('',#7193,#7191,#351,.T.);
#8842=EDGE_CURVE('',#7194,#7195,#4074,.T.);
#8843=EDGE_CURVE('',#7194,#7190,#352,.T.);
#8844=EDGE_CURVE('',#7191,#7195,#353,.T.);
#8845=EDGE_CURVE('',#7196,#7197,#4075,.T.);
#8846=EDGE_CURVE('',#7196,#7194,#354,.T.);
#8847=EDGE_CURVE('',#7195,#7197,#355,.T.);
#8848=EDGE_CURVE('',#7198,#7199,#4076,.T.);
#8849=EDGE_CURVE('',#7198,#7196,#356,.T.);
#8850=EDGE_CURVE('',#7197,#7199,#357,.T.);
#8851=EDGE_CURVE('',#7200,#7201,#4077,.T.);
#8852=EDGE_CURVE('',#7200,#7198,#358,.T.);
#8853=EDGE_CURVE('',#7199,#7201,#359,.T.);
#8854=EDGE_CURVE('',#7202,#7203,#4078,.T.);
#8855=EDGE_CURVE('',#7202,#7200,#360,.T.);
#8856=EDGE_CURVE('',#7201,#7203,#361,.T.);
#8857=EDGE_CURVE('',#7204,#7205,#4079,.T.);
#8858=EDGE_CURVE('',#7204,#7202,#362,.T.);
#8859=EDGE_CURVE('',#7203,#7205,#363,.T.);
#8860=EDGE_CURVE('',#7206,#7207,#4080,.T.);
#8861=EDGE_CURVE('',#7206,#7204,#364,.T.);
#8862=EDGE_CURVE('',#7205,#7207,#365,.T.);
#8863=EDGE_CURVE('',#7208,#7209,#4081,.T.);
#8864=EDGE_CURVE('',#7208,#7206,#366,.T.);
#8865=EDGE_CURVE('',#7207,#7209,#367,.T.);
#8866=EDGE_CURVE('',#7210,#7211,#4082,.T.);
#8867=EDGE_CURVE('',#7210,#7208,#368,.T.);
#8868=EDGE_CURVE('',#7209,#7211,#369,.T.);
#8869=EDGE_CURVE('',#7212,#7213,#4083,.T.);
#8870=EDGE_CURVE('',#7212,#7210,#370,.T.);
#8871=EDGE_CURVE('',#7211,#7213,#371,.T.);
#8872=EDGE_CURVE('',#7214,#7215,#4084,.T.);
#8873=EDGE_CURVE('',#7214,#7212,#372,.T.);
#8874=EDGE_CURVE('',#7213,#7215,#373,.T.);
#8875=EDGE_CURVE('',#7216,#7217,#4085,.T.);
#8876=EDGE_CURVE('',#7216,#7214,#374,.T.);
#8877=EDGE_CURVE('',#7215,#7217,#375,.T.);
#8878=EDGE_CURVE('',#7218,#7219,#4086,.T.);
#8879=EDGE_CURVE('',#7218,#7216,#376,.T.);
#8880=EDGE_CURVE('',#7217,#7219,#377,.T.);
#8881=EDGE_CURVE('',#7220,#7221,#4087,.T.);
#8882=EDGE_CURVE('',#7220,#7218,#378,.T.);
#8883=EDGE_CURVE('',#7219,#7221,#379,.T.);
#8884=EDGE_CURVE('',#7222,#7223,#4088,.T.);
#8885=EDGE_CURVE('',#7222,#7220,#380,.T.);
#8886=EDGE_CURVE('',#7221,#7223,#381,.T.);
#8887=EDGE_CURVE('',#7224,#7225,#4089,.T.);
#8888=EDGE_CURVE('',#7224,#7226,#382,.T.);
#8889=EDGE_CURVE('',#7227,#7226,#6600,.T.);
#8890=EDGE_CURVE('',#7225,#7227,#383,.T.);
#8891=EDGE_CURVE('',#7228,#7229,#4090,.T.);
#8892=EDGE_CURVE('',#7228,#7224,#384,.T.);
#8893=EDGE_CURVE('',#7229,#7225,#385,.T.);
#8894=EDGE_CURVE('',#7230,#7231,#4091,.T.);
#8895=EDGE_CURVE('',#7230,#7228,#386,.T.);
#8896=EDGE_CURVE('',#7231,#7229,#387,.T.);
#8897=EDGE_CURVE('',#7232,#7233,#4092,.T.);
#8898=EDGE_CURVE('',#7232,#7230,#388,.T.);
#8899=EDGE_CURVE('',#7233,#7231,#389,.T.);
#8900=EDGE_CURVE('',#7234,#7235,#4093,.T.);
#8901=EDGE_CURVE('',#7234,#7232,#390,.T.);
#8902=EDGE_CURVE('',#7235,#7233,#391,.T.);
#8903=EDGE_CURVE('',#7236,#7237,#4094,.T.);
#8904=EDGE_CURVE('',#7236,#7234,#392,.T.);
#8905=EDGE_CURVE('',#7237,#7235,#393,.T.);
#8906=EDGE_CURVE('',#7238,#7239,#4095,.T.);
#8907=EDGE_CURVE('',#7238,#7236,#394,.T.);
#8908=EDGE_CURVE('',#7239,#7237,#395,.T.);
#8909=EDGE_CURVE('',#7240,#7241,#4096,.T.);
#8910=EDGE_CURVE('',#7240,#7238,#396,.T.);
#8911=EDGE_CURVE('',#7241,#7239,#397,.T.);
#8912=EDGE_CURVE('',#7242,#7243,#4097,.T.);
#8913=EDGE_CURVE('',#7242,#7240,#398,.T.);
#8914=EDGE_CURVE('',#7243,#7241,#399,.T.);
#8915=EDGE_CURVE('',#7244,#7245,#4098,.T.);
#8916=EDGE_CURVE('',#7244,#7242,#400,.T.);
#8917=EDGE_CURVE('',#7245,#7243,#401,.T.);
#8918=EDGE_CURVE('',#7246,#7247,#4099,.T.);
#8919=EDGE_CURVE('',#7246,#7244,#402,.T.);
#8920=EDGE_CURVE('',#7247,#7245,#403,.T.);
#8921=EDGE_CURVE('',#7248,#7249,#4100,.T.);
#8922=EDGE_CURVE('',#7248,#7246,#404,.T.);
#8923=EDGE_CURVE('',#7249,#7247,#405,.T.);
#8924=EDGE_CURVE('',#7250,#7251,#4101,.T.);
#8925=EDGE_CURVE('',#7250,#7248,#406,.T.);
#8926=EDGE_CURVE('',#7251,#7249,#407,.T.);
#8927=EDGE_CURVE('',#7252,#7253,#4102,.T.);
#8928=EDGE_CURVE('',#7252,#7250,#408,.T.);
#8929=EDGE_CURVE('',#7253,#7251,#409,.T.);
#8930=EDGE_CURVE('',#7254,#7255,#4103,.T.);
#8931=EDGE_CURVE('',#7254,#7252,#410,.T.);
#8932=EDGE_CURVE('',#7255,#7253,#411,.T.);
#8933=EDGE_CURVE('',#7256,#7257,#4104,.T.);
#8934=EDGE_CURVE('',#7256,#7258,#412,.T.);
#8935=EDGE_CURVE('',#7258,#7259,#6601,.F.);
#8936=EDGE_CURVE('',#7259,#7257,#413,.T.);
#8937=EDGE_CURVE('',#7260,#7261,#4105,.T.);
#8938=EDGE_CURVE('',#7260,#7256,#414,.T.);
#8939=EDGE_CURVE('',#7257,#7261,#415,.T.);
#8940=EDGE_CURVE('',#7262,#7263,#4106,.T.);
#8941=EDGE_CURVE('',#7262,#7260,#416,.T.);
#8942=EDGE_CURVE('',#7261,#7263,#417,.T.);
#8943=EDGE_CURVE('',#7264,#7265,#4107,.T.);
#8944=EDGE_CURVE('',#7264,#7262,#418,.T.);
#8945=EDGE_CURVE('',#7263,#7265,#419,.T.);
#8946=EDGE_CURVE('',#7266,#7267,#4108,.T.);
#8947=EDGE_CURVE('',#7266,#7264,#420,.T.);
#8948=EDGE_CURVE('',#7265,#7267,#421,.T.);
#8949=EDGE_CURVE('',#7268,#7269,#4109,.T.);
#8950=EDGE_CURVE('',#7268,#7266,#422,.T.);
#8951=EDGE_CURVE('',#7267,#7269,#423,.T.);
#8952=EDGE_CURVE('',#7270,#7271,#4110,.T.);
#8953=EDGE_CURVE('',#7270,#7268,#424,.T.);
#8954=EDGE_CURVE('',#7269,#7271,#425,.T.);
#8955=EDGE_CURVE('',#7272,#7273,#4111,.T.);
#8956=EDGE_CURVE('',#7272,#7270,#426,.T.);
#8957=EDGE_CURVE('',#7271,#7273,#427,.T.);
#8958=EDGE_CURVE('',#7274,#7275,#4112,.T.);
#8959=EDGE_CURVE('',#7274,#7272,#428,.T.);
#8960=EDGE_CURVE('',#7273,#7275,#429,.T.);
#8961=EDGE_CURVE('',#7276,#7277,#4113,.T.);
#8962=EDGE_CURVE('',#7276,#7274,#430,.T.);
#8963=EDGE_CURVE('',#7275,#7277,#431,.T.);
#8964=EDGE_CURVE('',#7278,#7279,#4114,.T.);
#8965=EDGE_CURVE('',#7280,#7278,#6602,.F.);
#8966=EDGE_CURVE('',#7280,#7276,#432,.T.);
#8967=EDGE_CURVE('',#7277,#7279,#433,.T.);
#8968=EDGE_CURVE('',#7281,#7282,#4115,.T.);
#8969=EDGE_CURVE('',#7281,#7283,#434,.T.);
#8970=EDGE_CURVE('',#7284,#7283,#6603,.T.);
#8971=EDGE_CURVE('',#7282,#7284,#435,.T.);
#8972=EDGE_CURVE('',#7285,#7286,#4116,.T.);
#8973=EDGE_CURVE('',#7285,#7281,#436,.T.);
#8974=EDGE_CURVE('',#7286,#7282,#437,.T.);
#8975=EDGE_CURVE('',#7287,#7288,#4117,.T.);
#8976=EDGE_CURVE('',#7287,#7285,#438,.T.);
#8977=EDGE_CURVE('',#7288,#7286,#439,.T.);
#8978=EDGE_CURVE('',#7289,#7290,#4118,.T.);
#8979=EDGE_CURVE('',#7289,#7287,#440,.T.);
#8980=EDGE_CURVE('',#7290,#7288,#441,.T.);
#8981=EDGE_CURVE('',#7291,#7292,#4119,.T.);
#8982=EDGE_CURVE('',#7291,#7289,#442,.T.);
#8983=EDGE_CURVE('',#7292,#7290,#443,.T.);
#8984=EDGE_CURVE('',#7293,#7294,#4120,.T.);
#8985=EDGE_CURVE('',#7293,#7291,#444,.T.);
#8986=EDGE_CURVE('',#7294,#7292,#445,.T.);
#8987=EDGE_CURVE('',#7295,#7296,#4121,.T.);
#8988=EDGE_CURVE('',#7295,#7293,#446,.T.);
#8989=EDGE_CURVE('',#7296,#7294,#447,.T.);
#8990=EDGE_CURVE('',#7297,#7298,#4122,.T.);
#8991=EDGE_CURVE('',#7297,#7295,#448,.T.);
#8992=EDGE_CURVE('',#7298,#7296,#449,.T.);
#8993=EDGE_CURVE('',#7299,#7300,#4123,.T.);
#8994=EDGE_CURVE('',#7299,#7297,#450,.T.);
#8995=EDGE_CURVE('',#7300,#7298,#451,.T.);
#8996=EDGE_CURVE('',#7301,#7302,#4124,.T.);
#8997=EDGE_CURVE('',#7301,#7299,#452,.T.);
#8998=EDGE_CURVE('',#7302,#7300,#453,.T.);
#8999=EDGE_CURVE('',#7303,#7303,#6604,.T.);
#9000=EDGE_CURVE('',#7303,#7304,#4125,.T.);
#9001=EDGE_CURVE('',#7304,#7305,#6605,.T.);
#9002=EDGE_CURVE('',#7305,#7304,#6606,.T.);
#9003=EDGE_CURVE('',#7306,#7307,#6607,.T.);
#9004=EDGE_CURVE('',#7307,#7306,#6608,.T.);
#9005=EDGE_CURVE('',#7307,#7305,#4126,.T.);
#9006=EDGE_CURVE('',#7308,#7308,#6609,.T.);
#9007=EDGE_CURVE('',#7306,#7309,#4127,.T.);
#9008=EDGE_CURVE('',#7309,#7309,#6610,.T.);
#9009=EDGE_CURVE('',#7310,#7310,#6611,.T.);
#9010=EDGE_CURVE('',#7311,#7311,#6612,.T.);
#9011=EDGE_CURVE('',#7311,#7312,#4128,.T.);
#9012=EDGE_CURVE('',#7312,#7313,#6613,.T.);
#9013=EDGE_CURVE('',#7313,#7312,#6614,.T.);
#9014=EDGE_CURVE('',#7313,#7314,#4129,.T.);
#9015=EDGE_CURVE('',#7314,#7314,#6615,.T.);
#9016=EDGE_CURVE('',#7258,#7315,#454,.T.);
#9017=EDGE_CURVE('',#7315,#7316,#6616,.T.);
#9018=EDGE_CURVE('',#7316,#7259,#455,.T.);
#9019=EDGE_CURVE('',#7317,#7317,#6617,.T.);
#9020=EDGE_CURVE('',#7317,#7318,#4130,.T.);
#9021=EDGE_CURVE('',#7319,#7318,#456,.T.);
#9022=EDGE_CURVE('',#7319,#7320,#6618,.T.);
#9023=EDGE_CURVE('',#7318,#7320,#457,.T.);
#9024=EDGE_CURVE('',#7321,#7321,#6619,.T.);
#9025=EDGE_CURVE('',#7321,#7317,#4131,.T.);
#9026=EDGE_CURVE('',#7321,#7322,#4132,.T.);
#9027=EDGE_CURVE('',#7322,#7322,#6620,.T.);
#9028=EDGE_CURVE('',#7323,#7323,#6621,.T.);
#9029=EDGE_CURVE('',#7283,#7280,#458,.T.);
#9030=EDGE_CURVE('',#7324,#7280,#6622,.F.);
#9031=EDGE_CURVE('',#7324,#7284,#459,.T.);
#9032=EDGE_CURVE('',#7279,#7324,#460,.T.);
#9033=EDGE_CURVE('',#7316,#7302,#461,.T.);
#9034=EDGE_CURVE('',#7315,#7301,#462,.T.);
#9035=EDGE_CURVE('',#7278,#7324,#6623,.F.);
#9036=EDGE_CURVE('',#7325,#7227,#463,.T.);
#9037=EDGE_CURVE('',#7223,#7325,#464,.T.);
#9038=EDGE_CURVE('',#7326,#7193,#465,.T.);
#9039=EDGE_CURVE('',#7326,#7255,#466,.T.);
#9040=EDGE_CURVE('',#7193,#7327,#6624,.T.);
#9041=EDGE_CURVE('',#7327,#7192,#6625,.T.);
#9042=EDGE_CURVE('',#7192,#7328,#467,.T.);
#9043=EDGE_CURVE('',#7328,#7326,#6626,.T.);
#9044=EDGE_CURVE('',#7328,#7254,#468,.T.);
#9045=EDGE_CURVE('',#7226,#7329,#469,.T.);
#9046=EDGE_CURVE('',#7329,#7222,#470,.T.);
#9047=EDGE_CURVE('',#7330,#7331,#471,.T.);
#9048=EDGE_CURVE('',#7331,#7332,#4133,.T.);
#9049=EDGE_CURVE('',#7332,#7333,#472,.F.);
#9050=EDGE_CURVE('',#7333,#7330,#4134,.T.);
#9051=EDGE_CURVE('',#7334,#7330,#4135,.T.);
#9052=EDGE_CURVE('',#7335,#7334,#473,.T.);
#9053=EDGE_CURVE('',#7335,#7336,#6627,.T.);
#9054=EDGE_CURVE('',#7337,#7336,#474,.T.);
#9055=EDGE_CURVE('',#7337,#7319,#475,.T.);
#9056=EDGE_CURVE('',#7320,#7338,#476,.T.);
#9057=EDGE_CURVE('',#7339,#7338,#477,.T.);
#9058=EDGE_CURVE('',#7331,#7339,#6628,.T.);
#9059=EDGE_CURVE('',#7340,#7333,#6629,.T.);
#9060=EDGE_CURVE('',#7334,#7340,#4136,.T.);
#9061=EDGE_CURVE('',#7340,#7341,#478,.F.);
#9062=EDGE_CURVE('',#7341,#7335,#4137,.T.);
#9063=EDGE_CURVE('',#7342,#7343,#479,.T.);
#9064=EDGE_CURVE('',#7342,#7339,#4138,.T.);
#9065=EDGE_CURVE('',#7338,#7343,#4139,.T.);
#9066=EDGE_CURVE('',#7336,#7344,#4140,.T.);
#9067=EDGE_CURVE('',#7344,#7345,#480,.F.);
#9068=EDGE_CURVE('',#7345,#7337,#4141,.T.);
#9069=EDGE_CURVE('',#7346,#7346,#6630,.T.);
#9070=EDGE_CURVE('',#7346,#7347,#4142,.T.);
#9071=EDGE_CURVE('',#7347,#7347,#6631,.T.);
#9072=EDGE_CURVE('',#7348,#7348,#6632,.T.);
#9073=EDGE_CURVE('',#7347,#7349,#4143,.T.);
#9074=EDGE_CURVE('',#7349,#7349,#6633,.T.);
#9075=EDGE_CURVE('',#7323,#7350,#4144,.T.);
#9076=EDGE_CURVE('',#7350,#7350,#6634,.T.);
#9077=EDGE_CURVE('',#7350,#7351,#4145,.T.);
#9078=EDGE_CURVE('',#7351,#7351,#6635,.T.);
#9079=EDGE_CURVE('',#7348,#7352,#4146,.T.);
#9080=EDGE_CURVE('',#7352,#7352,#6636,.T.);
#9081=EDGE_CURVE('',#7352,#7353,#4147,.T.);
#9082=EDGE_CURVE('',#7314,#7353,#481,.T.);
#9083=EDGE_CURVE('',#7353,#7314,#482,.T.);
#9084=EDGE_CURVE('',#7343,#7345,#483,.T.);
#9085=EDGE_CURVE('',#7354,#7354,#6637,.T.);
#9086=EDGE_CURVE('',#7354,#7355,#4148,.T.);
#9087=EDGE_CURVE('',#7355,#7355,#6638,.T.);
#9088=EDGE_CURVE('',#7353,#7356,#4149,.T.);
#9089=EDGE_CURVE('',#7356,#7356,#6639,.T.);
#9090=EDGE_CURVE('',#7344,#7341,#4150,.T.);
#9091=EDGE_CURVE('',#7332,#7342,#4151,.T.);
#9092=EDGE_CURVE('',#7308,#7357,#4152,.T.);
#9093=EDGE_CURVE('',#7357,#7357,#6640,.T.);
#9094=EDGE_CURVE('',#7358,#7358,#6641,.T.);
#9095=EDGE_CURVE('',#7327,#7358,#4153,.T.);
#9096=EDGE_CURVE('',#7329,#7325,#6642,.T.);
#9097=EDGE_CURVE('',#7359,#7359,#6643,.T.);
#9098=EDGE_CURVE('',#7356,#7359,#4154,.T.);
#9099=EDGE_CURVE('',#7310,#7278,#4155,.T.);
#11550=ORIENTED_EDGE('',*,*,#8838,.F.);
#11551=ORIENTED_EDGE('',*,*,#8839,.T.);
#11552=ORIENTED_EDGE('',*,*,#8840,.T.);
#11553=ORIENTED_EDGE('',*,*,#8841,.T.);
#11554=ORIENTED_EDGE('',*,*,#8842,.F.);
#11555=ORIENTED_EDGE('',*,*,#8843,.T.);
#11556=ORIENTED_EDGE('',*,*,#8838,.T.);
#11557=ORIENTED_EDGE('',*,*,#8844,.T.);
#11558=ORIENTED_EDGE('',*,*,#8845,.F.);
#11559=ORIENTED_EDGE('',*,*,#8846,.T.);
#11560=ORIENTED_EDGE('',*,*,#8842,.T.);
#11561=ORIENTED_EDGE('',*,*,#8847,.T.);
#11562=ORIENTED_EDGE('',*,*,#8848,.F.);
#11563=ORIENTED_EDGE('',*,*,#8849,.T.);
#11564=ORIENTED_EDGE('',*,*,#8845,.T.);
#11565=ORIENTED_EDGE('',*,*,#8850,.T.);
#11566=ORIENTED_EDGE('',*,*,#8851,.F.);
#11567=ORIENTED_EDGE('',*,*,#8852,.T.);
#11568=ORIENTED_EDGE('',*,*,#8848,.T.);
#11569=ORIENTED_EDGE('',*,*,#8853,.T.);
#11570=ORIENTED_EDGE('',*,*,#8854,.F.);
#11571=ORIENTED_EDGE('',*,*,#8855,.T.);
#11572=ORIENTED_EDGE('',*,*,#8851,.T.);
#11573=ORIENTED_EDGE('',*,*,#8856,.T.);
#11574=ORIENTED_EDGE('',*,*,#8857,.F.);
#11575=ORIENTED_EDGE('',*,*,#8858,.T.);
#11576=ORIENTED_EDGE('',*,*,#8854,.T.);
#11577=ORIENTED_EDGE('',*,*,#8859,.T.);
#11578=ORIENTED_EDGE('',*,*,#8860,.F.);
#11579=ORIENTED_EDGE('',*,*,#8861,.T.);
#11580=ORIENTED_EDGE('',*,*,#8857,.T.);
#11581=ORIENTED_EDGE('',*,*,#8862,.T.);
#11582=ORIENTED_EDGE('',*,*,#8863,.F.);
#11583=ORIENTED_EDGE('',*,*,#8864,.T.);
#11584=ORIENTED_EDGE('',*,*,#8860,.T.);
#11585=ORIENTED_EDGE('',*,*,#8865,.T.);
#11586=ORIENTED_EDGE('',*,*,#8866,.F.);
#11587=ORIENTED_EDGE('',*,*,#8867,.T.);
#11588=ORIENTED_EDGE('',*,*,#8863,.T.);
#11589=ORIENTED_EDGE('',*,*,#8868,.T.);
#11590=ORIENTED_EDGE('',*,*,#8869,.F.);
#11591=ORIENTED_EDGE('',*,*,#8870,.T.);
#11592=ORIENTED_EDGE('',*,*,#8866,.T.);
#11593=ORIENTED_EDGE('',*,*,#8871,.T.);
#11594=ORIENTED_EDGE('',*,*,#8872,.F.);
#11595=ORIENTED_EDGE('',*,*,#8873,.T.);
#11596=ORIENTED_EDGE('',*,*,#8869,.T.);
#11597=ORIENTED_EDGE('',*,*,#8874,.T.);
#11598=ORIENTED_EDGE('',*,*,#8875,.F.);
#11599=ORIENTED_EDGE('',*,*,#8876,.T.);
#11600=ORIENTED_EDGE('',*,*,#8872,.T.);
#11601=ORIENTED_EDGE('',*,*,#8877,.T.);
#11602=ORIENTED_EDGE('',*,*,#8878,.F.);
#11603=ORIENTED_EDGE('',*,*,#8879,.T.);
#11604=ORIENTED_EDGE('',*,*,#8875,.T.);
#11605=ORIENTED_EDGE('',*,*,#8880,.T.);
#11606=ORIENTED_EDGE('',*,*,#8881,.F.);
#11607=ORIENTED_EDGE('',*,*,#8882,.T.);
#11608=ORIENTED_EDGE('',*,*,#8878,.T.);
#11609=ORIENTED_EDGE('',*,*,#8883,.T.);
#11610=ORIENTED_EDGE('',*,*,#8884,.F.);
#11611=ORIENTED_EDGE('',*,*,#8885,.T.);
#11612=ORIENTED_EDGE('',*,*,#8881,.T.);
#11613=ORIENTED_EDGE('',*,*,#8886,.T.);
#11614=ORIENTED_EDGE('',*,*,#8887,.F.);
#11615=ORIENTED_EDGE('',*,*,#8888,.T.);
#11616=ORIENTED_EDGE('',*,*,#8889,.F.);
#11617=ORIENTED_EDGE('',*,*,#8890,.F.);
#11618=ORIENTED_EDGE('',*,*,#8891,.F.);
#11619=ORIENTED_EDGE('',*,*,#8892,.T.);
#11620=ORIENTED_EDGE('',*,*,#8887,.T.);
#11621=ORIENTED_EDGE('',*,*,#8893,.F.);
#11622=ORIENTED_EDGE('',*,*,#8894,.F.);
#11623=ORIENTED_EDGE('',*,*,#8895,.T.);
#11624=ORIENTED_EDGE('',*,*,#8891,.T.);
#11625=ORIENTED_EDGE('',*,*,#8896,.F.);
#11626=ORIENTED_EDGE('',*,*,#8897,.F.);
#11627=ORIENTED_EDGE('',*,*,#8898,.T.);
#11628=ORIENTED_EDGE('',*,*,#8894,.T.);
#11629=ORIENTED_EDGE('',*,*,#8899,.F.);
#11630=ORIENTED_EDGE('',*,*,#8900,.F.);
#11631=ORIENTED_EDGE('',*,*,#8901,.T.);
#11632=ORIENTED_EDGE('',*,*,#8897,.T.);
#11633=ORIENTED_EDGE('',*,*,#8902,.F.);
#11634=ORIENTED_EDGE('',*,*,#8903,.F.);
#11635=ORIENTED_EDGE('',*,*,#8904,.T.);
#11636=ORIENTED_EDGE('',*,*,#8900,.T.);
#11637=ORIENTED_EDGE('',*,*,#8905,.F.);
#11638=ORIENTED_EDGE('',*,*,#8906,.F.);
#11639=ORIENTED_EDGE('',*,*,#8907,.T.);
#11640=ORIENTED_EDGE('',*,*,#8903,.T.);
#11641=ORIENTED_EDGE('',*,*,#8908,.F.);
#11642=ORIENTED_EDGE('',*,*,#8909,.F.);
#11643=ORIENTED_EDGE('',*,*,#8910,.T.);
#11644=ORIENTED_EDGE('',*,*,#8906,.T.);
#11645=ORIENTED_EDGE('',*,*,#8911,.F.);
#11646=ORIENTED_EDGE('',*,*,#8912,.F.);
#11647=ORIENTED_EDGE('',*,*,#8913,.T.);
#11648=ORIENTED_EDGE('',*,*,#8909,.T.);
#11649=ORIENTED_EDGE('',*,*,#8914,.F.);
#11650=ORIENTED_EDGE('',*,*,#8915,.F.);
#11651=ORIENTED_EDGE('',*,*,#8916,.T.);
#11652=ORIENTED_EDGE('',*,*,#8912,.T.);
#11653=ORIENTED_EDGE('',*,*,#8917,.F.);
#11654=ORIENTED_EDGE('',*,*,#8918,.F.);
#11655=ORIENTED_EDGE('',*,*,#8919,.T.);
#11656=ORIENTED_EDGE('',*,*,#8915,.T.);
#11657=ORIENTED_EDGE('',*,*,#8920,.F.);
#11658=ORIENTED_EDGE('',*,*,#8921,.F.);
#11659=ORIENTED_EDGE('',*,*,#8922,.T.);
#11660=ORIENTED_EDGE('',*,*,#8918,.T.);
#11661=ORIENTED_EDGE('',*,*,#8923,.F.);
#11662=ORIENTED_EDGE('',*,*,#8924,.F.);
#11663=ORIENTED_EDGE('',*,*,#8925,.T.);
#11664=ORIENTED_EDGE('',*,*,#8921,.T.);
#11665=ORIENTED_EDGE('',*,*,#8926,.F.);
#11666=ORIENTED_EDGE('',*,*,#8927,.F.);
#11667=ORIENTED_EDGE('',*,*,#8928,.T.);
#11668=ORIENTED_EDGE('',*,*,#8924,.T.);
#11669=ORIENTED_EDGE('',*,*,#8929,.F.);
#11670=ORIENTED_EDGE('',*,*,#8930,.F.);
#11671=ORIENTED_EDGE('',*,*,#8931,.T.);
#11672=ORIENTED_EDGE('',*,*,#8927,.T.);
#11673=ORIENTED_EDGE('',*,*,#8932,.F.);
#11674=ORIENTED_EDGE('',*,*,#8933,.F.);
#11675=ORIENTED_EDGE('',*,*,#8934,.T.);
#11676=ORIENTED_EDGE('',*,*,#8935,.T.);
#11677=ORIENTED_EDGE('',*,*,#8936,.T.);
#11678=ORIENTED_EDGE('',*,*,#8937,.F.);
#11679=ORIENTED_EDGE('',*,*,#8938,.T.);
#11680=ORIENTED_EDGE('',*,*,#8933,.T.);
#11681=ORIENTED_EDGE('',*,*,#8939,.T.);
#11682=ORIENTED_EDGE('',*,*,#8940,.F.);
#11683=ORIENTED_EDGE('',*,*,#8941,.T.);
#11684=ORIENTED_EDGE('',*,*,#8937,.T.);
#11685=ORIENTED_EDGE('',*,*,#8942,.T.);
#11686=ORIENTED_EDGE('',*,*,#8943,.F.);
#11687=ORIENTED_EDGE('',*,*,#8944,.T.);
#11688=ORIENTED_EDGE('',*,*,#8940,.T.);
#11689=ORIENTED_EDGE('',*,*,#8945,.T.);
#11690=ORIENTED_EDGE('',*,*,#8946,.F.);
#11691=ORIENTED_EDGE('',*,*,#8947,.T.);
#11692=ORIENTED_EDGE('',*,*,#8943,.T.);
#11693=ORIENTED_EDGE('',*,*,#8948,.T.);
#11694=ORIENTED_EDGE('',*,*,#8949,.F.);
#11695=ORIENTED_EDGE('',*,*,#8950,.T.);
#11696=ORIENTED_EDGE('',*,*,#8946,.T.);
#11697=ORIENTED_EDGE('',*,*,#8951,.T.);
#11698=ORIENTED_EDGE('',*,*,#8952,.F.);
#11699=ORIENTED_EDGE('',*,*,#8953,.T.);
#11700=ORIENTED_EDGE('',*,*,#8949,.T.);
#11701=ORIENTED_EDGE('',*,*,#8954,.T.);
#11702=ORIENTED_EDGE('',*,*,#8955,.F.);
#11703=ORIENTED_EDGE('',*,*,#8956,.T.);
#11704=ORIENTED_EDGE('',*,*,#8952,.T.);
#11705=ORIENTED_EDGE('',*,*,#8957,.T.);
#11706=ORIENTED_EDGE('',*,*,#8958,.F.);
#11707=ORIENTED_EDGE('',*,*,#8959,.T.);
#11708=ORIENTED_EDGE('',*,*,#8955,.T.);
#11709=ORIENTED_EDGE('',*,*,#8960,.T.);
#11710=ORIENTED_EDGE('',*,*,#8961,.F.);
#11711=ORIENTED_EDGE('',*,*,#8962,.T.);
#11712=ORIENTED_EDGE('',*,*,#8958,.T.);
#11713=ORIENTED_EDGE('',*,*,#8963,.T.);
#11714=ORIENTED_EDGE('',*,*,#8964,.F.);
#11715=ORIENTED_EDGE('',*,*,#8965,.F.);
#11716=ORIENTED_EDGE('',*,*,#8966,.T.);
#11717=ORIENTED_EDGE('',*,*,#8961,.T.);
#11718=ORIENTED_EDGE('',*,*,#8967,.T.);
#11719=ORIENTED_EDGE('',*,*,#8968,.F.);
#11720=ORIENTED_EDGE('',*,*,#8969,.T.);
#11721=ORIENTED_EDGE('',*,*,#8970,.F.);
#11722=ORIENTED_EDGE('',*,*,#8971,.F.);
#11723=ORIENTED_EDGE('',*,*,#8972,.F.);
#11724=ORIENTED_EDGE('',*,*,#8973,.T.);
#11725=ORIENTED_EDGE('',*,*,#8968,.T.);
#11726=ORIENTED_EDGE('',*,*,#8974,.F.);
#11727=ORIENTED_EDGE('',*,*,#8975,.F.);
#11728=ORIENTED_EDGE('',*,*,#8976,.T.);
#11729=ORIENTED_EDGE('',*,*,#8972,.T.);
#11730=ORIENTED_EDGE('',*,*,#8977,.F.);
#11731=ORIENTED_EDGE('',*,*,#8978,.F.);
#11732=ORIENTED_EDGE('',*,*,#8979,.T.);
#11733=ORIENTED_EDGE('',*,*,#8975,.T.);
#11734=ORIENTED_EDGE('',*,*,#8980,.F.);
#11735=ORIENTED_EDGE('',*,*,#8981,.F.);
#11736=ORIENTED_EDGE('',*,*,#8982,.T.);
#11737=ORIENTED_EDGE('',*,*,#8978,.T.);
#11738=ORIENTED_EDGE('',*,*,#8983,.F.);
#11739=ORIENTED_EDGE('',*,*,#8984,.F.);
#11740=ORIENTED_EDGE('',*,*,#8985,.T.);
#11741=ORIENTED_EDGE('',*,*,#8981,.T.);
#11742=ORIENTED_EDGE('',*,*,#8986,.F.);
#11743=ORIENTED_EDGE('',*,*,#8987,.F.);
#11744=ORIENTED_EDGE('',*,*,#8988,.T.);
#11745=ORIENTED_EDGE('',*,*,#8984,.T.);
#11746=ORIENTED_EDGE('',*,*,#8989,.F.);
#11747=ORIENTED_EDGE('',*,*,#8990,.F.);
#11748=ORIENTED_EDGE('',*,*,#8991,.T.);
#11749=ORIENTED_EDGE('',*,*,#8987,.T.);
#11750=ORIENTED_EDGE('',*,*,#8992,.F.);
#11751=ORIENTED_EDGE('',*,*,#8993,.F.);
#11752=ORIENTED_EDGE('',*,*,#8994,.T.);
#11753=ORIENTED_EDGE('',*,*,#8990,.T.);
#11754=ORIENTED_EDGE('',*,*,#8995,.F.);
#11755=ORIENTED_EDGE('',*,*,#8996,.F.);
#11756=ORIENTED_EDGE('',*,*,#8997,.T.);
#11757=ORIENTED_EDGE('',*,*,#8993,.T.);
#11758=ORIENTED_EDGE('',*,*,#8998,.F.);
#11759=ORIENTED_EDGE('',*,*,#8999,.T.);
#11760=ORIENTED_EDGE('',*,*,#9000,.T.);
#11761=ORIENTED_EDGE('',*,*,#9001,.T.);
#11762=ORIENTED_EDGE('',*,*,#9002,.T.);
#11763=ORIENTED_EDGE('',*,*,#9000,.F.);
#11764=ORIENTED_EDGE('',*,*,#9003,.F.);
#11765=ORIENTED_EDGE('',*,*,#9004,.F.);
#11766=ORIENTED_EDGE('',*,*,#9005,.T.);
#11767=ORIENTED_EDGE('',*,*,#9001,.F.);
#11768=ORIENTED_EDGE('',*,*,#9002,.F.);
#11769=ORIENTED_EDGE('',*,*,#9005,.F.);
#11770=ORIENTED_EDGE('',*,*,#9006,.F.);
#11771=ORIENTED_EDGE('',*,*,#8999,.F.);
#11772=ORIENTED_EDGE('',*,*,#9003,.T.);
#11773=ORIENTED_EDGE('',*,*,#9004,.T.);
#11774=ORIENTED_EDGE('',*,*,#9007,.T.);
#11775=ORIENTED_EDGE('',*,*,#9008,.T.);
#11776=ORIENTED_EDGE('',*,*,#9007,.F.);
#11777=ORIENTED_EDGE('',*,*,#9009,.T.);
#11778=ORIENTED_EDGE('',*,*,#9008,.F.);
#11779=ORIENTED_EDGE('',*,*,#9010,.T.);
#11780=ORIENTED_EDGE('',*,*,#9011,.T.);
#11781=ORIENTED_EDGE('',*,*,#9012,.T.);
#11782=ORIENTED_EDGE('',*,*,#9013,.T.);
#11783=ORIENTED_EDGE('',*,*,#9011,.F.);
#11784=ORIENTED_EDGE('',*,*,#9012,.F.);
#11785=ORIENTED_EDGE('',*,*,#9013,.F.);
#11786=ORIENTED_EDGE('',*,*,#9014,.T.);
#11787=ORIENTED_EDGE('',*,*,#9015,.T.);
#11788=ORIENTED_EDGE('',*,*,#9014,.F.);
#11789=ORIENTED_EDGE('',*,*,#9010,.F.);
#11790=ORIENTED_EDGE('',*,*,#9016,.T.);
#11791=ORIENTED_EDGE('',*,*,#9017,.T.);
#11792=ORIENTED_EDGE('',*,*,#9018,.T.);
#11793=ORIENTED_EDGE('',*,*,#8935,.F.);
#11794=ORIENTED_EDGE('',*,*,#9019,.T.);
#11795=ORIENTED_EDGE('',*,*,#9020,.T.);
#11796=ORIENTED_EDGE('',*,*,#9021,.F.);
#11797=ORIENTED_EDGE('',*,*,#9022,.T.);
#11798=ORIENTED_EDGE('',*,*,#9023,.F.);
#11799=ORIENTED_EDGE('',*,*,#9020,.F.);
#11800=ORIENTED_EDGE('',*,*,#9024,.F.);
#11801=ORIENTED_EDGE('',*,*,#9025,.T.);
#11802=ORIENTED_EDGE('',*,*,#9019,.F.);
#11803=ORIENTED_EDGE('',*,*,#9025,.F.);
#11804=ORIENTED_EDGE('',*,*,#9024,.T.);
#11805=ORIENTED_EDGE('',*,*,#9026,.T.);
#11806=ORIENTED_EDGE('',*,*,#9027,.T.);
#11807=ORIENTED_EDGE('',*,*,#9026,.F.);
#11808=ORIENTED_EDGE('',*,*,#9027,.F.);
#11809=ORIENTED_EDGE('',*,*,#9028,.F.);
#11810=ORIENTED_EDGE('',*,*,#8970,.T.);
#11811=ORIENTED_EDGE('',*,*,#9029,.T.);
#11812=ORIENTED_EDGE('',*,*,#9030,.F.);
#11813=ORIENTED_EDGE('',*,*,#9031,.T.);
#11814=ORIENTED_EDGE('',*,*,#9031,.F.);
#11815=ORIENTED_EDGE('',*,*,#9032,.F.);
#11816=ORIENTED_EDGE('',*,*,#8967,.F.);
#11817=ORIENTED_EDGE('',*,*,#8963,.F.);
#11818=ORIENTED_EDGE('',*,*,#8960,.F.);
#11819=ORIENTED_EDGE('',*,*,#8957,.F.);
#11820=ORIENTED_EDGE('',*,*,#8954,.F.);
#11821=ORIENTED_EDGE('',*,*,#8951,.F.);
#11822=ORIENTED_EDGE('',*,*,#8948,.F.);
#11823=ORIENTED_EDGE('',*,*,#8945,.F.);
#11824=ORIENTED_EDGE('',*,*,#8942,.F.);
#11825=ORIENTED_EDGE('',*,*,#8939,.F.);
#11826=ORIENTED_EDGE('',*,*,#8936,.F.);
#11827=ORIENTED_EDGE('',*,*,#9018,.F.);
#11828=ORIENTED_EDGE('',*,*,#9033,.T.);
#11829=ORIENTED_EDGE('',*,*,#8998,.T.);
#11830=ORIENTED_EDGE('',*,*,#8995,.T.);
#11831=ORIENTED_EDGE('',*,*,#8992,.T.);
#11832=ORIENTED_EDGE('',*,*,#8989,.T.);
#11833=ORIENTED_EDGE('',*,*,#8986,.T.);
#11834=ORIENTED_EDGE('',*,*,#8983,.T.);
#11835=ORIENTED_EDGE('',*,*,#8980,.T.);
#11836=ORIENTED_EDGE('',*,*,#8977,.T.);
#11837=ORIENTED_EDGE('',*,*,#8974,.T.);
#11838=ORIENTED_EDGE('',*,*,#8971,.T.);
#11839=ORIENTED_EDGE('',*,*,#8996,.T.);
#11840=ORIENTED_EDGE('',*,*,#9033,.F.);
#11841=ORIENTED_EDGE('',*,*,#9017,.F.);
#11842=ORIENTED_EDGE('',*,*,#9034,.T.);
#11843=ORIENTED_EDGE('',*,*,#9029,.F.);
#11844=ORIENTED_EDGE('',*,*,#8969,.F.);
#11845=ORIENTED_EDGE('',*,*,#8973,.F.);
#11846=ORIENTED_EDGE('',*,*,#8976,.F.);
#11847=ORIENTED_EDGE('',*,*,#8979,.F.);
#11848=ORIENTED_EDGE('',*,*,#8982,.F.);
#11849=ORIENTED_EDGE('',*,*,#8985,.F.);
#11850=ORIENTED_EDGE('',*,*,#8988,.F.);
#11851=ORIENTED_EDGE('',*,*,#8991,.F.);
#11852=ORIENTED_EDGE('',*,*,#8994,.F.);
#11853=ORIENTED_EDGE('',*,*,#8997,.F.);
#11854=ORIENTED_EDGE('',*,*,#9034,.F.);
#11855=ORIENTED_EDGE('',*,*,#9016,.F.);
#11856=ORIENTED_EDGE('',*,*,#8934,.F.);
#11857=ORIENTED_EDGE('',*,*,#8938,.F.);
#11858=ORIENTED_EDGE('',*,*,#8941,.F.);
#11859=ORIENTED_EDGE('',*,*,#8944,.F.);
#11860=ORIENTED_EDGE('',*,*,#8947,.F.);
#11861=ORIENTED_EDGE('',*,*,#8950,.F.);
#11862=ORIENTED_EDGE('',*,*,#8953,.F.);
#11863=ORIENTED_EDGE('',*,*,#8956,.F.);
#11864=ORIENTED_EDGE('',*,*,#8959,.F.);
#11865=ORIENTED_EDGE('',*,*,#8962,.F.);
#11866=ORIENTED_EDGE('',*,*,#8966,.F.);
#11867=ORIENTED_EDGE('',*,*,#8964,.T.);
#11868=ORIENTED_EDGE('',*,*,#9032,.T.);
#11869=ORIENTED_EDGE('',*,*,#9035,.F.);
#11870=ORIENTED_EDGE('',*,*,#9036,.F.);
#11871=ORIENTED_EDGE('',*,*,#9037,.F.);
#11872=ORIENTED_EDGE('',*,*,#8886,.F.);
#11873=ORIENTED_EDGE('',*,*,#8883,.F.);
#11874=ORIENTED_EDGE('',*,*,#8880,.F.);
#11875=ORIENTED_EDGE('',*,*,#8877,.F.);
#11876=ORIENTED_EDGE('',*,*,#8874,.F.);
#11877=ORIENTED_EDGE('',*,*,#8871,.F.);
#11878=ORIENTED_EDGE('',*,*,#8868,.F.);
#11879=ORIENTED_EDGE('',*,*,#8865,.F.);
#11880=ORIENTED_EDGE('',*,*,#8862,.F.);
#11881=ORIENTED_EDGE('',*,*,#8859,.F.);
#11882=ORIENTED_EDGE('',*,*,#8856,.F.);
#11883=ORIENTED_EDGE('',*,*,#8853,.F.);
#11884=ORIENTED_EDGE('',*,*,#8850,.F.);
#11885=ORIENTED_EDGE('',*,*,#8847,.F.);
#11886=ORIENTED_EDGE('',*,*,#8844,.F.);
#11887=ORIENTED_EDGE('',*,*,#8841,.F.);
#11888=ORIENTED_EDGE('',*,*,#9038,.F.);
#11889=ORIENTED_EDGE('',*,*,#9039,.T.);
#11890=ORIENTED_EDGE('',*,*,#8932,.T.);
#11891=ORIENTED_EDGE('',*,*,#8929,.T.);
#11892=ORIENTED_EDGE('',*,*,#8926,.T.);
#11893=ORIENTED_EDGE('',*,*,#8923,.T.);
#11894=ORIENTED_EDGE('',*,*,#8920,.T.);
#11895=ORIENTED_EDGE('',*,*,#8917,.T.);
#11896=ORIENTED_EDGE('',*,*,#8914,.T.);
#11897=ORIENTED_EDGE('',*,*,#8911,.T.);
#11898=ORIENTED_EDGE('',*,*,#8908,.T.);
#11899=ORIENTED_EDGE('',*,*,#8905,.T.);
#11900=ORIENTED_EDGE('',*,*,#8902,.T.);
#11901=ORIENTED_EDGE('',*,*,#8899,.T.);
#11902=ORIENTED_EDGE('',*,*,#8896,.T.);
#11903=ORIENTED_EDGE('',*,*,#8893,.T.);
#11904=ORIENTED_EDGE('',*,*,#8890,.T.);
#11905=ORIENTED_EDGE('',*,*,#9040,.T.);
#11906=ORIENTED_EDGE('',*,*,#9041,.T.);
#11907=ORIENTED_EDGE('',*,*,#9042,.T.);
#11908=ORIENTED_EDGE('',*,*,#9043,.T.);
#11909=ORIENTED_EDGE('',*,*,#9038,.T.);
#11910=ORIENTED_EDGE('',*,*,#8930,.T.);
#11911=ORIENTED_EDGE('',*,*,#9039,.F.);
#11912=ORIENTED_EDGE('',*,*,#9043,.F.);
#11913=ORIENTED_EDGE('',*,*,#9044,.T.);
#11914=ORIENTED_EDGE('',*,*,#9045,.F.);
#11915=ORIENTED_EDGE('',*,*,#8888,.F.);
#11916=ORIENTED_EDGE('',*,*,#8892,.F.);
#11917=ORIENTED_EDGE('',*,*,#8895,.F.);
#11918=ORIENTED_EDGE('',*,*,#8898,.F.);
#11919=ORIENTED_EDGE('',*,*,#8901,.F.);
#11920=ORIENTED_EDGE('',*,*,#8904,.F.);
#11921=ORIENTED_EDGE('',*,*,#8907,.F.);
#11922=ORIENTED_EDGE('',*,*,#8910,.F.);
#11923=ORIENTED_EDGE('',*,*,#8913,.F.);
#11924=ORIENTED_EDGE('',*,*,#8916,.F.);
#11925=ORIENTED_EDGE('',*,*,#8919,.F.);
#11926=ORIENTED_EDGE('',*,*,#8922,.F.);
#11927=ORIENTED_EDGE('',*,*,#8925,.F.);
#11928=ORIENTED_EDGE('',*,*,#8928,.F.);
#11929=ORIENTED_EDGE('',*,*,#8931,.F.);
#11930=ORIENTED_EDGE('',*,*,#9044,.F.);
#11931=ORIENTED_EDGE('',*,*,#9042,.F.);
#11932=ORIENTED_EDGE('',*,*,#8839,.F.);
#11933=ORIENTED_EDGE('',*,*,#8843,.F.);
#11934=ORIENTED_EDGE('',*,*,#8846,.F.);
#11935=ORIENTED_EDGE('',*,*,#8849,.F.);
#11936=ORIENTED_EDGE('',*,*,#8852,.F.);
#11937=ORIENTED_EDGE('',*,*,#8855,.F.);
#11938=ORIENTED_EDGE('',*,*,#8858,.F.);
#11939=ORIENTED_EDGE('',*,*,#8861,.F.);
#11940=ORIENTED_EDGE('',*,*,#8864,.F.);
#11941=ORIENTED_EDGE('',*,*,#8867,.F.);
#11942=ORIENTED_EDGE('',*,*,#8870,.F.);
#11943=ORIENTED_EDGE('',*,*,#8873,.F.);
#11944=ORIENTED_EDGE('',*,*,#8876,.F.);
#11945=ORIENTED_EDGE('',*,*,#8879,.F.);
#11946=ORIENTED_EDGE('',*,*,#8882,.F.);
#11947=ORIENTED_EDGE('',*,*,#8885,.F.);
#11948=ORIENTED_EDGE('',*,*,#9046,.F.);
#11949=ORIENTED_EDGE('',*,*,#9047,.T.);
#11950=ORIENTED_EDGE('',*,*,#9048,.T.);
#11951=ORIENTED_EDGE('',*,*,#9049,.T.);
#11952=ORIENTED_EDGE('',*,*,#9050,.T.);
#11953=ORIENTED_EDGE('',*,*,#9047,.F.);
#11954=ORIENTED_EDGE('',*,*,#9051,.F.);
#11955=ORIENTED_EDGE('',*,*,#9052,.F.);
#11956=ORIENTED_EDGE('',*,*,#9053,.T.);
#11957=ORIENTED_EDGE('',*,*,#9054,.F.);
#11958=ORIENTED_EDGE('',*,*,#9055,.T.);
#11959=ORIENTED_EDGE('',*,*,#9021,.T.);
#11960=ORIENTED_EDGE('',*,*,#9023,.T.);
#11961=ORIENTED_EDGE('',*,*,#9056,.T.);
#11962=ORIENTED_EDGE('',*,*,#9057,.F.);
#11963=ORIENTED_EDGE('',*,*,#9058,.F.);
#11964=ORIENTED_EDGE('',*,*,#9050,.F.);
#11965=ORIENTED_EDGE('',*,*,#9059,.F.);
#11966=ORIENTED_EDGE('',*,*,#9060,.F.);
#11967=ORIENTED_EDGE('',*,*,#9051,.T.);
#11968=ORIENTED_EDGE('',*,*,#9052,.T.);
#11969=ORIENTED_EDGE('',*,*,#9060,.T.);
#11970=ORIENTED_EDGE('',*,*,#9061,.T.);
#11971=ORIENTED_EDGE('',*,*,#9062,.T.);
#11972=ORIENTED_EDGE('',*,*,#9063,.F.);
#11973=ORIENTED_EDGE('',*,*,#9064,.T.);
#11974=ORIENTED_EDGE('',*,*,#9057,.T.);
#11975=ORIENTED_EDGE('',*,*,#9065,.T.);
#11976=ORIENTED_EDGE('',*,*,#9054,.T.);
#11977=ORIENTED_EDGE('',*,*,#9066,.T.);
#11978=ORIENTED_EDGE('',*,*,#9067,.T.);
#11979=ORIENTED_EDGE('',*,*,#9068,.T.);
#11980=ORIENTED_EDGE('',*,*,#9069,.T.);
#11981=ORIENTED_EDGE('',*,*,#9070,.T.);
#11982=ORIENTED_EDGE('',*,*,#9071,.T.);
#11983=ORIENTED_EDGE('',*,*,#9070,.F.);
#11984=ORIENTED_EDGE('',*,*,#9072,.F.);
#11985=ORIENTED_EDGE('',*,*,#9069,.F.);
#11986=ORIENTED_EDGE('',*,*,#9071,.F.);
#11987=ORIENTED_EDGE('',*,*,#9073,.T.);
#11988=ORIENTED_EDGE('',*,*,#9074,.T.);
#11989=ORIENTED_EDGE('',*,*,#9073,.F.);
#11990=ORIENTED_EDGE('',*,*,#9028,.T.);
#11991=ORIENTED_EDGE('',*,*,#9075,.T.);
#11992=ORIENTED_EDGE('',*,*,#9076,.T.);
#11993=ORIENTED_EDGE('',*,*,#9075,.F.);
#11994=ORIENTED_EDGE('',*,*,#9076,.F.);
#11995=ORIENTED_EDGE('',*,*,#9077,.T.);
#11996=ORIENTED_EDGE('',*,*,#9078,.T.);
#11997=ORIENTED_EDGE('',*,*,#9077,.F.);
#11998=ORIENTED_EDGE('',*,*,#9072,.T.);
#11999=ORIENTED_EDGE('',*,*,#9079,.T.);
#12000=ORIENTED_EDGE('',*,*,#9080,.T.);
#12001=ORIENTED_EDGE('',*,*,#9079,.F.);
#12002=ORIENTED_EDGE('',*,*,#9080,.F.);
#12003=ORIENTED_EDGE('',*,*,#9081,.T.);
#12004=ORIENTED_EDGE('',*,*,#9082,.F.);
#12005=ORIENTED_EDGE('',*,*,#9083,.F.);
#12006=ORIENTED_EDGE('',*,*,#9081,.F.);
#12007=ORIENTED_EDGE('',*,*,#9022,.F.);
#12008=ORIENTED_EDGE('',*,*,#9055,.F.);
#12009=ORIENTED_EDGE('',*,*,#9068,.F.);
#12010=ORIENTED_EDGE('',*,*,#9084,.F.);
#12011=ORIENTED_EDGE('',*,*,#9065,.F.);
#12012=ORIENTED_EDGE('',*,*,#9056,.F.);
#12013=ORIENTED_EDGE('',*,*,#9074,.F.);
#12014=ORIENTED_EDGE('',*,*,#9078,.F.);
#12015=ORIENTED_EDGE('',*,*,#9085,.F.);
#12016=ORIENTED_EDGE('',*,*,#9086,.T.);
#12017=ORIENTED_EDGE('',*,*,#9087,.F.);
#12018=ORIENTED_EDGE('',*,*,#9086,.F.);
#12019=ORIENTED_EDGE('',*,*,#9015,.F.);
#12020=ORIENTED_EDGE('',*,*,#9082,.T.);
#12021=ORIENTED_EDGE('',*,*,#9088,.T.);
#12022=ORIENTED_EDGE('',*,*,#9089,.T.);
#12023=ORIENTED_EDGE('',*,*,#9088,.F.);
#12024=ORIENTED_EDGE('',*,*,#9083,.T.);
#12025=ORIENTED_EDGE('',*,*,#9084,.T.);
#12026=ORIENTED_EDGE('',*,*,#9067,.F.);
#12027=ORIENTED_EDGE('',*,*,#9090,.T.);
#12028=ORIENTED_EDGE('',*,*,#9061,.F.);
#12029=ORIENTED_EDGE('',*,*,#9059,.T.);
#12030=ORIENTED_EDGE('',*,*,#9049,.F.);
#12031=ORIENTED_EDGE('',*,*,#9091,.T.);
#12032=ORIENTED_EDGE('',*,*,#9063,.T.);
#12033=ORIENTED_EDGE('',*,*,#9062,.F.);
#12034=ORIENTED_EDGE('',*,*,#9090,.F.);
#12035=ORIENTED_EDGE('',*,*,#9066,.F.);
#12036=ORIENTED_EDGE('',*,*,#9053,.F.);
#12037=ORIENTED_EDGE('',*,*,#9085,.T.);
#12038=ORIENTED_EDGE('',*,*,#9048,.F.);
#12039=ORIENTED_EDGE('',*,*,#9058,.T.);
#12040=ORIENTED_EDGE('',*,*,#9064,.F.);
#12041=ORIENTED_EDGE('',*,*,#9091,.F.);
#12042=ORIENTED_EDGE('',*,*,#9087,.T.);
#12043=ORIENTED_EDGE('',*,*,#9006,.T.);
#12044=ORIENTED_EDGE('',*,*,#9092,.T.);
#12045=ORIENTED_EDGE('',*,*,#9093,.F.);
#12046=ORIENTED_EDGE('',*,*,#9092,.F.);
#12047=ORIENTED_EDGE('',*,*,#9094,.F.);
#12048=ORIENTED_EDGE('',*,*,#9093,.T.);
#12049=ORIENTED_EDGE('',*,*,#9040,.F.);
#12050=ORIENTED_EDGE('',*,*,#8840,.F.);
#12051=ORIENTED_EDGE('',*,*,#9041,.F.);
#12052=ORIENTED_EDGE('',*,*,#9095,.T.);
#12053=ORIENTED_EDGE('',*,*,#9094,.T.);
#12054=ORIENTED_EDGE('',*,*,#9095,.F.);
#12055=ORIENTED_EDGE('',*,*,#8884,.T.);
#12056=ORIENTED_EDGE('',*,*,#9037,.T.);
#12057=ORIENTED_EDGE('',*,*,#9096,.F.);
#12058=ORIENTED_EDGE('',*,*,#9046,.T.);
#12059=ORIENTED_EDGE('',*,*,#9097,.F.);
#12060=ORIENTED_EDGE('',*,*,#9096,.T.);
#12061=ORIENTED_EDGE('',*,*,#9036,.T.);
#12062=ORIENTED_EDGE('',*,*,#8889,.T.);
#12063=ORIENTED_EDGE('',*,*,#9045,.T.);
#12064=ORIENTED_EDGE('',*,*,#9089,.F.);
#12065=ORIENTED_EDGE('',*,*,#9098,.T.);
#12066=ORIENTED_EDGE('',*,*,#9097,.T.);
#12067=ORIENTED_EDGE('',*,*,#9098,.F.);
#12068=ORIENTED_EDGE('',*,*,#9009,.F.);
#12069=ORIENTED_EDGE('',*,*,#9099,.T.);
#12070=ORIENTED_EDGE('',*,*,#9035,.T.);
#12071=ORIENTED_EDGE('',*,*,#9030,.T.);
#12072=ORIENTED_EDGE('',*,*,#8965,.T.);
#12073=ORIENTED_EDGE('',*,*,#9099,.F.);
#15482=CONICAL_SURFACE('',#17027,4.25,0.785398163397441);
#15483=CONICAL_SURFACE('',#17036,4.25,0.785398163397441);
#15484=CONICAL_SURFACE('',#17040,24.9267766952966,1.17809724509617);
#15485=CONICAL_SURFACE('',#17044,25.5,0.785398163397451);
#15486=CONICAL_SURFACE('',#17048,9.82322330470336,0.39269908169873);
#15487=CONICAL_SURFACE('',#17051,9.6,0.785398163397448);
#15488=CONICAL_SURFACE('',#17053,9.12677669529663,1.17809724509617);
#15489=CONICAL_SURFACE('',#17076,5.25,0.785398163397437);
#15490=CONICAL_SURFACE('',#17083,4.20999999999999,0.785398163397437);
#15491=CONICAL_SURFACE('',#17087,12.6,0.785398163397448);
#15492=CONICAL_SURFACE('',#17104,20.6,0.785398163397448);
#15493=CONICAL_SURFACE('',#17109,25.5,0.785398163397442);
#15494=CONICAL_SURFACE('',#17110,16.1,0.785398163397437);
#15698=ADVANCED_FACE('',(#1970),#1605,.T.);
#15699=ADVANCED_FACE('',(#1971),#1606,.T.);
#15700=ADVANCED_FACE('',(#1972),#1607,.T.);
#15701=ADVANCED_FACE('',(#1973),#1608,.T.);
#15702=ADVANCED_FACE('',(#1974),#1609,.T.);
#15703=ADVANCED_FACE('',(#1975),#1610,.T.);
#15704=ADVANCED_FACE('',(#1976),#1611,.T.);
#15705=ADVANCED_FACE('',(#1977),#1612,.T.);
#15706=ADVANCED_FACE('',(#1978),#1613,.T.);
#15707=ADVANCED_FACE('',(#1979),#1614,.T.);
#15708=ADVANCED_FACE('',(#1980),#1615,.T.);
#15709=ADVANCED_FACE('',(#1981),#1616,.T.);
#15710=ADVANCED_FACE('',(#1982),#1617,.T.);
#15711=ADVANCED_FACE('',(#1983),#1618,.T.);
#15712=ADVANCED_FACE('',(#1984),#1619,.T.);
#15713=ADVANCED_FACE('',(#1985),#1620,.T.);
#15714=ADVANCED_FACE('',(#1986),#1621,.T.);
#15715=ADVANCED_FACE('',(#1987),#1622,.T.);
#15716=ADVANCED_FACE('',(#1988),#1623,.T.);
#15717=ADVANCED_FACE('',(#1989),#1624,.T.);
#15718=ADVANCED_FACE('',(#1990),#1625,.T.);
#15719=ADVANCED_FACE('',(#1991),#1626,.T.);
#15720=ADVANCED_FACE('',(#1992),#1627,.T.);
#15721=ADVANCED_FACE('',(#1993),#1628,.T.);
#15722=ADVANCED_FACE('',(#1994),#1629,.T.);
#15723=ADVANCED_FACE('',(#1995),#1630,.T.);
#15724=ADVANCED_FACE('',(#1996),#1631,.T.);
#15725=ADVANCED_FACE('',(#1997),#1632,.T.);
#15726=ADVANCED_FACE('',(#1998),#1633,.T.);
#15727=ADVANCED_FACE('',(#1999),#1634,.T.);
#15728=ADVANCED_FACE('',(#2000),#1635,.T.);
#15729=ADVANCED_FACE('',(#2001),#1636,.T.);
#15730=ADVANCED_FACE('',(#2002),#1637,.T.);
#15731=ADVANCED_FACE('',(#2003),#1638,.T.);
#15732=ADVANCED_FACE('',(#2004),#1639,.T.);
#15733=ADVANCED_FACE('',(#2005),#1640,.T.);
#15734=ADVANCED_FACE('',(#2006),#1641,.T.);
#15735=ADVANCED_FACE('',(#2007),#1642,.T.);
#15736=ADVANCED_FACE('',(#2008),#1643,.T.);
#15737=ADVANCED_FACE('',(#2009),#1644,.T.);
#15738=ADVANCED_FACE('',(#2010),#1645,.T.);
#15739=ADVANCED_FACE('',(#2011),#1646,.T.);
#15740=ADVANCED_FACE('',(#2012),#1647,.T.);
#15741=ADVANCED_FACE('',(#2013),#1648,.T.);
#15742=ADVANCED_FACE('',(#2014),#1649,.T.);
#15743=ADVANCED_FACE('',(#2015),#1650,.T.);
#15744=ADVANCED_FACE('',(#2016),#1651,.T.);
#15745=ADVANCED_FACE('',(#2017),#1652,.T.);
#15746=ADVANCED_FACE('',(#2018),#1653,.T.);
#15747=ADVANCED_FACE('',(#2019),#1654,.T.);
#15748=ADVANCED_FACE('',(#2020),#1655,.T.);
#15749=ADVANCED_FACE('',(#2021),#1656,.T.);
#15750=ADVANCED_FACE('',(#2022),#15482,.F.);
#15751=ADVANCED_FACE('',(#2023),#1657,.F.);
#15752=ADVANCED_FACE('',(#2024,#947),#1108,.T.);
#15753=ADVANCED_FACE('',(#2025),#15483,.F.);
#15754=ADVANCED_FACE('',(#2026,#948),#1109,.T.);
#15755=ADVANCED_FACE('',(#2027),#15484,.T.);
#15756=ADVANCED_FACE('',(#2028),#15485,.T.);
#15757=ADVANCED_FACE('',(#2029,#949),#1110,.T.);
#15758=ADVANCED_FACE('',(#2030),#15486,.T.);
#15759=ADVANCED_FACE('',(#2031),#15487,.T.);
#15760=ADVANCED_FACE('',(#2032),#15488,.T.);
#15761=ADVANCED_FACE('',(#2033,#950),#1111,.T.);
#15762=ADVANCED_FACE('',(#2034),#1112,.F.);
#15763=ADVANCED_FACE('',(#2035),#853,.F.);
#15764=ADVANCED_FACE('',(#2036),#1658,.T.);
#15765=ADVANCED_FACE('',(#2037),#854,.F.);
#15766=ADVANCED_FACE('',(#2038),#1659,.T.);
#15767=ADVANCED_FACE('',(#2039),#855,.F.);
#15768=ADVANCED_FACE('',(#2040),#1113,.T.);
#15769=ADVANCED_FACE('',(#2041),#1660,.T.);
#15770=ADVANCED_FACE('',(#2042),#856,.F.);
#15771=ADVANCED_FACE('',(#2043),#1661,.T.);
#15772=ADVANCED_FACE('',(#2044),#1662,.T.);
#15773=ADVANCED_FACE('',(#2045),#1114,.T.);
#15774=ADVANCED_FACE('',(#2046),#1663,.T.);
#15775=ADVANCED_FACE('',(#2047),#1664,.T.);
#15776=ADVANCED_FACE('',(#2048),#1665,.T.);
#15777=ADVANCED_FACE('',(#2049),#15489,.F.);
#15778=ADVANCED_FACE('',(#2050,#951),#1115,.F.);
#15779=ADVANCED_FACE('',(#2051),#1666,.F.);
#15780=ADVANCED_FACE('',(#2052),#15490,.F.);
#15781=ADVANCED_FACE('',(#2053),#1667,.F.);
#15782=ADVANCED_FACE('',(#2054),#15491,.T.);
#15783=ADVANCED_FACE('',(#2055),#1668,.T.);
#15784=ADVANCED_FACE('',(#2056),#1669,.T.);
#15785=ADVANCED_FACE('',(#2057),#1116,.F.);
#15786=ADVANCED_FACE('',(#2058),#1117,.T.);
#15787=ADVANCED_FACE('',(#2059),#1670,.F.);
#15788=ADVANCED_FACE('',(#2060,#952),#1671,.T.);
#15789=ADVANCED_FACE('',(#2061,#953),#1118,.F.);
#15790=ADVANCED_FACE('',(#2062,#954),#1119,.T.);
#15791=ADVANCED_FACE('',(#2063),#1672,.F.);
#15792=ADVANCED_FACE('',(#2064,#955),#1120,.T.);
#15793=ADVANCED_FACE('',(#2065),#15492,.T.);
#15794=ADVANCED_FACE('',(#2066),#1673,.T.);
#15795=ADVANCED_FACE('',(#2067,#956),#1121,.T.);
#15796=ADVANCED_FACE('',(#2068),#15493,.T.);
#15797=ADVANCED_FACE('',(#2069),#15494,.T.);
#16518=CLOSED_SHELL('',(#15698,#15699,#15700,#15701,#15702,#15703,#15704,
#15705,#15706,#15707,#15708,#15709,#15710,#15711,#15712,#15713,#15714,#15715,
#15716,#15717,#15718,#15719,#15720,#15721,#15722,#15723,#15724,#15725,#15726,
#15727,#15728,#15729,#15730,#15731,#15732,#15733,#15734,#15735,#15736,#15737,
#15738,#15739,#15740,#15741,#15742,#15743,#15744,#15745,#15746,#15747,#15748,
#15749,#15750,#15751,#15752,#15753,#15754,#15755,#15756,#15757,#15758,#15759,
#15760,#15761,#15762,#15763,#15764,#15765,#15766,#15767,#15768,#15769,#15770,
#15771,#15772,#15773,#15774,#15775,#15776,#15777,#15778,#15779,#15780,#15781,
#15782,#15783,#15784,#15785,#15786,#15787,#15788,#15789,#15790,#15791,#15792,
#15793,#15794,#15795,#15796,#15797));
#16969=AXIS2_PLACEMENT_3D('',#23909,#18732,#18733);
#16970=AXIS2_PLACEMENT_3D('',#23910,#18734,#18735);
#16971=AXIS2_PLACEMENT_3D('',#23932,#18737,#18738);
#16972=AXIS2_PLACEMENT_3D('',#23943,#18739,#18740);
#16973=AXIS2_PLACEMENT_3D('',#24027,#18742,#18743);
#16974=AXIS2_PLACEMENT_3D('',#24117,#18745,#18746);
#16975=AXIS2_PLACEMENT_3D('',#24207,#18748,#18749);
#16976=AXIS2_PLACEMENT_3D('',#24291,#18751,#18752);
#16977=AXIS2_PLACEMENT_3D('',#24381,#18754,#18755);
#16978=AXIS2_PLACEMENT_3D('',#24465,#18757,#18758);
#16979=AXIS2_PLACEMENT_3D('',#24555,#18760,#18761);
#16980=AXIS2_PLACEMENT_3D('',#24645,#18763,#18764);
#16981=AXIS2_PLACEMENT_3D('',#24729,#18766,#18767);
#16982=AXIS2_PLACEMENT_3D('',#24819,#18769,#18770);
#16983=AXIS2_PLACEMENT_3D('',#24909,#18772,#18773);
#16984=AXIS2_PLACEMENT_3D('',#24993,#18775,#18776);
#16985=AXIS2_PLACEMENT_3D('',#25083,#18778,#18779);
#16986=AXIS2_PLACEMENT_3D('',#25167,#18781,#18782);
#16987=AXIS2_PLACEMENT_3D('',#25257,#18784,#18785);
#16988=AXIS2_PLACEMENT_3D('',#25278,#18787,#18788);
#16989=AXIS2_PLACEMENT_3D('',#25291,#18789,#18790);
#16990=AXIS2_PLACEMENT_3D('',#25328,#18792,#18793);
#16991=AXIS2_PLACEMENT_3D('',#25365,#18795,#18796);
#16992=AXIS2_PLACEMENT_3D('',#25402,#18798,#18799);
#16993=AXIS2_PLACEMENT_3D('',#25439,#18801,#18802);
#16994=AXIS2_PLACEMENT_3D('',#25477,#18804,#18805);
#16995=AXIS2_PLACEMENT_3D('',#25514,#18807,#18808);
#16996=AXIS2_PLACEMENT_3D('',#25551,#18810,#18811);
#16997=AXIS2_PLACEMENT_3D('',#25589,#18813,#18814);
#16998=AXIS2_PLACEMENT_3D('',#25626,#18816,#18817);
#16999=AXIS2_PLACEMENT_3D('',#25663,#18819,#18820);
#17000=AXIS2_PLACEMENT_3D('',#25700,#18822,#18823);
#17001=AXIS2_PLACEMENT_3D('',#25737,#18825,#18826);
#17002=AXIS2_PLACEMENT_3D('',#25775,#18828,#18829);
#17003=AXIS2_PLACEMENT_3D('',#25812,#18831,#18832);
#17004=AXIS2_PLACEMENT_3D('',#25834,#18834,#18835);
#17005=AXIS2_PLACEMENT_3D('',#25845,#18836,#18837);
#17006=AXIS2_PLACEMENT_3D('',#25935,#18839,#18840);
#17007=AXIS2_PLACEMENT_3D('',#26019,#18842,#18843);
#17008=AXIS2_PLACEMENT_3D('',#26109,#18845,#18846);
#17009=AXIS2_PLACEMENT_3D('',#26199,#18848,#18849);
#17010=AXIS2_PLACEMENT_3D('',#26289,#18851,#18852);
#17011=AXIS2_PLACEMENT_3D('',#26373,#18854,#18855);
#17012=AXIS2_PLACEMENT_3D('',#26463,#18857,#18858);
#17013=AXIS2_PLACEMENT_3D('',#26553,#18860,#18861);
#17014=AXIS2_PLACEMENT_3D('',#26640,#18863,#18864);
#17015=AXIS2_PLACEMENT_3D('',#26645,#18866,#18867);
#17016=AXIS2_PLACEMENT_3D('',#26723,#18868,#18869);
#17017=AXIS2_PLACEMENT_3D('',#26739,#18871,#18872);
#17018=AXIS2_PLACEMENT_3D('',#26748,#18873,#18874);
#17019=AXIS2_PLACEMENT_3D('',#26786,#18876,#18877);
#17020=AXIS2_PLACEMENT_3D('',#26823,#18879,#18880);
#17021=AXIS2_PLACEMENT_3D('',#26861,#18882,#18883);
#17022=AXIS2_PLACEMENT_3D('',#26898,#18885,#18886);
#17023=AXIS2_PLACEMENT_3D('',#26935,#18888,#18889);
#17024=AXIS2_PLACEMENT_3D('',#26973,#18891,#18892);
#17025=AXIS2_PLACEMENT_3D('',#27011,#18894,#18895);
#17026=AXIS2_PLACEMENT_3D('',#27048,#18897,#18898);
#17027=AXIS2_PLACEMENT_3D('',#27085,#18900,#18901);
#17028=AXIS2_PLACEMENT_3D('',#27087,#18902,#18903);
#17029=AXIS2_PLACEMENT_3D('',#27091,#18905,#18906);
#17030=AXIS2_PLACEMENT_3D('',#27092,#18907,#18908);
#17031=AXIS2_PLACEMENT_3D('',#27093,#18909,#18910);
#17032=AXIS2_PLACEMENT_3D('',#27096,#18911,#18912);
#17033=AXIS2_PLACEMENT_3D('',#27097,#18913,#18914);
#17034=AXIS2_PLACEMENT_3D('',#27099,#18916,#18917);
#17035=AXIS2_PLACEMENT_3D('',#27101,#18918,#18919);
#17036=AXIS2_PLACEMENT_3D('',#27102,#18920,#18921);
#17037=AXIS2_PLACEMENT_3D('',#27105,#18923,#18924);
#17038=AXIS2_PLACEMENT_3D('',#27106,#18925,#18926);
#17039=AXIS2_PLACEMENT_3D('',#27108,#18927,#18928);
#17040=AXIS2_PLACEMENT_3D('',#27109,#18929,#18930);
#17041=AXIS2_PLACEMENT_3D('',#27111,#18931,#18932);
#17042=AXIS2_PLACEMENT_3D('',#27115,#18934,#18935);
#17043=AXIS2_PLACEMENT_3D('',#27116,#18936,#18937);
#17044=AXIS2_PLACEMENT_3D('',#27117,#18938,#18939);
#17045=AXIS2_PLACEMENT_3D('',#27120,#18941,#18942);
#17046=AXIS2_PLACEMENT_3D('',#27121,#18943,#18944);
#17047=AXIS2_PLACEMENT_3D('',#27263,#18945,#18946);
#17048=AXIS2_PLACEMENT_3D('',#27403,#18947,#18948);
#17049=AXIS2_PLACEMENT_3D('',#27405,#18949,#18950);
#17050=AXIS2_PLACEMENT_3D('',#27416,#18952,#18953);
#17051=AXIS2_PLACEMENT_3D('',#27423,#18954,#18955);
#17052=AXIS2_PLACEMENT_3D('',#27425,#18956,#18957);
#17053=AXIS2_PLACEMENT_3D('',#27427,#18959,#18960);
#17054=AXIS2_PLACEMENT_3D('',#27430,#18962,#18963);
#17055=AXIS2_PLACEMENT_3D('',#27431,#18964,#18965);
#17056=AXIS2_PLACEMENT_3D('',#27433,#18966,#18967);
#17057=AXIS2_PLACEMENT_3D('',#27434,#18968,#18969);
#17058=AXIS2_PLACEMENT_3D('',#27575,#18970,#18971);
#17059=AXIS2_PLACEMENT_3D('',#28282,#18972,#18973);
#17060=AXIS2_PLACEMENT_3D('',#28843,#18974,#18975);
#17061=AXIS2_PLACEMENT_3D('',#28844,#18976,#18977);
#17062=AXIS2_PLACEMENT_3D('',#29955,#18978,#18979);
#17063=AXIS2_PLACEMENT_3D('',#29957,#18980,#18981);
#17064=AXIS2_PLACEMENT_3D('',#29958,#18982,#18983);
#17065=AXIS2_PLACEMENT_3D('',#30096,#18984,#18985);
#17066=AXIS2_PLACEMENT_3D('',#30097,#18986,#18987);
#17067=AXIS2_PLACEMENT_3D('',#31063,#18988,#18989);
#17068=AXIS2_PLACEMENT_3D('',#31086,#18992,#18993);
#17069=AXIS2_PLACEMENT_3D('',#31097,#18995,#18996);
#17070=AXIS2_PLACEMENT_3D('',#31137,#18997,#18998);
#17071=AXIS2_PLACEMENT_3D('',#31138,#18999,#19000);
#17072=AXIS2_PLACEMENT_3D('',#31140,#19001,#19002);
#17073=AXIS2_PLACEMENT_3D('',#31142,#19004,#19005);
#17074=AXIS2_PLACEMENT_3D('',#31155,#19007,#19008);
#17075=AXIS2_PLACEMENT_3D('',#31170,#19011,#19012);
#17076=AXIS2_PLACEMENT_3D('',#31185,#19015,#19016);
#17077=AXIS2_PLACEMENT_3D('',#31187,#19017,#19018);
#17078=AXIS2_PLACEMENT_3D('',#31190,#19020,#19021);
#17079=AXIS2_PLACEMENT_3D('',#31191,#19022,#19023);
#17080=AXIS2_PLACEMENT_3D('',#31193,#19024,#19025);
#17081=AXIS2_PLACEMENT_3D('',#31194,#19026,#19027);
#17082=AXIS2_PLACEMENT_3D('',#31197,#19029,#19030);
#17083=AXIS2_PLACEMENT_3D('',#31198,#19031,#19032);
#17084=AXIS2_PLACEMENT_3D('',#31201,#19034,#19035);
#17085=AXIS2_PLACEMENT_3D('',#31202,#19036,#19037);
#17086=AXIS2_PLACEMENT_3D('',#31205,#19039,#19040);
#17087=AXIS2_PLACEMENT_3D('',#31206,#19041,#19042);
#17088=AXIS2_PLACEMENT_3D('',#31209,#19044,#19045);
#17089=AXIS2_PLACEMENT_3D('',#31210,#19046,#19047);
#17090=AXIS2_PLACEMENT_3D('',#31266,#19049,#19050);
#17091=AXIS2_PLACEMENT_3D('',#31298,#19051,#19052);
#17092=AXIS2_PLACEMENT_3D('',#31299,#19053,#19054);
#17093=AXIS2_PLACEMENT_3D('',#31300,#19055,#19056);
#17094=AXIS2_PLACEMENT_3D('',#31302,#19057,#19058);
#17095=AXIS2_PLACEMENT_3D('',#31305,#19060,#19061);
#17096=AXIS2_PLACEMENT_3D('',#31306,#19062,#19063);
#17097=AXIS2_PLACEMENT_3D('',#31309,#19065,#19066);
#17098=AXIS2_PLACEMENT_3D('',#31312,#19069,#19070);
#17099=AXIS2_PLACEMENT_3D('',#31313,#19071,#19072);
#17100=AXIS2_PLACEMENT_3D('',#31314,#19073,#19074);
#17101=AXIS2_PLACEMENT_3D('',#31317,#19076,#19077);
#17102=AXIS2_PLACEMENT_3D('',#31318,#19078,#19079);
#17103=AXIS2_PLACEMENT_3D('',#31320,#19080,#19081);
#17104=AXIS2_PLACEMENT_3D('',#31321,#19082,#19083);
#17105=AXIS2_PLACEMENT_3D('',#31323,#19085,#19086);
#17106=AXIS2_PLACEMENT_3D('',#31324,#19087,#19088);
#17107=AXIS2_PLACEMENT_3D('',#31325,#19089,#19090);
#17108=AXIS2_PLACEMENT_3D('',#31327,#19091,#19092);
#17109=AXIS2_PLACEMENT_3D('',#31328,#19093,#19094);
#17110=AXIS2_PLACEMENT_3D('',#31330,#19096,#19097);
#18732=DIRECTION('axis',(0.,0.,1.));
#18733=DIRECTION('refdir',(1.,0.,0.));
#18734=DIRECTION('center_axis',(1.,0.,0.));
#18735=DIRECTION('ref_axis',(0.,1.,0.));
#18736=DIRECTION('',(-1.,0.,0.));
#18737=DIRECTION('center_axis',(1.,0.,0.));
#18738=DIRECTION('ref_axis',(0.,1.,0.));
#18739=DIRECTION('center_axis',(1.,0.,0.));
#18740=DIRECTION('ref_axis',(0.,1.,0.));
#18741=DIRECTION('',(-1.,0.,0.));
#18742=DIRECTION('center_axis',(1.,0.,0.));
#18743=DIRECTION('ref_axis',(0.,1.,0.));
#18744=DIRECTION('',(-1.,0.,0.));
#18745=DIRECTION('center_axis',(1.,0.,0.));
#18746=DIRECTION('ref_axis',(0.,1.,0.));
#18747=DIRECTION('',(-1.,0.,0.));
#18748=DIRECTION('center_axis',(1.,0.,0.));
#18749=DIRECTION('ref_axis',(0.,1.,0.));
#18750=DIRECTION('',(-1.,0.,0.));
#18751=DIRECTION('center_axis',(1.,0.,0.));
#18752=DIRECTION('ref_axis',(0.,1.,0.));
#18753=DIRECTION('',(-1.,0.,0.));
#18754=DIRECTION('center_axis',(1.,0.,0.));
#18755=DIRECTION('ref_axis',(0.,1.,0.));
#18756=DIRECTION('',(-1.,0.,0.));
#18757=DIRECTION('center_axis',(1.,0.,0.));
#18758=DIRECTION('ref_axis',(0.,1.,0.));
#18759=DIRECTION('',(-1.,0.,0.));
#18760=DIRECTION('center_axis',(1.,0.,0.));
#18761=DIRECTION('ref_axis',(0.,1.,0.));
#18762=DIRECTION('',(-1.,0.,0.));
#18763=DIRECTION('center_axis',(1.,0.,0.));
#18764=DIRECTION('ref_axis',(0.,1.,0.));
#18765=DIRECTION('',(-1.,0.,0.));
#18766=DIRECTION('center_axis',(1.,0.,0.));
#18767=DIRECTION('ref_axis',(0.,1.,0.));
#18768=DIRECTION('',(-1.,0.,0.));
#18769=DIRECTION('center_axis',(1.,0.,0.));
#18770=DIRECTION('ref_axis',(0.,1.,0.));
#18771=DIRECTION('',(-1.,0.,0.));
#18772=DIRECTION('center_axis',(1.,0.,0.));
#18773=DIRECTION('ref_axis',(0.,1.,0.));
#18774=DIRECTION('',(-1.,0.,0.));
#18775=DIRECTION('center_axis',(1.,0.,0.));
#18776=DIRECTION('ref_axis',(0.,1.,0.));
#18777=DIRECTION('',(-1.,0.,0.));
#18778=DIRECTION('center_axis',(1.,0.,0.));
#18779=DIRECTION('ref_axis',(0.,1.,0.));
#18780=DIRECTION('',(-1.,0.,0.));
#18781=DIRECTION('center_axis',(1.,0.,0.));
#18782=DIRECTION('ref_axis',(0.,1.,0.));
#18783=DIRECTION('',(-1.,0.,0.));
#18784=DIRECTION('center_axis',(1.,0.,0.));
#18785=DIRECTION('ref_axis',(0.,1.,7.24992115782204E-14));
#18786=DIRECTION('',(1.,0.,0.));
#18787=DIRECTION('center_axis',(1.,0.,0.));
#18788=DIRECTION('ref_axis',(0.,1.,7.24992115782204E-14));
#18789=DIRECTION('center_axis',(1.,0.,0.));
#18790=DIRECTION('ref_axis',(0.,1.,7.24992115782204E-14));
#18791=DIRECTION('',(1.,0.,0.));
#18792=DIRECTION('center_axis',(1.,0.,0.));
#18793=DIRECTION('ref_axis',(0.,1.,7.24992115782204E-14));
#18794=DIRECTION('',(1.,0.,0.));
#18795=DIRECTION('center_axis',(1.,0.,0.));
#18796=DIRECTION('ref_axis',(0.,1.,7.24992115782204E-14));
#18797=DIRECTION('',(1.,0.,0.));
#18798=DIRECTION('center_axis',(1.,0.,0.));
#18799=DIRECTION('ref_axis',(0.,1.,7.24992115782204E-14));
#18800=DIRECTION('',(1.,0.,0.));
#18801=DIRECTION('center_axis',(1.,0.,0.));
#18802=DIRECTION('ref_axis',(0.,1.,7.24992115782204E-14));
#18803=DIRECTION('',(1.,0.,0.));
#18804=DIRECTION('center_axis',(1.,0.,0.));
#18805=DIRECTION('ref_axis',(0.,1.,7.24992115782204E-14));
#18806=DIRECTION('',(1.,0.,0.));
#18807=DIRECTION('center_axis',(1.,0.,0.));
#18808=DIRECTION('ref_axis',(0.,1.,7.24992115782204E-14));
#18809=DIRECTION('',(1.,0.,0.));
#18810=DIRECTION('center_axis',(1.,0.,0.));
#18811=DIRECTION('ref_axis',(0.,1.,7.24992115782204E-14));
#18812=DIRECTION('',(1.,0.,0.));
#18813=DIRECTION('center_axis',(1.,0.,0.));
#18814=DIRECTION('ref_axis',(0.,1.,7.24992115782204E-14));
#18815=DIRECTION('',(1.,0.,0.));
#18816=DIRECTION('center_axis',(1.,0.,0.));
#18817=DIRECTION('ref_axis',(0.,1.,7.24992115782204E-14));
#18818=DIRECTION('',(1.,0.,0.));
#18819=DIRECTION('center_axis',(1.,0.,0.));
#18820=DIRECTION('ref_axis',(0.,1.,7.24992115782204E-14));
#18821=DIRECTION('',(1.,0.,0.));
#18822=DIRECTION('center_axis',(1.,0.,0.));
#18823=DIRECTION('ref_axis',(0.,1.,7.24992115782204E-14));
#18824=DIRECTION('',(1.,0.,0.));
#18825=DIRECTION('center_axis',(1.,0.,0.));
#18826=DIRECTION('ref_axis',(0.,1.,7.24992115782204E-14));
#18827=DIRECTION('',(1.,0.,0.));
#18828=DIRECTION('center_axis',(1.,0.,0.));
#18829=DIRECTION('ref_axis',(0.,1.,7.24992115782204E-14));
#18830=DIRECTION('',(1.,0.,0.));
#18831=DIRECTION('center_axis',(1.,0.,0.));
#18832=DIRECTION('ref_axis',(0.,1.,0.));
#18833=DIRECTION('',(-1.,0.,0.));
#18834=DIRECTION('center_axis',(-1.,0.,0.));
#18835=DIRECTION('ref_axis',(0.,1.,0.));
#18836=DIRECTION('center_axis',(1.,0.,0.));
#18837=DIRECTION('ref_axis',(0.,1.,0.));
#18838=DIRECTION('',(-1.,0.,0.));
#18839=DIRECTION('center_axis',(1.,0.,0.));
#18840=DIRECTION('ref_axis',(0.,1.,0.));
#18841=DIRECTION('',(-1.,0.,0.));
#18842=DIRECTION('center_axis',(1.,0.,0.));
#18843=DIRECTION('ref_axis',(0.,1.,0.));
#18844=DIRECTION('',(-1.,0.,0.));
#18845=DIRECTION('center_axis',(1.,0.,0.));
#18846=DIRECTION('ref_axis',(0.,1.,0.));
#18847=DIRECTION('',(-1.,0.,0.));
#18848=DIRECTION('center_axis',(1.,0.,0.));
#18849=DIRECTION('ref_axis',(0.,1.,0.));
#18850=DIRECTION('',(-1.,0.,0.));
#18851=DIRECTION('center_axis',(1.,0.,0.));
#18852=DIRECTION('ref_axis',(0.,1.,0.));
#18853=DIRECTION('',(-1.,0.,0.));
#18854=DIRECTION('center_axis',(1.,0.,0.));
#18855=DIRECTION('ref_axis',(0.,1.,0.));
#18856=DIRECTION('',(-1.,0.,0.));
#18857=DIRECTION('center_axis',(1.,0.,0.));
#18858=DIRECTION('ref_axis',(0.,1.,0.));
#18859=DIRECTION('',(-1.,0.,0.));
#18860=DIRECTION('center_axis',(1.,0.,0.));
#18861=DIRECTION('ref_axis',(0.,1.,0.));
#18862=DIRECTION('',(-1.,0.,0.));
#18863=DIRECTION('center_axis',(1.,0.,0.));
#18864=DIRECTION('ref_axis',(0.,1.,0.));
#18865=DIRECTION('',(-1.,0.,0.));
#18866=DIRECTION('center_axis',(-1.,0.,0.));
#18867=DIRECTION('ref_axis',(0.,1.,0.));
#18868=DIRECTION('center_axis',(1.,0.,0.));
#18869=DIRECTION('ref_axis',(0.,0.100102849209394,-0.994977095002775));
#18870=DIRECTION('',(1.,0.,0.));
#18871=DIRECTION('center_axis',(1.,0.,0.));
#18872=DIRECTION('ref_axis',(0.,1.,4.89925865752541E-14));
#18873=DIRECTION('center_axis',(1.,0.,0.));
#18874=DIRECTION('ref_axis',(0.,1.,4.89925865752541E-14));
#18875=DIRECTION('',(1.,0.,0.));
#18876=DIRECTION('center_axis',(1.,0.,0.));
#18877=DIRECTION('ref_axis',(0.,1.,4.89925865752541E-14));
#18878=DIRECTION('',(1.,0.,0.));
#18879=DIRECTION('center_axis',(1.,0.,0.));
#18880=DIRECTION('ref_axis',(0.,1.,4.89925865752541E-14));
#18881=DIRECTION('',(1.,0.,0.));
#18882=DIRECTION('center_axis',(1.,0.,0.));
#18883=DIRECTION('ref_axis',(0.,1.,4.89925865752541E-14));
#18884=DIRECTION('',(1.,0.,0.));
#18885=DIRECTION('center_axis',(1.,0.,0.));
#18886=DIRECTION('ref_axis',(0.,1.,4.89925865752541E-14));
#18887=DIRECTION('',(1.,0.,0.));
#18888=DIRECTION('center_axis',(1.,0.,0.));
#18889=DIRECTION('ref_axis',(0.,1.,4.89925865752541E-14));
#18890=DIRECTION('',(1.,0.,0.));
#18891=DIRECTION('center_axis',(1.,0.,0.));
#18892=DIRECTION('ref_axis',(0.,1.,4.89925865752541E-14));
#18893=DIRECTION('',(1.,0.,0.));
#18894=DIRECTION('center_axis',(1.,0.,0.));
#18895=DIRECTION('ref_axis',(0.,1.,4.89925865752541E-14));
#18896=DIRECTION('',(1.,0.,0.));
#18897=DIRECTION('center_axis',(1.,0.,0.));
#18898=DIRECTION('ref_axis',(0.,1.,4.89925865752541E-14));
#18899=DIRECTION('',(1.,0.,0.));
#18900=DIRECTION('center_axis',(-1.,0.,0.));
#18901=DIRECTION('ref_axis',(0.,-1.,0.));
#18902=DIRECTION('center_axis',(-1.,0.,0.));
#18903=DIRECTION('ref_axis',(0.,-1.,0.));
#18904=DIRECTION('',(0.707106781186553,-0.707106781186542,8.65956056235487E-17));
#18905=DIRECTION('center_axis',(1.,0.,0.));
#18906=DIRECTION('ref_axis',(0.,-1.,0.));
#18907=DIRECTION('center_axis',(1.,0.,0.));
#18908=DIRECTION('ref_axis',(0.,-1.,0.));
#18909=DIRECTION('center_axis',(1.,0.,0.));
#18910=DIRECTION('ref_axis',(0.,1.,0.));
#18911=DIRECTION('center_axis',(-1.,0.,0.));
#18912=DIRECTION('ref_axis',(0.,-1.,0.));
#18913=DIRECTION('center_axis',(-1.,0.,0.));
#18914=DIRECTION('ref_axis',(0.,-1.,0.));
#18915=DIRECTION('',(-1.,0.,0.));
#18916=DIRECTION('center_axis',(-1.,0.,0.));
#18917=DIRECTION('ref_axis',(0.,0.,1.));
#18918=DIRECTION('center_axis',(1.,0.,0.));
#18919=DIRECTION('ref_axis',(0.,0.,-1.));
#18920=DIRECTION('center_axis',(1.,0.,0.));
#18921=DIRECTION('ref_axis',(0.,-1.,0.));
#18922=DIRECTION('',(0.707106781186553,0.707106781186542,-8.65956056235487E-17));
#18923=DIRECTION('center_axis',(1.,0.,0.));
#18924=DIRECTION('ref_axis',(0.,-1.,0.));
#18925=DIRECTION('center_axis',(1.,0.,0.));
#18926=DIRECTION('ref_axis',(0.,0.,-1.));
#18927=DIRECTION('center_axis',(1.,0.,0.));
#18928=DIRECTION('ref_axis',(0.,0.,-1.));
#18929=DIRECTION('center_axis',(-1.,0.,-4.39101262113484E-15));
#18930=DIRECTION('ref_axis',(0.,-1.,-3.11403559978336E-17));
#18931=DIRECTION('center_axis',(-1.,0.,0.));
#18932=DIRECTION('ref_axis',(0.,-1.,0.));
#18933=DIRECTION('',(-0.382683432365094,0.923879532511285,-1.53845523264404E-15));
#18934=DIRECTION('center_axis',(1.,0.,0.));
#18935=DIRECTION('ref_axis',(0.,-1.,-6.12323399573677E-17));
#18936=DIRECTION('center_axis',(1.,0.,0.));
#18937=DIRECTION('ref_axis',(0.,-1.,-6.12323399573677E-17));
#18938=DIRECTION('center_axis',(-1.,0.,0.));
#18939=DIRECTION('ref_axis',(0.,1.,0.));
#18940=DIRECTION('',(-0.707106781186546,-0.707106781186549,-8.65956056235495E-17));
#18941=DIRECTION('center_axis',(1.,0.,0.));
#18942=DIRECTION('ref_axis',(0.,0.,-1.));
#18943=DIRECTION('center_axis',(1.,0.,0.));
#18944=DIRECTION('ref_axis',(0.,0.,-1.));
#18945=DIRECTION('center_axis',(-1.,0.,0.));
#18946=DIRECTION('ref_axis',(0.,1.,4.89925865752541E-14));
#18947=DIRECTION('center_axis',(0.,6.92018220157551E-16,-1.));
#18948=DIRECTION('ref_axis',(1.,3.00652077147108E-17,0.));
#18949=DIRECTION('center_axis',(-5.63785247977654E-32,9.20731182852366E-16,
-1.));
#18950=DIRECTION('ref_axis',(1.,6.12323399573677E-17,0.));
#18951=DIRECTION('',(-0.382683432365095,5.80970808792151E-16,-0.923879532511284));
#18952=DIRECTION('center_axis',(0.,0.,1.));
#18953=DIRECTION('ref_axis',(1.,0.,0.));
#18954=DIRECTION('center_axis',(0.,0.,-1.));
#18955=DIRECTION('ref_axis',(1.,0.,0.));
#18956=DIRECTION('center_axis',(-2.84633584564593E-32,4.64841919748234E-16,
1.));
#18957=DIRECTION('ref_axis',(1.,6.12323399573677E-17,0.));
#18958=DIRECTION('',(-0.707106781186547,-8.65956056235493E-17,-0.707106781186547));
#18959=DIRECTION('center_axis',(0.,-1.65459148343064E-15,-1.));
#18960=DIRECTION('ref_axis',(1.,3.20478109930714E-17,0.));
#18961=DIRECTION('',(0.923879532511284,5.49650453450813E-16,0.382683432365097));
#18962=DIRECTION('center_axis',(0.,0.,-1.));
#18963=DIRECTION('ref_axis',(1.,0.,0.));
#18964=DIRECTION('center_axis',(0.,0.,1.));
#18965=DIRECTION('ref_axis',(1.,0.,0.));
#18966=DIRECTION('center_axis',(0.,0.,1.));
#18967=DIRECTION('ref_axis',(1.,0.,0.));
#18968=DIRECTION('center_axis',(1.,0.,0.));
#18969=DIRECTION('ref_axis',(0.,0.,-1.));
#18970=DIRECTION('center_axis',(-1.,0.,0.));
#18971=DIRECTION('ref_axis',(0.,1.,0.));
#18972=DIRECTION('center_axis',(1.,0.,0.));
#18973=DIRECTION('ref_axis',(0.,1.,4.89925865752541E-14));
#18974=DIRECTION('center_axis',(1.,0.,0.));
#18975=DIRECTION('ref_axis',(0.,1.,0.));
#18976=DIRECTION('center_axis',(-1.,0.,0.));
#18977=DIRECTION('ref_axis',(0.,1.,0.));
#18978=DIRECTION('center_axis',(1.,0.,0.));
#18979=DIRECTION('ref_axis',(0.,0.,-1.));
#18980=DIRECTION('center_axis',(1.,0.,0.));
#18981=DIRECTION('ref_axis',(0.,1.,0.));
#18982=DIRECTION('center_axis',(1.,0.,0.));
#18983=DIRECTION('ref_axis',(0.,1.,0.));
#18984=DIRECTION('center_axis',(-1.,0.,0.));
#18985=DIRECTION('ref_axis',(0.,1.,7.24992115782204E-14));
#18986=DIRECTION('center_axis',(1.,0.,0.));
#18987=DIRECTION('ref_axis',(0.,0.888973712533679,0.45795822781569));
#18988=DIRECTION('center_axis',(0.,0.,1.));
#18989=DIRECTION('ref_axis',(-0.707106781186561,0.707106781186534,0.));
#18990=DIRECTION('',(0.,0.,-1.));
#18991=DIRECTION('',(0.,0.,1.));
#18992=DIRECTION('center_axis',(0.,1.,0.));
#18993=DIRECTION('ref_axis',(-1.,0.,6.34413156928661E-16));
#18994=DIRECTION('',(0.,1.,0.));
#18995=DIRECTION('center_axis',(0.,1.,0.));
#18996=DIRECTION('ref_axis',(-1.,0.,6.34413156928661E-16));
#18997=DIRECTION('center_axis',(0.,1.,0.));
#18998=DIRECTION('ref_axis',(-1.,0.,6.34413156928661E-16));
#18999=DIRECTION('center_axis',(-1.,0.,0.));
#19000=DIRECTION('ref_axis',(0.,0.,1.));
#19001=DIRECTION('center_axis',(-1.,0.,0.));
#19002=DIRECTION('ref_axis',(0.,1.,0.));
#19003=DIRECTION('',(0.,0.,-1.));
#19004=DIRECTION('center_axis',(0.,0.,-1.));
#19005=DIRECTION('ref_axis',(-0.707106781186561,-0.707106781186534,0.));
#19006=DIRECTION('',(0.,0.,1.));
#19007=DIRECTION('center_axis',(0.,0.,1.));
#19008=DIRECTION('ref_axis',(0.995170161956952,0.0981649059011095,0.));
#19009=DIRECTION('',(0.,0.,1.));
#19010=DIRECTION('',(0.,0.,-1.));
#19011=DIRECTION('center_axis',(0.,0.,-1.));
#19012=DIRECTION('ref_axis',(0.995170161956952,-0.0981649059011095,0.));
#19013=DIRECTION('',(0.,0.,-1.));
#19014=DIRECTION('',(0.,0.,1.));
#19015=DIRECTION('center_axis',(0.,-1.,0.));
#19016=DIRECTION('ref_axis',(1.,0.,0.));
#19017=DIRECTION('center_axis',(0.,-1.,0.));
#19018=DIRECTION('ref_axis',(1.,0.,0.));
#19019=DIRECTION('',(0.70710678118654,0.707106781186555,8.65956056235484E-17));
#19020=DIRECTION('center_axis',(0.,1.,0.));
#19021=DIRECTION('ref_axis',(1.,0.,0.));
#19022=DIRECTION('center_axis',(0.,1.,0.));
#19023=DIRECTION('ref_axis',(1.,0.,0.));
#19024=DIRECTION('center_axis',(0.,1.,0.));
#19025=DIRECTION('ref_axis',(1.,0.,0.));
#19026=DIRECTION('center_axis',(0.,1.,0.));
#19027=DIRECTION('ref_axis',(1.,0.,0.));
#19028=DIRECTION('',(0.,1.,0.));
#19029=DIRECTION('center_axis',(0.,1.,0.));
#19030=DIRECTION('ref_axis',(1.,0.,0.));
#19031=DIRECTION('center_axis',(0.,0.,1.));
#19032=DIRECTION('ref_axis',(1.,0.,0.));
#19033=DIRECTION('',(0.70710678118654,8.65956056235484E-17,-0.707106781186555));
#19034=DIRECTION('center_axis',(0.,0.,-1.));
#19035=DIRECTION('ref_axis',(1.,0.,0.));
#19036=DIRECTION('center_axis',(0.,0.,-1.));
#19037=DIRECTION('ref_axis',(1.,0.,0.));
#19038=DIRECTION('',(0.,0.,-1.));
#19039=DIRECTION('center_axis',(0.,0.,-1.));
#19040=DIRECTION('ref_axis',(1.,0.,0.));
#19041=DIRECTION('center_axis',(0.,1.,0.));
#19042=DIRECTION('ref_axis',(1.,0.,0.));
#19043=DIRECTION('',(-0.707106781186548,0.707106781186548,-8.65956056235493E-17));
#19044=DIRECTION('center_axis',(0.,-1.,0.));
#19045=DIRECTION('ref_axis',(1.,0.,0.));
#19046=DIRECTION('center_axis',(0.,-1.,0.));
#19047=DIRECTION('ref_axis',(1.,0.,0.));
#19048=DIRECTION('',(0.,1.,0.));
#19049=DIRECTION('center_axis',(0.,0.,1.));
#19050=DIRECTION('ref_axis',(1.,0.,0.));
#19051=DIRECTION('center_axis',(0.,1.,0.));
#19052=DIRECTION('ref_axis',(1.,0.,0.));
#19053=DIRECTION('center_axis',(0.,0.,1.));
#19054=DIRECTION('ref_axis',(1.,0.,0.));
#19055=DIRECTION('center_axis',(0.,1.,0.));
#19056=DIRECTION('ref_axis',(1.,0.,0.));
#19057=DIRECTION('center_axis',(0.,1.,0.));
#19058=DIRECTION('ref_axis',(1.,0.,0.));
#19059=DIRECTION('',(0.,1.,0.));
#19060=DIRECTION('center_axis',(0.,-1.,0.));
#19061=DIRECTION('ref_axis',(1.,0.,0.));
#19062=DIRECTION('center_axis',(1.,0.,0.));
#19063=DIRECTION('ref_axis',(0.,1.,0.));
#19064=DIRECTION('',(-1.,0.,0.));
#19065=DIRECTION('center_axis',(1.,0.,0.));
#19066=DIRECTION('ref_axis',(0.,0.,-1.));
#19067=DIRECTION('',(-1.,0.,0.));
#19068=DIRECTION('',(1.,0.,0.));
#19069=DIRECTION('center_axis',(0.,1.,0.));
#19070=DIRECTION('ref_axis',(1.,0.,0.));
#19071=DIRECTION('center_axis',(0.,1.,0.));
#19072=DIRECTION('ref_axis',(1.,0.,0.));
#19073=DIRECTION('center_axis',(1.,0.,0.));
#19074=DIRECTION('ref_axis',(0.,1.,0.));
#19075=DIRECTION('',(-1.,0.,0.));
#19076=DIRECTION('center_axis',(1.,0.,0.));
#19077=DIRECTION('ref_axis',(0.,0.,-1.));
#19078=DIRECTION('center_axis',(-1.,0.,0.));
#19079=DIRECTION('ref_axis',(0.,0.,1.));
#19080=DIRECTION('center_axis',(1.,0.,0.));
#19081=DIRECTION('ref_axis',(0.,0.,-1.));
#19082=DIRECTION('center_axis',(1.,0.,0.));
#19083=DIRECTION('ref_axis',(0.,1.,0.));
#19084=DIRECTION('',(-0.707106781186548,0.707106781186548,8.65956056235493E-17));
#19085=DIRECTION('center_axis',(1.,0.,0.));
#19086=DIRECTION('ref_axis',(0.,-0.488782589557792,-0.872405628217276));
#19087=DIRECTION('center_axis',(1.,0.,0.));
#19088=DIRECTION('ref_axis',(0.,1.,0.));
#19089=DIRECTION('center_axis',(-1.,0.,0.));
#19090=DIRECTION('ref_axis',(0.,0.,1.));
#19091=DIRECTION('center_axis',(1.,0.,0.));
#19092=DIRECTION('ref_axis',(0.,0.,-1.));
#19093=DIRECTION('center_axis',(1.,0.,0.));
#19094=DIRECTION('ref_axis',(0.,1.,0.));
#19095=DIRECTION('',(-0.707106781186552,0.707106781186543,8.65956056235488E-17));
#19096=DIRECTION('center_axis',(-1.,0.,0.));
#19097=DIRECTION('ref_axis',(0.,1.,0.));
#19098=DIRECTION('',(-0.707106781186555,-0.70710678118654,-8.65956056235484E-17));
#23909=CARTESIAN_POINT('',(0.,0.,0.));
#23910=CARTESIAN_POINT('Origin',(80.4,0.,0.));
#23911=CARTESIAN_POINT('',(69.2061568471518,-20.9251045326925,0.000537903476663659));
#23912=CARTESIAN_POINT('',(68.9938431528481,-20.9246928645182,0.000347110336330147));
#23913=CARTESIAN_POINT('',(80.4,-20.925,-2.56257342721584E-15));
#23914=CARTESIAN_POINT('',(68.725,9.00143038127672,18.8903144283542));
#23915=CARTESIAN_POINT('Ctrl Pts',(69.2061568471518,-20.9251045326925,0.000537903476663659));
#23916=CARTESIAN_POINT('Ctrl Pts',(69.1973932851687,-20.925892267353,0.768641798467955));
#23917=CARTESIAN_POINT('Ctrl Pts',(69.1886297231856,-20.8844127756245,1.53666082027718));
#23918=CARTESIAN_POINT('Ctrl Pts',(69.1798661612025,-20.8000149036333,2.29993382021793));
#23919=CARTESIAN_POINT('Ctrl Pts',(69.140247873288,-20.4184692263878,5.75053638654726));
#23920=CARTESIAN_POINT('Ctrl Pts',(69.1006295853734,-19.1597744826372,9.10414161453262));
#23921=CARTESIAN_POINT('Ctrl Pts',(69.0610112974588,-17.1767275083919,11.9536689002946));
#23922=CARTESIAN_POINT('Ctrl Pts',(69.0213930095442,-15.1936805341465,14.8031961860566));
#23923=CARTESIAN_POINT('Ctrl Pts',(68.9817747216296,-12.4862813294065,17.1486455295952));
#23924=CARTESIAN_POINT('Ctrl Pts',(68.9421564337151,-9.38318674595559,18.7052533021947));
#23925=CARTESIAN_POINT('Ctrl Pts',(68.9025381458005,-6.28009216250464,20.2618610747941));
#23926=CARTESIAN_POINT('Ctrl Pts',(68.8629198578859,-2.7813022003428,21.0296272764544));
#23927=CARTESIAN_POINT('Ctrl Pts',(68.8233015699713,0.688453527214973,20.9154363519887));
#23928=CARTESIAN_POINT('Ctrl Pts',(68.7905343799809,3.55819250711376,20.8209921971777));
#23929=CARTESIAN_POINT('Ctrl Pts',(68.7577671899904,6.40807065798892,20.1232464597002));
#23930=CARTESIAN_POINT('Ctrl Pts',(68.725,9.00178625489531,18.890518144815));
#23931=CARTESIAN_POINT('',(68.725,-9.00107450765889,18.890110711893));
#23932=CARTESIAN_POINT('Origin',(68.725,0.,0.));
#23933=CARTESIAN_POINT('Ctrl Pts',(68.725,-9.0010745076589,18.890110711893));
#23934=CARTESIAN_POINT('Ctrl Pts',(68.7646182879146,-12.1359393145908,17.3963581273268));
#23935=CARTESIAN_POINT('Ctrl Pts',(68.8042365758292,-14.8902410183971,15.1079808431403));
#23936=CARTESIAN_POINT('Ctrl Pts',(68.8438548637437,-16.9306635496692,12.2997765477629));
#23937=CARTESIAN_POINT('Ctrl Pts',(68.8834731516583,-18.9710860809414,9.49157225238549));
#23938=CARTESIAN_POINT('Ctrl Pts',(68.9230914395729,-20.2976294396793,6.16354094581719));
#23939=CARTESIAN_POINT('Ctrl Pts',(68.9627097274875,-20.7491077747907,2.72122018983935));
#23940=CARTESIAN_POINT('Ctrl Pts',(68.973087535941,-20.8673702219923,1.81952182472461));
#23941=CARTESIAN_POINT('Ctrl Pts',(68.9834653443946,-20.9255899684262,0.909981474127051));
#23942=CARTESIAN_POINT('Ctrl Pts',(68.9938431528481,-20.9246928645182,0.000347110336330147));
#23943=CARTESIAN_POINT('Origin',(80.4,0.,0.));
#23944=CARTESIAN_POINT('',(70.7061568471518,-20.9257818388602,-0.000467423370275055));
#23945=CARTESIAN_POINT('',(70.4938431528481,-20.9261779264193,-0.000381460781396608));
#23946=CARTESIAN_POINT('',(80.4,-20.925,-2.56257342721584E-15));
#23947=CARTESIAN_POINT('Ctrl Pts',(70.7061568471518,-20.9257818388602,-0.000467423370275055));
#23948=CARTESIAN_POINT('Ctrl Pts',(70.6728127401437,-20.9229483509825,2.92178557156433));
#23949=CARTESIAN_POINT('Ctrl Pts',(70.6394686331356,-20.3051998739425,5.84519881683506));
#23950=CARTESIAN_POINT('Ctrl Pts',(70.6061245261274,-19.1164161743571,8.51427815820994));
#23951=CARTESIAN_POINT('Ctrl Pts',(70.5665062382128,-17.7039454530144,11.6855837741494));
#23952=CARTESIAN_POINT('Ctrl Pts',(70.5268879502982,-15.4853242409376,14.4978372802698));
#23953=CARTESIAN_POINT('Ctrl Pts',(70.4872696623837,-12.7298766583704,16.6096520162404));
#23954=CARTESIAN_POINT('Ctrl Pts',(70.4476513744691,-9.97442907580324,18.7214667522109));
#23955=CARTESIAN_POINT('Ctrl Pts',(70.4080330865545,-6.68215512274561,20.1328427180316));
#23956=CARTESIAN_POINT('Ctrl Pts',(70.3684147986399,-3.25271237917639,20.6724493517347));
#23957=CARTESIAN_POINT('Ctrl Pts',(70.3287965107253,0.176730364392844,21.2120559854378));
#23958=CARTESIAN_POINT('Ctrl Pts',(70.2891782228108,3.74334189847368,20.8798932870233));
#23959=CARTESIAN_POINT('Ctrl Pts',(70.2495599348962,7.01416209926513,19.7162833642022));
#23960=CARTESIAN_POINT('Ctrl Pts',(70.2099416469816,10.2849823000566,18.5526734413812));
#23961=CARTESIAN_POINT('Ctrl Pts',(70.170323359067,13.2600111675587,16.5576162941535));
#23962=CARTESIAN_POINT('Ctrl Pts',(70.1307050711524,15.5781023176152,13.9732969767378));
#23963=CARTESIAN_POINT('Ctrl Pts',(70.0910867832378,17.8961934676717,11.3889776593222));
#23964=CARTESIAN_POINT('Ctrl Pts',(70.0514684953233,19.5573469002827,8.21539617171875));
#23965=CARTESIAN_POINT('Ctrl Pts',(70.0118502074087,20.3599109362165,4.83780181075189));
#23966=CARTESIAN_POINT('Ctrl Pts',(69.9722319194941,21.1624749721504,1.46020744978499));
#23967=CARTESIAN_POINT('Ctrl Pts',(69.9326136315796,21.1064496114072,-2.12139978454527));
#23968=CARTESIAN_POINT('Ctrl Pts',(69.892995343665,20.1986359219932,-5.47223959788331));
#23969=CARTESIAN_POINT('Ctrl Pts',(69.8533770557504,19.2908222325792,-8.82307941122133));
#23970=CARTESIAN_POINT('Ctrl Pts',(69.8137587678358,17.5312202144946,-11.9431518035671));
#23971=CARTESIAN_POINT('Ctrl Pts',(69.7741404799212,15.1334324590649,-14.4537028000153));
#23972=CARTESIAN_POINT('Ctrl Pts',(69.7345221920066,12.7356447036353,-16.9642537964634));
#23973=CARTESIAN_POINT('Ctrl Pts',(69.6949039040921,9.6996712108608,-18.8652833970139));
#23974=CARTESIAN_POINT('Ctrl Pts',(69.6552856161775,6.39405661300567,-19.926021496295));
#23975=CARTESIAN_POINT('Ctrl Pts',(69.6156673282629,3.08844201515051,-20.9867595955761));
#23976=CARTESIAN_POINT('Ctrl Pts',(69.5760490403483,-0.486813687785254,
-21.2072061935878));
#23977=CARTESIAN_POINT('Ctrl Pts',(69.5364307524337,-3.89770107861504,-20.5605992296267));
#23978=CARTESIAN_POINT('Ctrl Pts',(69.4968124645191,-7.3085884694448,-19.9139922656657));
#23979=CARTESIAN_POINT('Ctrl Pts',(69.4571941766046,-10.5551075481686,-18.400331739732));
#23980=CARTESIAN_POINT('Ctrl Pts',(69.41757588869,-13.2431549501084,-16.2033677003751));
#23981=CARTESIAN_POINT('Ctrl Pts',(69.3779576007755,-15.9312023520481,-14.0064036610182));
#23982=CARTESIAN_POINT('Ctrl Pts',(69.3383393128609,-18.0607780772039,-11.126136108238));
#23983=CARTESIAN_POINT('Ctrl Pts',(69.2987210249463,-19.3733676344116,-7.91220237951135));
#23984=CARTESIAN_POINT('Ctrl Pts',(69.2678662990148,-20.3956124910162,-5.40919052358253));
#23985=CARTESIAN_POINT('Ctrl Pts',(69.2370115730833,-20.922331078576,-2.70380026547276));
#23986=CARTESIAN_POINT('Ctrl Pts',(69.2061568471518,-20.9251045326925,0.000537903476663659));
#23987=CARTESIAN_POINT('Ctrl Pts',(68.9938431528481,-20.9246928645182,0.000347110336330147));
#23988=CARTESIAN_POINT('Ctrl Pts',(69.0230836323092,-20.9221651874547,-2.56263572467314));
#23989=CARTESIAN_POINT('Ctrl Pts',(69.0523241117702,-20.4503176146989,-5.1263649164617));
#23990=CARTESIAN_POINT('Ctrl Pts',(69.0815645912312,-19.5298600150513,-7.51753008448147));
#23991=CARTESIAN_POINT('Ctrl Pts',(69.1211828791458,-18.2827206087156,-10.7573493974371));
#23992=CARTESIAN_POINT('Ctrl Pts',(69.1608011670604,-16.2120284845591,-13.6803778179609));
#23993=CARTESIAN_POINT('Ctrl Pts',(69.2004194549749,-13.5691025042824,-15.9314525116625));
#23994=CARTESIAN_POINT('Ctrl Pts',(69.2400377428895,-10.9261765240057,-18.1825272053641));
#23995=CARTESIAN_POINT('Ctrl Pts',(69.2796560308041,-7.71101668760872,-19.7616481722434));
#23996=CARTESIAN_POINT('Ctrl Pts',(69.3192743187187,-4.31394387820961,-20.4772883046503));
#23997=CARTESIAN_POINT('Ctrl Pts',(69.3588926066333,-0.916871068810491,
-21.1929284370572));
#23998=CARTESIAN_POINT('Ctrl Pts',(69.3985108945478,2.66211471359076,-21.0450877349916));
#23999=CARTESIAN_POINT('Ctrl Pts',(69.4381291824624,5.98856361433238,-20.0516283795423));
#24000=CARTESIAN_POINT('Ctrl Pts',(69.477747470377,9.31501251507399,-19.0581690240929));
#24001=CARTESIAN_POINT('Ctrl Pts',(69.5173657582916,12.388924534156,-17.2190910152599));
#24002=CARTESIAN_POINT('Ctrl Pts',(69.5569840462062,14.8371432934536,-14.7576877650994));
#24003=CARTESIAN_POINT('Ctrl Pts',(69.5966023341207,17.2853620527513,-12.2962845149389));
#24004=CARTESIAN_POINT('Ctrl Pts',(69.6362206220353,19.1078875522646,-9.21255602345092));
#24005=CARTESIAN_POINT('Ctrl Pts',(69.6758389099499,20.0834819577218,-5.88082212359926));
#24006=CARTESIAN_POINT('Ctrl Pts',(69.7154571978645,21.059076363179,-2.54908822374764));
#24007=CARTESIAN_POINT('Ctrl Pts',(69.755075485779,21.1877396745801,1.03065108446768));
#24008=CARTESIAN_POINT('Ctrl Pts',(69.7946937736936,20.4538514891497,4.42383093525681));
#24009=CARTESIAN_POINT('Ctrl Pts',(69.8343120616082,19.7199633037193,7.81701078604597));
#24010=CARTESIAN_POINT('Ctrl Pts',(69.8739303495228,18.1235236214575,11.0236311794089));
#24011=CARTESIAN_POINT('Ctrl Pts',(69.9135486374374,15.8583291813194,13.6544379008176));
#24012=CARTESIAN_POINT('Ctrl Pts',(69.953166925352,13.5931347411813,16.2852446222263));
#24013=CARTESIAN_POINT('Ctrl Pts',(69.9927852132666,10.659185543167,18.3402376716807));
#24014=CARTESIAN_POINT('Ctrl Pts',(70.0324035011811,7.41264078387936,19.5699532923244));
#24015=CARTESIAN_POINT('Ctrl Pts',(70.0720217890957,4.1660960245917,20.7996689129682));
#24016=CARTESIAN_POINT('Ctrl Pts',(70.1116400770103,0.606955704030666,21.2041071048013));
#24017=CARTESIAN_POINT('Ctrl Pts',(70.1512583649248,-2.8327267895864,20.7341735427668));
#24018=CARTESIAN_POINT('Ctrl Pts',(70.1908766528394,-6.27240928320346,20.2642399807324));
#24019=CARTESIAN_POINT('Ctrl Pts',(70.230494940754,-9.59263394987655,18.9199346648303));
#24020=CARTESIAN_POINT('Ctrl Pts',(70.2701132286686,-12.3903503097503,16.864445520801));
#24021=CARTESIAN_POINT('Ctrl Pts',(70.3097315165832,-15.1880666696241,14.8089563767717));
#24022=CARTESIAN_POINT('Ctrl Pts',(70.3493498044977,-17.4632747226986,12.0422834046151));
#24023=CARTESIAN_POINT('Ctrl Pts',(70.3889680924123,-18.9397810715315,8.90028051227176));
#24024=CARTESIAN_POINT('Ctrl Pts',(70.4239264458909,-20.2426195729629,6.12784249127099));
#24025=CARTESIAN_POINT('Ctrl Pts',(70.4588847993695,-20.9235944663035,3.06317519724849));
#24026=CARTESIAN_POINT('Ctrl Pts',(70.4938431528481,-20.9261779264193,-0.000381460781396608));
#24027=CARTESIAN_POINT('Origin',(80.4,0.,0.));
#24028=CARTESIAN_POINT('',(72.2061568471519,-20.9232657042053,0.000120932580692235));
#24029=CARTESIAN_POINT('',(71.9938431528481,-20.923224691771,-9.04407733959185E-6));
#24030=CARTESIAN_POINT('',(80.4,-20.925,-2.56257342721584E-15));
#24031=CARTESIAN_POINT('Ctrl Pts',(72.2061568471519,-20.9232657042053,0.000120932580692235));
#24032=CARTESIAN_POINT('Ctrl Pts',(72.1878504830332,-20.9235905266545,1.6050316355066));
#24033=CARTESIAN_POINT('Ctrl Pts',(72.1695441189146,-20.7412699845247,3.20986972041554));
#24034=CARTESIAN_POINT('Ctrl Pts',(72.151237754796,-20.3754940092624,4.77174431109023));
#24035=CARTESIAN_POINT('Ctrl Pts',(72.1116194668814,-19.5838885431924,8.15192383875766));
#24036=CARTESIAN_POINT('Ctrl Pts',(72.0720011789668,-17.9330365351294,11.3308761079985));
#24037=CARTESIAN_POINT('Ctrl Pts',(72.0323828910522,-15.6233391450283,13.9226999483342));
#24038=CARTESIAN_POINT('Ctrl Pts',(71.9927646031376,-13.3136417549272,16.5145237886699));
#24039=CARTESIAN_POINT('Ctrl Pts',(71.9531463152231,-10.3450989827881,18.5192192001004));
#24040=CARTESIAN_POINT('Ctrl Pts',(71.9135280273085,-7.07806985050165,19.693431064274));
#24041=CARTESIAN_POINT('Ctrl Pts',(71.8739097393939,-3.81104071821527,20.8676429284476));
#24042=CARTESIAN_POINT('Ctrl Pts',(71.8342914514793,-0.245525225781651,
21.2113712453643));
#24043=CARTESIAN_POINT('Ctrl Pts',(71.7946731635647,3.1856495550627,20.6828899529123));
#24044=CARTESIAN_POINT('Ctrl Pts',(71.7550548756502,6.61682433590708,20.1544086604602));
#24045=CARTESIAN_POINT('Ctrl Pts',(71.7154365877356,9.91365840516219,18.7537177586395));
#24046=CARTESIAN_POINT('Ctrl Pts',(71.675818299821,12.6759406182611,16.650850709023));
#24047=CARTESIAN_POINT('Ctrl Pts',(71.6362000119064,15.43822283136,14.5479836594065));
#24048=CARTESIAN_POINT('Ctrl Pts',(71.5965817239918,17.6659531883027,11.7429404619943));
#24049=CARTESIAN_POINT('Ctrl Pts',(71.5569634360773,19.0887017865803,8.57623250588363));
#24050=CARTESIAN_POINT('Ctrl Pts',(71.5173451481627,20.511450384858,5.40952454977299));
#24051=CARTESIAN_POINT('Ctrl Pts',(71.4777268602481,21.1292172244705,1.88115183496394));
#24052=CARTESIAN_POINT('Ctrl Pts',(71.4381085723336,20.8670100040871,-1.58056742383));
#24053=CARTESIAN_POINT('Ctrl Pts',(71.398490284419,20.6048027837037,-5.04228668262394));
#24054=CARTESIAN_POINT('Ctrl Pts',(71.3588719965044,19.4626215033242,-8.43735248540277));
#24055=CARTESIAN_POINT('Ctrl Pts',(71.3192537085898,17.5791184784511,-11.3536290855461));
#24056=CARTESIAN_POINT('Ctrl Pts',(71.2796354206752,15.695615453578,-14.2699056856894));
#24057=CARTESIAN_POINT('Ctrl Pts',(71.2400171327607,13.0707906842112,-16.7073930831972));
#24058=CARTESIAN_POINT('Ctrl Pts',(71.2003988448461,10.0232783821906,-18.3701984302307));
#24059=CARTESIAN_POINT('Ctrl Pts',(71.1607805569315,6.97576608016998,-20.0330037772643));
#24060=CARTESIAN_POINT('Ctrl Pts',(71.1211622690169,3.50556624549558,-20.9211270738236));
#24061=CARTESIAN_POINT('Ctrl Pts',(71.0815439811023,0.0339353377155988,
-20.9267567549895));
#24062=CARTESIAN_POINT('Ctrl Pts',(71.0419256931877,-3.43769557006433,-20.9323864361554));
#24063=CARTESIAN_POINT('Ctrl Pts',(71.0023074052732,-6.91075755094984,-20.0555225019279));
#24064=CARTESIAN_POINT('Ctrl Pts',(70.9626891173586,-9.96364670214212,-18.4026097141319));
#24065=CARTESIAN_POINT('Ctrl Pts',(70.923070829444,-13.0165358533344,-16.7496969263358));
#24066=CARTESIAN_POINT('Ctrl Pts',(70.8834525415295,-15.6492521748335,-14.3207352849711));
#24067=CARTESIAN_POINT('Ctrl Pts',(70.8438342536149,-17.5422034790138,-11.4105826752288));
#24068=CARTESIAN_POINT('Ctrl Pts',(70.8042159657003,-19.435154783194,-8.5004300654865));
#24069=CARTESIAN_POINT('Ctrl Pts',(70.7645976777857,-20.5883410700555,-5.10908648736654));
#24070=CARTESIAN_POINT('Ctrl Pts',(70.7249793898711,-20.861774098182,-1.64823583542732));
#24071=CARTESIAN_POINT('Ctrl Pts',(70.7187052089647,-20.9050765318448,-1.10015553657129));
#24072=CARTESIAN_POINT('Ctrl Pts',(70.7124310280583,-20.926315001003,-0.550332019836438));
#24073=CARTESIAN_POINT('Ctrl Pts',(70.7061568471518,-20.9257818388602,-0.000467423370275055));
#24074=CARTESIAN_POINT('Ctrl Pts',(70.4938431528481,-20.9261779264193,-0.000381460781396608));
#24075=CARTESIAN_POINT('Ctrl Pts',(70.4985030872841,-20.926522300612,-0.408752329164892));
#24076=CARTESIAN_POINT('Ctrl Pts',(70.5031630217201,-20.9148124849085,-0.81710346289888));
#24077=CARTESIAN_POINT('Ctrl Pts',(70.507822956156,-20.8909145891097,-1.22474006541663));
#24078=CARTESIAN_POINT('Ctrl Pts',(70.5474412440706,-20.6877371132634,-4.69042493823162));
#24079=CARTESIAN_POINT('Ctrl Pts',(70.5870595319852,-19.6035775169795,-8.10446187133154));
#24080=CARTESIAN_POINT('Ctrl Pts',(70.6266778198998,-17.7700447003034,-11.0524120658346));
#24081=CARTESIAN_POINT('Ctrl Pts',(70.6662961078144,-15.9365118836273,-14.0003622603376));
#24082=CARTESIAN_POINT('Ctrl Pts',(70.7059143957289,-13.3536058465589,-16.4822257162438));
#24083=CARTESIAN_POINT('Ctrl Pts',(70.7455326836435,-10.3348721858182,-18.1967227121314));
#24084=CARTESIAN_POINT('Ctrl Pts',(70.7851509715581,-7.31613852507755,-19.911219708019));
#24085=CARTESIAN_POINT('Ctrl Pts',(70.8247692594727,-3.8615772406645,-20.8583502438879));
#24086=CARTESIAN_POINT('Ctrl Pts',(70.8643875473873,-0.390546384666549,
-20.9231396890874));
#24087=CARTESIAN_POINT('Ctrl Pts',(70.9040058353019,3.0804844713314,-20.9879291342869));
#24088=CARTESIAN_POINT('Ctrl Pts',(70.9436241232164,6.56798489891426,-20.170377488817));
#24089=CARTESIAN_POINT('Ctrl Pts',(70.983242411131,9.64859827329515,-18.5697294569708));
#24090=CARTESIAN_POINT('Ctrl Pts',(71.0228606990455,12.7292116476761,-16.9690814251246));
#24091=CARTESIAN_POINT('Ctrl Pts',(71.0624789869601,15.402937968855,-14.5853370069021));
#24092=CARTESIAN_POINT('Ctrl Pts',(71.1020972748747,17.3452067411371,-11.7078650453502));
#24093=CARTESIAN_POINT('Ctrl Pts',(71.1417155627893,19.2874755134191,-8.83039308379838));
#24094=CARTESIAN_POINT('Ctrl Pts',(71.1813338507039,20.4982867368043,-5.45919357891726));
#24095=CARTESIAN_POINT('Ctrl Pts',(71.2209521386185,20.8306569304741,-2.00350508960085));
#24096=CARTESIAN_POINT('Ctrl Pts',(71.2605704265331,21.1630271241438,1.45218339971558));
#24097=CARTESIAN_POINT('Ctrl Pts',(71.3001887144476,20.6169562880982,4.99236087346727));
#24098=CARTESIAN_POINT('Ctrl Pts',(71.3398070023622,19.2587333621318,8.18727610869908));
#24099=CARTESIAN_POINT('Ctrl Pts',(71.3794252902768,17.9005104361654,11.3821913439309));
#24100=CARTESIAN_POINT('Ctrl Pts',(71.4190435781914,15.7301354202783,14.2318443406428));
#24101=CARTESIAN_POINT('Ctrl Pts',(71.458661866106,13.0110757048767,16.3903084108907));
#24102=CARTESIAN_POINT('Ctrl Pts',(71.4982801540205,10.2920159894752,18.5487724811387));
#24103=CARTESIAN_POINT('Ctrl Pts',(71.5378984419351,7.02427157455919,20.0160476249225));
#24104=CARTESIAN_POINT('Ctrl Pts',(71.5775167298497,3.60452233700019,20.6140175491853));
#24105=CARTESIAN_POINT('Ctrl Pts',(71.6171350177642,0.184773099441191,21.211987473448));
#24106=CARTESIAN_POINT('Ctrl Pts',(71.6567533056788,-3.38698096076084,20.9406521781897));
#24107=CARTESIAN_POINT('Ctrl Pts',(71.6963715935934,-6.67715545615774,19.8329497506961));
#24108=CARTESIAN_POINT('Ctrl Pts',(71.735989881508,-9.96732995155464,18.7252473232025));
#24109=CARTESIAN_POINT('Ctrl Pts',(71.7756081694226,-12.9759248821464,16.7811777634736));
#24110=CARTESIAN_POINT('Ctrl Pts',(71.8152264573371,-15.3377191917709,14.236736662324));
#24111=CARTESIAN_POINT('Ctrl Pts',(71.8548447452517,-17.6995135013954,11.6922955611743));
#24112=CARTESIAN_POINT('Ctrl Pts',(71.8944630331663,-19.4145071900526,8.54748291860389));
#24113=CARTESIAN_POINT('Ctrl Pts',(71.9340813210809,-20.2745127746554,5.18405560817734));
#24114=CARTESIAN_POINT('Ctrl Pts',(71.95400193167,-20.706935205232,3.49287890109326));
#24115=CARTESIAN_POINT('Ctrl Pts',(71.9739225422591,-20.9231983203047,1.74643172095956));
#24116=CARTESIAN_POINT('Ctrl Pts',(71.9938431528481,-20.923224691771,-9.04407733959185E-6));
#24117=CARTESIAN_POINT('Origin',(80.4,0.,0.));
#24118=CARTESIAN_POINT('',(73.7061568471518,-20.9264624460885,0.000284169623841063));
#24119=CARTESIAN_POINT('',(73.4938431528481,-20.9261267613403,0.000395174936093916));
#24120=CARTESIAN_POINT('',(80.4,-20.925,-2.56257342721584E-15));
#24121=CARTESIAN_POINT('Ctrl Pts',(73.7061568471518,-20.9264624460885,0.000284169623841063));
#24122=CARTESIAN_POINT('Ctrl Pts',(73.7028882259227,-20.9266544080345,0.286716760992491));
#24123=CARTESIAN_POINT('Ctrl Pts',(73.6996196046936,-20.9208949345101,0.573141625488209));
#24124=CARTESIAN_POINT('Ctrl Pts',(73.6963509834645,-20.9091336340165,0.859319827974444));
#24125=CARTESIAN_POINT('Ctrl Pts',(73.6567326955499,-20.76657732157,4.32802715938114));
#24126=CARTESIAN_POINT('Ctrl Pts',(73.6171144076354,-19.742270570929,7.76049646925485));
#24127=CARTESIAN_POINT('Ctrl Pts',(73.5774961197208,-17.9605566060624,10.7400515032444));
#24128=CARTESIAN_POINT('Ctrl Pts',(73.5378778318062,-16.1788426411958,13.7196065372339));
#24129=CARTESIAN_POINT('Ctrl Pts',(73.4982595438916,-13.6397214621036,16.2462472953392));
#24130=CARTESIAN_POINT('Ctrl Pts',(73.458641255977,-10.6514235019624,18.0132583747015));
#24131=CARTESIAN_POINT('Ctrl Pts',(73.4190229680625,-7.66312554182124,19.7802694540639));
#24132=CARTESIAN_POINT('Ctrl Pts',(73.3794046801479,-4.22565080063109,20.7876508546832));
#24133=CARTESIAN_POINT('Ctrl Pts',(73.3397863922333,-0.756283154890432,
20.913113964246));
#24134=CARTESIAN_POINT('Ctrl Pts',(73.3001681043188,2.71308449085023,21.0385770738088));
#24135=CARTESIAN_POINT('Ctrl Pts',(73.2605498164042,6.21434504114142,20.2821218923151));
#24136=CARTESIAN_POINT('Ctrl Pts',(73.2209315284896,9.32247149649723,18.7355764546733));
#24137=CARTESIAN_POINT('Ctrl Pts',(73.181313240575,12.430597951853,17.1890310170316));
#24138=CARTESIAN_POINT('Ctrl Pts',(73.1416949526605,15.1455903122734,14.8523953232418));
#24139=CARTESIAN_POINT('Ctrl Pts',(73.1020766647459,17.1378686907431,12.0093195740126));
#24140=CARTESIAN_POINT('Ctrl Pts',(73.0624583768313,19.1301470692127,9.16624382478331));
#24141=CARTESIAN_POINT('Ctrl Pts',(73.0228400889167,20.3997114657316,5.81672802011455));
#24142=CARTESIAN_POINT('Ctrl Pts',(72.9832218010021,20.7924462015731,2.36737847557188));
#24143=CARTESIAN_POINT('Ctrl Pts',(72.9436035130875,21.1851809374146,-1.08197106897078));
#24144=CARTESIAN_POINT('Ctrl Pts',(72.9039852251729,20.7010860125789,-4.63115435338729));
#24145=CARTESIAN_POINT('Ctrl Pts',(72.8643669372584,19.3989269517715,-7.84932691456705));
#24146=CARTESIAN_POINT('Ctrl Pts',(72.8247486493438,18.0967678909641,-11.0674994757468));
#24147=CARTESIAN_POINT('Ctrl Pts',(72.7851303614292,15.9765446941852,-13.9546613136897));
#24148=CARTESIAN_POINT('Ctrl Pts',(72.7455120735146,13.2956366939988,-16.1603324468621));
#24149=CARTESIAN_POINT('Ctrl Pts',(72.7058937856001,10.6147286938125,-18.3660035800345));
#24150=CARTESIAN_POINT('Ctrl Pts',(72.6662754976855,7.37313589021869,-19.8901840084363));
#24151=CARTESIAN_POINT('Ctrl Pts',(72.6266572097709,3.96436354884304,-20.5478495601004));
#24152=CARTESIAN_POINT('Ctrl Pts',(72.5870389218563,0.555591207467407,-21.2055151117644));
#24153=CARTESIAN_POINT('Ctrl Pts',(72.5474206339417,-3.02036067169011,-20.9966657866908));
#24154=CARTESIAN_POINT('Ctrl Pts',(72.5078023460271,-6.32939811713748,-19.9466543401817));
#24155=CARTESIAN_POINT('Ctrl Pts',(72.4681840581126,-9.63843556258485,-18.8966428936726));
#24156=CARTESIAN_POINT('Ctrl Pts',(72.428565770198,-12.6805585743221,-17.0054693257279));
#24157=CARTESIAN_POINT('Ctrl Pts',(72.3889474822835,-15.0864760364287,-14.5027080469193));
#24158=CARTESIAN_POINT('Ctrl Pts',(72.3493291943689,-17.4923934985352,-11.9999467681106));
#24159=CARTESIAN_POINT('Ctrl Pts',(72.3097109064543,-19.2621054110111,-8.88559777843788));
#24160=CARTESIAN_POINT('Ctrl Pts',(72.2700926185397,-20.1807819052104,-5.53771989055453));
#24161=CARTESIAN_POINT('Ctrl Pts',(72.2487806947437,-20.6749669007791,-3.73679102208467));
#24162=CARTESIAN_POINT('Ctrl Pts',(72.2274687709478,-20.9228875520371,-1.86828583450939));
#24163=CARTESIAN_POINT('Ctrl Pts',(72.2061568471519,-20.9232657042053,0.000120932580692235));
#24164=CARTESIAN_POINT('Ctrl Pts',(71.9938431528481,-20.923224691771,-9.04407733959185E-6));
#24165=CARTESIAN_POINT('Ctrl Pts',(72.0135408301736,-20.923250768112,-1.72690524055486));
#24166=CARTESIAN_POINT('Ctrl Pts',(72.0332385074991,-20.7118528671994,-3.45379516471595));
#24167=CARTESIAN_POINT('Ctrl Pts',(72.0529361848246,-20.2889561314617,-5.12723706239442));
#24168=CARTESIAN_POINT('Ctrl Pts',(72.0925544727392,-19.4383764231168,-8.49306044425692));
#24169=CARTESIAN_POINT('Ctrl Pts',(72.1321727606538,-17.7321995258788,-11.6426652296992));
#24170=CARTESIAN_POINT('Ctrl Pts',(72.1717910485684,-15.3775426299187,-14.193712814598));
#24171=CARTESIAN_POINT('Ctrl Pts',(72.211409336483,-13.0228857339585,-16.7447603994967));
#24172=CARTESIAN_POINT('Ctrl Pts',(72.2510276243975,-10.0197488392763,-18.6972507838519));
#24173=CARTESIAN_POINT('Ctrl Pts',(72.2906459123121,-6.73269043703646,-19.814166151453));
#24174=CARTESIAN_POINT('Ctrl Pts',(72.3302642002267,-3.4456320347966,-20.9310815190541));
#24175=CARTESIAN_POINT('Ctrl Pts',(72.3698824881413,0.125347875000815,-21.2124218699011));
#24176=CARTESIAN_POINT('Ctrl Pts',(72.4095007760559,3.54675888097773,-20.6240345771262));
#24177=CARTESIAN_POINT('Ctrl Pts',(72.4491190639704,6.96816988695464,-20.0356472843512));
#24178=CARTESIAN_POINT('Ctrl Pts',(72.488737351885,10.240011989111,-18.5775323479543));
#24179=CARTESIAN_POINT('Ctrl Pts',(72.5283556397996,12.965107881875,-16.4266940803577));
#24180=CARTESIAN_POINT('Ctrl Pts',(72.5679739277141,15.6902037746389,-14.2758558127611));
#24181=CARTESIAN_POINT('Ctrl Pts',(72.6075922156288,17.8685534580103,-11.4322942139648));
#24182=CARTESIAN_POINT('Ctrl Pts',(72.6472105035433,19.2357214761139,-8.24119652063211));
#24183=CARTESIAN_POINT('Ctrl Pts',(72.6868287914579,20.6028894942175,-5.05009882729935));
#24184=CARTESIAN_POINT('Ctrl Pts',(72.7264470793725,21.1588758470531,-1.51146503943013));
#24185=CARTESIAN_POINT('Ctrl Pts',(72.766065367287,20.8361879250575,1.94514101031227));
#24186=CARTESIAN_POINT('Ctrl Pts',(72.8056836552016,20.5135000030618,5.40174706005465));
#24187=CARTESIAN_POINT('Ctrl Pts',(72.8453019431162,19.3121378062348,8.77632537167022));
#24188=CARTESIAN_POINT('Ctrl Pts',(72.8849202310308,17.377937773333,11.6592272275857));
#24189=CARTESIAN_POINT('Ctrl Pts',(72.9245385189454,15.4437377404312,14.5421290835011));
#24190=CARTESIAN_POINT('Ctrl Pts',(72.9641568068599,12.7766998714546,16.9333544837164));
#24191=CARTESIAN_POINT('Ctrl Pts',(73.0037750947745,9.70058273469135,18.542626443029));
#24192=CARTESIAN_POINT('Ctrl Pts',(73.0433933826891,6.62446559792813,20.1518984023415));
#24193=CARTESIAN_POINT('Ctrl Pts',(73.0830116706037,3.13926919337822,20.9792169207512));
#24194=CARTESIAN_POINT('Ctrl Pts',(73.1226299585183,-0.331929547330916,
20.9241516811057));
#24195=CARTESIAN_POINT('Ctrl Pts',(73.1622482464329,-3.80312828804008,20.8690864414602));
#24196=CARTESIAN_POINT('Ctrl Pts',(73.2018665343474,-7.26032936490853,19.9316374437595));
#24197=CARTESIAN_POINT('Ctrl Pts',(73.241484822262,-10.2838542709487,18.2256040265391));
#24198=CARTESIAN_POINT('Ctrl Pts',(73.2811031101765,-13.307379176989,16.5195706093187));
#24199=CARTESIAN_POINT('Ctrl Pts',(73.3207213980912,-15.8972279122009,14.0449527725788));
#24200=CARTESIAN_POINT('Ctrl Pts',(73.3603396860057,-17.7390120952464,11.1021507233064));
#24201=CARTESIAN_POINT('Ctrl Pts',(73.3999579739203,-19.5807962782918,8.15934867403405));
#24202=CARTESIAN_POINT('Ctrl Pts',(73.4395762618349,-20.6745159091708,4.7483624122293));
#24203=CARTESIAN_POINT('Ctrl Pts',(73.4791945497495,-20.8874015563273,1.28326030993092));
#24204=CARTESIAN_POINT('Ctrl Pts',(73.484077417449,-20.913639248689,0.856194022577959));
#24205=CARTESIAN_POINT('Ctrl Pts',(73.4889602851486,-20.9264970502493,0.428305714220112));
#24206=CARTESIAN_POINT('Ctrl Pts',(73.4938431528481,-20.9261267613403,0.000395174936093916));
#24207=CARTESIAN_POINT('Origin',(80.4,0.,0.));
#24208=CARTESIAN_POINT('',(75.2061568471518,-20.9243088587828,-0.000506040078050995));
#24209=CARTESIAN_POINT('',(74.9938431528481,-20.9247245309142,-0.000535895639339255));
#24210=CARTESIAN_POINT('',(80.4,-20.925,-2.56257342721584E-15));
#24211=CARTESIAN_POINT('Ctrl Pts',(75.2061568471518,-20.9243088587828,-0.000506040078050995));
#24212=CARTESIAN_POINT('Ctrl Pts',(75.1783076808977,-20.9220942780769,2.44066904141215));
#24213=CARTESIAN_POINT('Ctrl Pts',(75.1504585146435,-20.4950188134656,4.88259874686084));
#24214=CARTESIAN_POINT('Ctrl Pts',(75.1226093483894,-19.6583159988833,7.17501999857562));
#24215=CARTESIAN_POINT('Ctrl Pts',(75.0829910604748,-18.4680206519944,10.436223739581));
#24216=CARTESIAN_POINT('Ctrl Pts',(75.0433727725602,-16.4487225807659,13.3948526757888));
#24217=CARTESIAN_POINT('Ctrl Pts',(75.0037544846456,-13.8455495578827,15.6917512512826));
#24218=CARTESIAN_POINT('Ctrl Pts',(74.9641361967311,-11.2423765349993,17.9886498267764));
#24219=CARTESIAN_POINT('Ctrl Pts',(74.9245179088165,-8.05532856046113,19.6238180415562));
#24220=CARTESIAN_POINT('Ctrl Pts',(74.8848996209019,-4.67128956317847,20.3987586315651));
#24221=CARTESIAN_POINT('Ctrl Pts',(74.8452813329873,-1.2872505658958,21.1736992215741));
#24222=CARTESIAN_POINT('Ctrl Pts',(74.8056630450727,2.29377945413133,21.0884121868122));
#24223=CARTESIAN_POINT('Ctrl Pts',(74.7660447571582,5.63709007686453,20.153250739204));
#24224=CARTESIAN_POINT('Ctrl Pts',(74.7264264692436,8.98040069959767,19.2180892915959));
#24225=CARTESIAN_POINT('Ctrl Pts',(74.686808181329,12.0859919250369,17.4330534311413));
#24226=CARTESIAN_POINT('Ctrl Pts',(74.6471898934144,14.5768680679944,15.0148332398398));
#24227=CARTESIAN_POINT('Ctrl Pts',(74.6075716054999,17.0677442109518,12.5966130485383));
#24228=CARTESIAN_POINT('Ctrl Pts',(74.5679533175852,18.9439052714275,9.54520852638985));
#24229=CARTESIAN_POINT('Ctrl Pts',(74.5283350296707,19.9775992456411,6.23103749567228));
#24230=CARTESIAN_POINT('Ctrl Pts',(74.4887167417561,21.0112932198546,2.91686646495466));
#24231=CARTESIAN_POINT('Ctrl Pts',(74.4490984538415,21.2025201078059,-0.660071074332059));
#24232=CARTESIAN_POINT('Ctrl Pts',(74.409480165927,20.5280663870395,-4.06556149888438));
#24233=CARTESIAN_POINT('Ctrl Pts',(74.3698618780124,19.8536126662731,-7.47105192343671));
#24234=CARTESIAN_POINT('Ctrl Pts',(74.3302435900978,18.3134783367888,-10.7050952332546));
#24235=CARTESIAN_POINT('Ctrl Pts',(74.2906253021832,16.0946242555306,-13.3751026151278));
#24236=CARTESIAN_POINT('Ctrl Pts',(74.2510070142686,13.8757701742724,-16.0451099970009));
#24237=CARTESIAN_POINT('Ctrl Pts',(74.211388726354,10.9781963412402,-18.1510814509292));
#24238=CARTESIAN_POINT('Ctrl Pts',(74.1717704384395,7.75364667676002,-19.4373676999711));
#24239=CARTESIAN_POINT('Ctrl Pts',(74.1321521505249,4.52909701227992,-20.723653949013));
#24240=CARTESIAN_POINT('Ctrl Pts',(74.0925338626103,0.977571516351926,-21.1902549931685));
#24241=CARTESIAN_POINT('Ctrl Pts',(74.0529155746958,-2.46980102084973,-20.7805289347822));
#24242=CARTESIAN_POINT('Ctrl Pts',(74.0132972867812,-5.91717355805138,-20.370802876396));
#24243=CARTESIAN_POINT('Ctrl Pts',(73.9736789988666,-9.2603931365267,-19.084749715468));
#24244=CARTESIAN_POINT('Ctrl Pts',(73.934060710952,-12.0936177557586,-17.0784867441326));
#24245=CARTESIAN_POINT('Ctrl Pts',(73.8944424230374,-14.9268423749905,-15.0722237727972));
#24246=CARTESIAN_POINT('Ctrl Pts',(73.8548241351229,-17.2500720349789,-12.3457509910545));
#24247=CARTESIAN_POINT('Ctrl Pts',(73.8152058472083,-18.7812839278471,-9.23004192371327));
#24248=CARTESIAN_POINT('Ctrl Pts',(73.7788561805228,-20.1861664924497,-6.37138769991231));
#24249=CARTESIAN_POINT('Ctrl Pts',(73.7425065138373,-20.9243276766347,-3.18507396591327));
#24250=CARTESIAN_POINT('Ctrl Pts',(73.7061568471518,-20.9264624460885,0.000284169623841063));
#24251=CARTESIAN_POINT('Ctrl Pts',(73.4938431528481,-20.9261267613403,0.000395174936093916));
#24252=CARTESIAN_POINT('Ctrl Pts',(73.5285785730632,-20.9234926246723,-3.04364642337207));
#24253=CARTESIAN_POINT('Ctrl Pts',(73.5633139932782,-20.2514482408018,-6.08881302228566));
#24254=CARTESIAN_POINT('Ctrl Pts',(73.5980494134932,-18.9646405085985,-8.84718662502006));
#24255=CARTESIAN_POINT('Ctrl Pts',(73.6376677014078,-17.4969421502789,-11.9933135148807));
#24256=CARTESIAN_POINT('Ctrl Pts',(73.6772859893224,-15.2294937702056,-14.7663493518099));
#24257=CARTESIAN_POINT('Ctrl Pts',(73.7169042772369,-12.4375467435986,-16.8296682022881));
#24258=CARTESIAN_POINT('Ctrl Pts',(73.7565225651515,-9.64559971699171,-18.8929870527663));
#24259=CARTESIAN_POINT('Ctrl Pts',(73.7961408530661,-6.32915404385119,-20.2465889167936));
#24260=CARTESIAN_POINT('Ctrl Pts',(73.8357591409807,-2.89080157164628,-20.7261565918932));
#24261=CARTESIAN_POINT('Ctrl Pts',(73.8753774288953,0.547550900558613,-21.2057242669927));
#24262=CARTESIAN_POINT('Ctrl Pts',(73.9149957168098,4.10781017182792,-20.8112577531646));
#24263=CARTESIAN_POINT('Ctrl Pts',(73.9546140047244,7.35778723659513,-19.5906423523913));
#24264=CARTESIAN_POINT('Ctrl Pts',(73.994232292639,10.6077643013624,-18.3700269516179));
#24265=CARTESIAN_POINT('Ctrl Pts',(74.0338505805536,13.5474591596276,-16.3232626638993));
#24266=CARTESIAN_POINT('Ctrl Pts',(74.0734688684682,15.8200147117645,-13.6988114563952));
#24267=CARTESIAN_POINT('Ctrl Pts',(74.1130871563828,18.0925702639014,-11.0743602488911));
#24268=CARTESIAN_POINT('Ctrl Pts',(74.1527054442973,19.6979865099099,-7.87222212160154));
#24269=CARTESIAN_POINT('Ctrl Pts',(74.1923237322119,20.4413778535412,-4.48111283578782));
#24270=CARTESIAN_POINT('Ctrl Pts',(74.2319420201265,21.1847691971725,-1.09000354997409));
#24271=CARTESIAN_POINT('Ctrl Pts',(74.2715603080411,21.0661356384265,2.49007689436369));
#24272=CARTESIAN_POINT('Ctrl Pts',(74.3111785959557,20.0998784093131,5.82453334861588));
#24273=CARTESIAN_POINT('Ctrl Pts',(74.3507968838702,19.1336211801997,9.15898980286805));
#24274=CARTESIAN_POINT('Ctrl Pts',(74.3904151717848,17.3197402807189,12.2478222670347));
#24275=CARTESIAN_POINT('Ctrl Pts',(74.4300334596993,14.8784273661496,14.7160694449476));
#24276=CARTESIAN_POINT('Ctrl Pts',(74.4696517476139,12.4371144515803,17.1843166228605));
#24277=CARTESIAN_POINT('Ctrl Pts',(74.5092700355286,9.36836952192247,19.0319785145197));
#24278=CARTESIAN_POINT('Ctrl Pts',(74.5488883234432,6.04471539600249,20.0347627033524));
#24279=CARTESIAN_POINT('Ctrl Pts',(74.5885066113577,2.72106127008243,21.037546892185));
#24280=CARTESIAN_POINT('Ctrl Pts',(74.6281248992722,-0.857502052099787,
21.1954533781911));
#24281=CARTESIAN_POINT('Ctrl Pts',(74.6677431871868,-4.25656358928468,20.4893134879792));
#24282=CARTESIAN_POINT('Ctrl Pts',(74.7073614751014,-7.65562512646958,19.7831735977672));
#24283=CARTESIAN_POINT('Ctrl Pts',(74.746979763016,-10.8751848786571,18.2129873313374));
#24284=CARTESIAN_POINT('Ctrl Pts',(74.7865980509306,-13.5244122288502,15.9693636273471));
#24285=CARTESIAN_POINT('Ctrl Pts',(74.8262163388453,-16.1736395790433,13.7257399233568));
#24286=CARTESIAN_POINT('Ctrl Pts',(74.8658346267597,-18.252534527242,10.8086787818062));
#24287=CARTESIAN_POINT('Ctrl Pts',(74.9054529146743,-19.5087346829906,7.57228973739029));
#24288=CARTESIAN_POINT('Ctrl Pts',(74.9349163273989,-20.4429482899325,5.1654450408548));
#24289=CARTESIAN_POINT('Ctrl Pts',(74.9643797401235,-20.9221597565615,2.58199186132092));
#24290=CARTESIAN_POINT('Ctrl Pts',(74.9938431528481,-20.9247245309142,-0.000535895639339255));
#24291=CARTESIAN_POINT('Origin',(80.4,0.,0.));
#24292=CARTESIAN_POINT('',(76.7061568471518,-20.9240642695764,0.000470086318913876));
#24293=CARTESIAN_POINT('',(76.4938431528481,-20.9237353903355,0.000391611568432831));
#24294=CARTESIAN_POINT('',(80.4,-20.925,-2.56257342721584E-15));
#24295=CARTESIAN_POINT('Ctrl Pts',(76.7061568471518,-20.9240642695764,0.000470086318913876));
#24296=CARTESIAN_POINT('Ctrl Pts',(76.6933454237872,-20.9249940480266,1.1235190201765));
#24297=CARTESIAN_POINT('Ctrl Pts',(76.6805340004226,-20.8361268006114,2.24642227573881));
#24298=CARTESIAN_POINT('Ctrl Pts',(76.667722577058,-20.6561712045076,3.35453291263967));
#24299=CARTESIAN_POINT('Ctrl Pts',(76.6281042891434,-20.0996731156252,6.78127520383157));
#24300=CARTESIAN_POINT('Ctrl Pts',(76.5884860012288,-18.6720921626798,10.0665548731172));
#24301=CARTESIAN_POINT('Ctrl Pts',(76.5488677133143,-16.54672605952,12.8115633941809));
#24302=CARTESIAN_POINT('Ctrl Pts',(76.5092494253997,-14.4213599563602,15.5565719152446));
#24303=CARTESIAN_POINT('Ctrl Pts',(76.469631137485,-11.598208702986,17.7613092880865));
#24304=CARTESIAN_POINT('Ctrl Pts',(76.4300128495705,-8.41998187187309,19.1581367875178));
#24305=CARTESIAN_POINT('Ctrl Pts',(76.3903945616559,-5.24175504076021,20.554964286949));
#24306=CARTESIAN_POINT('Ctrl Pts',(76.3507762737414,-1.70845263190867,21.1438819129698));
#24307=CARTESIAN_POINT('Ctrl Pts',(76.3111579858268,1.7510087117926,20.8533994442906));
#24308=CARTESIAN_POINT('Ctrl Pts',(76.2715396979122,5.21047005549381,20.5629169756114));
#24309=CARTESIAN_POINT('Ctrl Pts',(76.2319214099976,8.59609033404474,19.3930344122323));
#24310=CARTESIAN_POINT('Ctrl Pts',(76.192303122083,11.4968804171816,17.4857667994554));
#24311=CARTESIAN_POINT('Ctrl Pts',(76.1526848341684,14.3976705003185,15.5784991866785));
#24312=CARTESIAN_POINT('Ctrl Pts',(76.1130665462539,16.8136303880413,12.9338465245038));
#24313=CARTESIAN_POINT('Ctrl Pts',(76.0734482583393,18.4514805122609,9.87284998354419));
#24314=CARTESIAN_POINT('Ctrl Pts',(76.0338299704247,20.0893306364805,6.81185344258452));
#24315=CARTESIAN_POINT('Ctrl Pts',(75.9942116825101,20.9490709971969,3.33451302283995));
#24316=CARTESIAN_POINT('Ctrl Pts',(75.9545933945955,20.9263355066529,-0.137048002209587));
#24317=CARTESIAN_POINT('Ctrl Pts',(75.9149751066809,20.9036000161089,-3.60860902725913));
#24318=CARTESIAN_POINT('Ctrl Pts',(75.8753568187664,19.9983886743046,-7.07439065761364));
#24319=CARTESIAN_POINT('Ctrl Pts',(75.8357385308518,18.3205874080315,-10.1136727708874));
#24320=CARTESIAN_POINT('Ctrl Pts',(75.7961202429372,16.6427861417585,-13.1529548841611));
#24321=CARTESIAN_POINT('Ctrl Pts',(75.7565019550227,14.1923949510166,-15.7657374803541));
#24322=CARTESIAN_POINT('Ctrl Pts',(75.7168836671081,11.2668731080905,-17.6348481779147));
#24323=CARTESIAN_POINT('Ctrl Pts',(75.6772653791935,8.34135126516437,-19.5039588754752));
#24324=CARTESIAN_POINT('Ctrl Pts',(75.6376470912789,4.94069877005392,-20.6293976744032));
#24325=CARTESIAN_POINT('Ctrl Pts',(75.5980288033643,1.47772955235106,-20.8745446719688));
#24326=CARTESIAN_POINT('Ctrl Pts',(75.5584105154498,-1.98523966535179,-21.1196916695344));
#24327=CARTESIAN_POINT('Ctrl Pts',(75.5187922275352,-5.51052560564705,-20.4845468657374));
#24328=CARTESIAN_POINT('Ctrl Pts',(75.4791739396206,-8.67018476532732,-19.0462121175576));
#24329=CARTESIAN_POINT('Ctrl Pts',(75.439555651706,-11.8298439250076,-17.6078773693778));
#24330=CARTESIAN_POINT('Ctrl Pts',(75.3999373637915,-14.6238763040729,-15.366352676815));
#24331=CARTESIAN_POINT('Ctrl Pts',(75.3603190758769,-16.7131071448944,-12.5937424721642));
#24332=CARTESIAN_POINT('Ctrl Pts',(75.3207007879623,-18.8023379857158,-9.82113226751339));
#24333=CARTESIAN_POINT('Ctrl Pts',(75.2810825000477,-20.1867672882934,-6.51743655077455));
#24334=CARTESIAN_POINT('Ctrl Pts',(75.2414642121331,-20.6983356283075,-3.08369941950365));
#24335=CARTESIAN_POINT('Ctrl Pts',(75.2296950904727,-20.8503035791748,-2.06366366896917));
#24336=CARTESIAN_POINT('Ctrl Pts',(75.2179259688123,-20.9252447456786,-1.03215223968963));
#24337=CARTESIAN_POINT('Ctrl Pts',(75.2061568471518,-20.9243088587828,-0.000506040078050995));
#24338=CARTESIAN_POINT('Ctrl Pts',(74.9938431528481,-20.9247245309142,-0.000535895639339255));
#24339=CARTESIAN_POINT('Ctrl Pts',(75.0039980280381,-20.9256085073797,-0.890631258715375));
#24340=CARTESIAN_POINT('Ctrl Pts',(75.0141529032281,-20.8698712062196,-1.78061669003418));
#24341=CARTESIAN_POINT('Ctrl Pts',(75.024307778418,-20.7566264448263,-2.66322350324698));
#24342=CARTESIAN_POINT('Ctrl Pts',(75.0639260663326,-20.3148126876145,-6.10663075218757));
#24343=CARTESIAN_POINT('Ctrl Pts',(75.1035443542472,-18.9976798098923,-9.43772830278766));
#24344=CARTESIAN_POINT('Ctrl Pts',(75.1431626421618,-16.9651179503399,-12.2521456785888));
#24345=CARTESIAN_POINT('Ctrl Pts',(75.1827809300764,-14.9325560907876,-15.0665630543899));
#24346=CARTESIAN_POINT('Ctrl Pts',(75.222399217991,-12.1845652494053,-17.3643002553922));
#24347=CARTESIAN_POINT('Ctrl Pts',(75.2620175059056,-9.05473108345861,-18.8664290687071));
#24348=CARTESIAN_POINT('Ctrl Pts',(75.3016357938201,-5.92489691751194,-20.3685578820221));
#24349=CARTESIAN_POINT('Ctrl Pts',(75.3412540817347,-2.41321942700093,-21.0750783076498));
#24350=CARTESIAN_POINT('Ctrl Pts',(75.3808723696492,1.05400984949412,-20.9002240187869));
#24351=CARTESIAN_POINT('Ctrl Pts',(75.4204906575638,4.52123912598912,-20.7253697299241));
#24352=CARTESIAN_POINT('Ctrl Pts',(75.4601089454784,7.94402018846819,-19.6691407265706));
#24353=CARTESIAN_POINT('Ctrl Pts',(75.499727233393,10.9068528637832,-17.8597553568377));
#24354=CARTESIAN_POINT('Ctrl Pts',(75.5393455213076,13.8696855390983,-16.0503699871048));
#24355=CARTESIAN_POINT('Ctrl Pts',(75.5789638092222,16.3725698272493,-13.4878282509926));
#24356=CARTESIAN_POINT('Ctrl Pts',(75.6185820971367,18.1116741842043,-10.4832036631717));
#24357=CARTESIAN_POINT('Ctrl Pts',(75.6582003850513,19.8507785411594,-7.47857907535073));
#24358=CARTESIAN_POINT('Ctrl Pts',(75.6978186729659,20.8261029669184,-4.03187163582119));
#24359=CARTESIAN_POINT('Ctrl Pts',(75.7374369608805,20.9192503275774,-0.561486002016126));
#24360=CARTESIAN_POINT('Ctrl Pts',(75.7770552487951,21.0123976882365,2.90889963178892));
#24361=CARTESIAN_POINT('Ctrl Pts',(75.8166735367096,20.2233679837955,6.40296345986942));
#24362=CARTESIAN_POINT('Ctrl Pts',(75.8562918246242,18.6479435540623,9.49655211130938));
#24363=CARTESIAN_POINT('Ctrl Pts',(75.8959101125388,17.0725191243292,12.5901407627493));
#24364=CARTESIAN_POINT('Ctrl Pts',(75.9355284004534,14.7106999693039,15.2832542375487));
#24365=CARTESIAN_POINT('Ctrl Pts',(75.9751466883679,11.8491933746539,17.2489685827404));
#24366=CARTESIAN_POINT('Ctrl Pts',(76.0147649762825,8.98768678000398,19.2146829279322));
#24367=CARTESIAN_POINT('Ctrl Pts',(76.0543832641971,5.62649274572937,20.4529981435163));
#24368=CARTESIAN_POINT('Ctrl Pts',(76.0940015521117,2.173635237644,20.8135919689991));
#24369=CARTESIAN_POINT('Ctrl Pts',(76.1336198400263,-1.27922227044142,21.1741857944818));
#24370=CARTESIAN_POINT('Ctrl Pts',(76.1732381279408,-4.82374325233762,20.6570582298631));
#24371=CARTESIAN_POINT('Ctrl Pts',(76.2128564158554,-8.02964921379633,19.3249847167259));
#24372=CARTESIAN_POINT('Ctrl Pts',(76.25247470377,-11.235555175255,17.9929112035887));
#24373=CARTESIAN_POINT('Ctrl Pts',(76.2920929916846,-14.1028461162763,15.845891741933));
#24374=CARTESIAN_POINT('Ctrl Pts',(76.3317112795992,-16.2834542344755,13.144558531653));
#24375=CARTESIAN_POINT('Ctrl Pts',(76.3713295675138,-18.4640623526748,10.443225321373));
#24376=CARTESIAN_POINT('Ctrl Pts',(76.4109478554283,-19.9579876480521,7.18757836246868));
#24377=CARTESIAN_POINT('Ctrl Pts',(76.4505661433429,-20.5838786968473,3.77282899052993));
#24378=CARTESIAN_POINT('Ctrl Pts',(76.464991813178,-20.8117759154783,2.52946261600763));
#24379=CARTESIAN_POINT('Ctrl Pts',(76.4794174830131,-20.9245884769033,1.2650023195153));
#24380=CARTESIAN_POINT('Ctrl Pts',(76.4938431528481,-20.9237353903355,0.000391611568432831));
#24381=CARTESIAN_POINT('Origin',(80.4,0.,0.));
#24382=CARTESIAN_POINT('',(78.2061568471519,-20.9266265721997,-0.000199885376053199));
#24383=CARTESIAN_POINT('',(77.9938431528481,-20.9267713605918,-5.6450652404226E-5));
#24384=CARTESIAN_POINT('',(80.4,-20.925,-2.56257342721584E-15));
#24385=CARTESIAN_POINT('Ctrl Pts',(78.2061568471519,-20.9266265721997,-0.000199885376053199));
#24386=CARTESIAN_POINT('Ctrl Pts',(78.1687648787622,-20.9249937207778,3.27642156312699));
#24387=CARTESIAN_POINT('Ctrl Pts',(78.1313729103724,-20.1423394509286,6.55379572127686));
#24388=CARTESIAN_POINT('Ctrl Pts',(78.0939809419828,-18.6587817608754,9.47523947412083));
#24389=CARTESIAN_POINT('Ctrl Pts',(78.0543626540682,-17.0868929774374,12.5706261229379));
#24390=CARTESIAN_POINT('Ctrl Pts',(78.0147443661537,-14.7281524151643,15.2664363615343));
#24391=CARTESIAN_POINT('Ctrl Pts',(77.9751260782391,-11.8688936414524,17.2354188698681));
#24392=CARTESIAN_POINT('Ctrl Pts',(77.9355077903245,-9.00963486774041,19.2044013782019));
#24393=CARTESIAN_POINT('Ctrl Pts',(77.8958895024099,-5.64985788258961,20.446556156273));
#24394=CARTESIAN_POINT('Ctrl Pts',(77.8562712144953,-2.19741463258577,20.8110948492483));
#24395=CARTESIAN_POINT('Ctrl Pts',(77.8166529265807,1.25502861741808,21.1756335422237));
#24396=CARTESIAN_POINT('Ctrl Pts',(77.7770346386661,4.80013813227497,20.6625561501032));
#24397=CARTESIAN_POINT('Ctrl Pts',(77.7374163507516,8.00756397421087,19.3341464536408));
#24398=CARTESIAN_POINT('Ctrl Pts',(77.697798062837,11.2149898161467,18.0057367571785));
#24399=CARTESIAN_POINT('Ctrl Pts',(77.6581797749224,14.0847319851616,15.8619947563745));
#24400=CARTESIAN_POINT('Ctrl Pts',(77.6185614870079,16.2684251180171,13.1631547917429));
#24401=CARTESIAN_POINT('Ctrl Pts',(77.5789431990933,18.4521182508726,10.4643148271113));
#24402=CARTESIAN_POINT('Ctrl Pts',(77.5393249111787,19.9497623475687,7.21037689865213));
#24403=CARTESIAN_POINT('Ctrl Pts',(77.4997066232641,20.5795545495139,3.79634487836558));
#24404=CARTESIAN_POINT('Ctrl Pts',(77.4600883353496,21.2093467514592,0.382312858078985));
#24405=CARTESIAN_POINT('Ctrl Pts',(77.420470047435,20.9712870586536,-3.19181325403503));
#24406=CARTESIAN_POINT('Ctrl Pts',(77.3808517595204,19.8942741478675,-6.49216112102925));
#24407=CARTESIAN_POINT('Ctrl Pts',(77.3412334716058,18.8172612370814,-9.79250898802348));
#24408=CARTESIAN_POINT('Ctrl Pts',(77.3016151836912,16.9012951083147,-12.8190786098979));
#24409=CARTESIAN_POINT('Ctrl Pts',(77.2619968957766,14.3789598046942,-15.2044669366243));
#24410=CARTESIAN_POINT('Ctrl Pts',(77.2223786078621,11.8566245010736,-17.5898552633507));
#24411=CARTESIAN_POINT('Ctrl Pts',(77.1827603199475,8.72792002259909,-19.3340622949291));
#24412=CARTESIAN_POINT('Ctrl Pts',(77.1431420320329,5.37264783153356,-20.2253542656298));
#24413=CARTESIAN_POINT('Ctrl Pts',(77.1035237441183,2.01737564046811,-21.1166462363305));
#24414=CARTESIAN_POINT('Ctrl Pts',(77.0639054562038,-1.56446426318834,-21.1550231461535));
#24415=CARTESIAN_POINT('Ctrl Pts',(77.0242871682892,-4.93806314554617,-20.3358263235727));
#24416=CARTESIAN_POINT('Ctrl Pts',(76.9846688803746,-8.31166202790415,-19.5166295009918));
#24417=CARTESIAN_POINT('Ctrl Pts',(76.94505059246,-11.4770198889634,-17.839858946007));
#24418=CARTESIAN_POINT('Ctrl Pts',(76.9054323045454,-14.0498858183275,-15.509062137469));
#24419=CARTESIAN_POINT('Ctrl Pts',(76.8658140166308,-16.6227517476915,-13.178265328931));
#24420=CARTESIAN_POINT('Ctrl Pts',(76.8261957287163,-18.6031257453604,-10.1934422668398));
#24421=CARTESIAN_POINT('Ctrl Pts',(76.7865774408017,-19.750605131785,-6.91692827924511));
#24422=CARTESIAN_POINT('Ctrl Pts',(76.7597705762517,-20.5270224406819,-4.69994538359761));
#24423=CARTESIAN_POINT('Ctrl Pts',(76.7329637117018,-20.9221187835623,-2.34941874305164));
#24424=CARTESIAN_POINT('Ctrl Pts',(76.7061568471518,-20.9240642695764,0.000470086318913876));
#24425=CARTESIAN_POINT('Ctrl Pts',(76.4938431528481,-20.9237353903355,0.000391611568432831));
#24426=CARTESIAN_POINT('Ctrl Pts',(76.5190357709276,-20.9222455819358,-2.20809194231692));
#24427=CARTESIAN_POINT('Ctrl Pts',(76.5442283890071,-20.5740956707248,-4.41703422450956));
#24428=CARTESIAN_POINT('Ctrl Pts',(76.5694210070866,-19.886843487402,-6.51488732871773));
#24429=CARTESIAN_POINT('Ctrl Pts',(76.6090392950012,-18.8060604269481,-9.81400249105353));
#24430=CARTESIAN_POINT('Ctrl Pts',(76.6486575829158,-16.886637503827,-12.8383810307519));
#24431=CARTESIAN_POINT('Ctrl Pts',(76.6882758708304,-14.3615783902992,-15.2208858788705));
#24432=CARTESIAN_POINT('Ctrl Pts',(76.7278941587449,-11.8365192767715,-17.603390726989));
#24433=CARTESIAN_POINT('Ctrl Pts',(76.7675124466595,-8.70582397283707,-19.3440218835278));
#24434=CARTESIAN_POINT('Ctrl Pts',(76.8071307345741,-5.34953561216826,-20.2314796674008));
#24435=CARTESIAN_POINT('Ctrl Pts',(76.8467490224887,-1.99324725149935,-21.1189374512739));
#24436=CARTESIAN_POINT('Ctrl Pts',(76.8863673104033,1.58863416590386,-21.1532218624812));
#24437=CARTESIAN_POINT('Ctrl Pts',(76.9259855983179,4.96129486669173,-20.3301710284013));
#24438=CARTESIAN_POINT('Ctrl Pts',(76.9656038862325,8.33395556747946,-19.5071201943215));
#24439=CARTESIAN_POINT('Ctrl Pts',(77.005222174147,11.4973955516517,-17.8267341149546));
#24440=CARTESIAN_POINT('Ctrl Pts',(77.0448404620616,14.067596724807,-15.4929991669305));
#24441=CARTESIAN_POINT('Ctrl Pts',(77.0844587499761,16.6377978979623,-13.1592642189064));
#24442=CARTESIAN_POINT('Ctrl Pts',(77.1240770378908,18.6147602601005,-10.172180402225));
#24443=CARTESIAN_POINT('Ctrl Pts',(77.1636953258054,19.7584952788611,-6.89435748373493));
#24444=CARTESIAN_POINT('Ctrl Pts',(77.2033136137199,20.9022302976217,-3.61653456524486));
#24445=CARTESIAN_POINT('Ctrl Pts',(77.2429319016344,21.2127379730048,-0.0479725449460383));
#24446=CARTESIAN_POINT('Ctrl Pts',(77.282550189549,20.6523249817942,3.37813167959247));
#24447=CARTESIAN_POINT('Ctrl Pts',(77.3221684774636,20.0919119905837,6.80423590413097));
#24448=CARTESIAN_POINT('Ctrl Pts',(77.3617867653783,18.6605783327797,10.0878823329092));
#24449=CARTESIAN_POINT('Ctrl Pts',(77.4014050532928,16.5320772726997,12.8304607028663));
#24450=CARTESIAN_POINT('Ctrl Pts',(77.4410233412074,14.4035762126197,15.5730390728233));
#24451=CARTESIAN_POINT('Ctrl Pts',(77.4806416291219,11.5779077502638,17.7745493839593));
#24452=CARTESIAN_POINT('Ctrl Pts',(77.5202599170365,8.39808702856311,19.1677446523838));
#24453=CARTESIAN_POINT('Ctrl Pts',(77.5598782049511,5.21826630686235,20.5609399208084));
#24454=CARTESIAN_POINT('Ctrl Pts',(77.5994964928657,1.68429332581686,21.1458201465215));
#24455=CARTESIAN_POINT('Ctrl Pts',(77.6391147807803,-1.77483386920591,20.8513852186139));
#24456=CARTESIAN_POINT('Ctrl Pts',(77.6787330686949,-5.23396106422867,20.5569502907062));
#24457=CARTESIAN_POINT('Ctrl Pts',(77.7183513566094,-8.61824247322863,19.3832002091777));
#24458=CARTESIAN_POINT('Ctrl Pts',(77.7579696445239,-11.5168514947511,17.4726195072793));
#24459=CARTESIAN_POINT('Ctrl Pts',(77.7975879324385,-14.4154605162737,15.5620388053809));
#24460=CARTESIAN_POINT('Ctrl Pts',(77.8372062203532,-16.8283971503188,12.9146274831127));
#24461=CARTESIAN_POINT('Ctrl Pts',(77.8768245082678,-18.4627488293163,9.85176159191279));
#24462=CARTESIAN_POINT('Ctrl Pts',(77.9158307231279,-20.0718509915664,6.83621469858147));
#24463=CARTESIAN_POINT('Ctrl Pts',(77.954836937988,-20.9262394823794,3.41795100344054));
#24464=CARTESIAN_POINT('Ctrl Pts',(77.9938431528481,-20.9267713605918,-5.6450652404226E-5));
#24465=CARTESIAN_POINT('Origin',(80.4,0.,0.));
#24466=CARTESIAN_POINT('',(79.7061568471518,-20.923342133494,-0.000201647965826224));
#24467=CARTESIAN_POINT('',(79.4938431528481,-20.9235342978811,-0.000316448518974899));
#24468=CARTESIAN_POINT('',(80.4,-20.925,-2.56257342721584E-15));
#24469=CARTESIAN_POINT('Ctrl Pts',(79.7061568471518,-20.923342133494,-0.000201647965826224));
#24470=CARTESIAN_POINT('Ctrl Pts',(79.6838026216517,-20.9226777745741,1.95956275646496));
#24471=CARTESIAN_POINT('Ctrl Pts',(79.6614483961515,-20.6495711928031,3.91950855148925));
#24472=CARTESIAN_POINT('Ctrl Pts',(79.6390941706513,-20.1065201583901,5.80156418667976));
#24473=CARTESIAN_POINT('Ctrl Pts',(79.5994758827368,-19.1440733836838,9.13712246964086));
#24474=CARTESIAN_POINT('Ctrl Pts',(79.5598575948222,-17.333722852153,12.2280253855573));
#24475=CARTESIAN_POINT('Ctrl Pts',(79.5202393069077,-14.8952316586553,14.6990603008119));
#24476=CARTESIAN_POINT('Ctrl Pts',(79.4806210189931,-12.4567404651576,17.1700952160665));
#24477=CARTESIAN_POINT('Ctrl Pts',(79.4410027310785,-9.39010860969301,19.0212621306593));
#24478=CARTESIAN_POINT('Ctrl Pts',(79.4013844431639,-6.06760239959109,20.0278431442926));
#24479=CARTESIAN_POINT('Ctrl Pts',(79.3617661552493,-2.74509618948911,21.0344241579259));
#24480=CARTESIAN_POINT('Ctrl Pts',(79.3221478673347,0.833284375250171,21.1964192705997));
#24481=CARTESIAN_POINT('Ctrl Pts',(79.2825295794201,4.23315049876201,20.4941634800434));
#24482=CARTESIAN_POINT('Ctrl Pts',(79.2429112915056,7.63301662227385,19.7919076894871));
#24483=CARTESIAN_POINT('Ctrl Pts',(79.203293003591,10.8543683045582,18.2254009957007));
#24484=CARTESIAN_POINT('Ctrl Pts',(79.1636747156764,13.5061574016271,15.9848056645799));
#24485=CARTESIAN_POINT('Ctrl Pts',(79.1240564277619,16.1579464986958,13.7442103334592));
#24486=CARTESIAN_POINT('Ctrl Pts',(79.0844381398473,18.2401730105491,10.8295263650042));
#24487=CARTESIAN_POINT('Ctrl Pts',(79.0448198519327,19.5000701196733,7.59457472277011));
#24488=CARTESIAN_POINT('Ctrl Pts',(79.0052015640181,20.7599672287975,4.35962308053591));
#24489=CARTESIAN_POINT('Ctrl Pts',(78.9655832761036,21.1975349351925,0.804403764522593));
#24490=CARTESIAN_POINT('Ctrl Pts',(78.925964988189,20.7596557725489,-2.63950603280019));
#24491=CARTESIAN_POINT('Ctrl Pts',(78.8863467002744,20.3217766099053,-6.08341583012296));
#24492=CARTESIAN_POINT('Ctrl Pts',(78.8467284123598,19.008450578223,-9.41601610875521));
#24493=CARTESIAN_POINT('Ctrl Pts',(78.8071101244452,16.9791056933766,-12.2327539722279));
#24494=CARTESIAN_POINT('Ctrl Pts',(78.7674918365306,14.9497608085302,-15.0494918357007));
#24495=CARTESIAN_POINT('Ctrl Pts',(78.727873548616,12.2043970705196,-17.3503672840139));
#24496=CARTESIAN_POINT('Ctrl Pts',(78.6882552607015,9.07628122579333,-18.8560711443881));
#24497=CARTESIAN_POINT('Ctrl Pts',(78.6486369727869,5.94816538106711,-20.3617750047622));
#24498=CARTESIAN_POINT('Ctrl Pts',(78.6090186848723,2.43729742962522,-21.0723072771974));
#24499=CARTESIAN_POINT('Ctrl Pts',(78.5694003969577,-1.03012936197627,-20.9014146265153));
#24500=CARTESIAN_POINT('Ctrl Pts',(78.5297821090432,-4.49755615357775,-20.7305219758331));
#24501=CARTESIAN_POINT('Ctrl Pts',(78.4901638211286,-7.92154178533884,-19.6782044020336));
#24502=CARTESIAN_POINT('Ctrl Pts',(78.450545533214,-10.8864398583564,-17.872205434761));
#24503=CARTESIAN_POINT('Ctrl Pts',(78.4109272452994,-13.851337931374,-16.0662064674884));
#24504=CARTESIAN_POINT('Ctrl Pts',(78.3713089573849,-16.357148445648,-13.5065261067426));
#24505=CARTESIAN_POINT('Ctrl Pts',(78.3316906694703,-18.0996846350513,-10.5038905174988));
#24506=CARTESIAN_POINT('Ctrl Pts',(78.2920723815557,-19.8422208244545,-7.50125492825505));
#24507=CARTESIAN_POINT('Ctrl Pts',(78.2524540936411,-20.8214826889869,-4.05566411051326));
#24508=CARTESIAN_POINT('Ctrl Pts',(78.2128358057265,-20.9185951189516,-0.585387172123522));
#24509=CARTESIAN_POINT('Ctrl Pts',(78.2106094862016,-20.9240522780143,-0.390377601760896));
#24510=CARTESIAN_POINT('Ctrl Pts',(78.2083831666768,-20.9267237922488,-0.195290077752758));
#24511=CARTESIAN_POINT('Ctrl Pts',(78.2061568471519,-20.9266265721997,-0.000199885376053199));
#24512=CARTESIAN_POINT('Ctrl Pts',(77.9938431528481,-20.9267713605918,-5.6450652404226E-5));
#24513=CARTESIAN_POINT('Ctrl Pts',(77.9944552259026,-20.9267797066547,-0.0536907309856513));
#24514=CARTESIAN_POINT('Ctrl Pts',(77.995067298957,-20.9265778086015,-0.107324948224965));
#24515=CARTESIAN_POINT('Ctrl Pts',(77.9956793720115,-20.9261652833693,-0.160957545385623));
#24516=CARTESIAN_POINT('Ctrl Pts',(78.035297659926,-20.8994633344748,-3.63249033135252));
#24517=CARTESIAN_POINT('Ctrl Pts',(78.0749159478406,-19.9902927127358,-7.09723544315468));
#24518=CARTESIAN_POINT('Ctrl Pts',(78.1145342357552,-18.3090199720912,-10.1345985840523));
#24519=CARTESIAN_POINT('Ctrl Pts',(78.1541525236698,-16.6277472314466,-13.1719617249499));
#24520=CARTESIAN_POINT('Ctrl Pts',(78.1937708115843,-14.1743723718966,-15.781942894943));
#24521=CARTESIAN_POINT('Ctrl Pts',(78.2333890994989,-11.2467168609356,-17.6477097847924));
#24522=CARTESIAN_POINT('Ctrl Pts',(78.2730073874135,-8.31906134997462,-19.5134766746417));
#24523=CARTESIAN_POINT('Ctrl Pts',(78.3126256753281,-4.91712518760277,-20.6350292843473));
#24524=CARTESIAN_POINT('Ctrl Pts',(78.3522439632427,-1.45387813107363,-20.8762194656575));
#24525=CARTESIAN_POINT('Ctrl Pts',(78.3918622511573,2.00936892545546,-21.1174096469676));
#24526=CARTESIAN_POINT('Ctrl Pts',(78.4314805390718,5.53392687614181,-20.4782373998824));
#24527=CARTESIAN_POINT('Ctrl Pts',(78.4710988269864,8.6919405903041,-19.0362934830532));
#24528=CARTESIAN_POINT('Ctrl Pts',(78.510717114901,11.8499543044664,-17.594349566224));
#24529=CARTESIAN_POINT('Ctrl Pts',(78.5503354028156,14.6414237821046,-15.3496339796508));
#24530=CARTESIAN_POINT('Ctrl Pts',(78.5899536907302,16.7274853827683,-12.5746385064375));
#24531=CARTESIAN_POINT('Ctrl Pts',(78.6295719786448,18.8135469834321,-9.79964303322422));
#24532=CARTESIAN_POINT('Ctrl Pts',(78.6691902665594,20.1942007071214,-6.49436767337088));
#24533=CARTESIAN_POINT('Ctrl Pts',(78.7088085544739,20.7018454567228,-3.06004828136315));
#24534=CARTESIAN_POINT('Ctrl Pts',(78.7484268423885,21.2094902063242,0.37427111064453));
#24535=CARTESIAN_POINT('Ctrl Pts',(78.788045130303,20.8441259818378,3.9376345348067));
#24536=CARTESIAN_POINT('Ctrl Pts',(78.8276634182176,19.6501052836908,7.19747616447438));
#24537=CARTESIAN_POINT('Ctrl Pts',(78.8672817061322,18.4560845855438,10.4573177941421));
#24538=CARTESIAN_POINT('Ctrl Pts',(78.9068999940468,16.4334074137363,13.4136376293154));
#24539=CARTESIAN_POINT('Ctrl Pts',(78.9465182819614,13.8276117386402,15.7075604217756));
#24540=CARTESIAN_POINT('Ctrl Pts',(78.986136569876,11.2218160635441,18.0014832142357));
#24541=CARTESIAN_POINT('Ctrl Pts',(79.0257548577905,8.03290188515943,19.6330089639828));
#24542=CARTESIAN_POINT('Ctrl Pts',(79.0653731457051,4.6479796756686,20.4040825751338));
#24543=CARTESIAN_POINT('Ctrl Pts',(79.1049914336197,1.26305746617771,21.1751561862849));
#24544=CARTESIAN_POINT('Ctrl Pts',(79.1446097215342,-2.31787277441935,21.0857776588399));
#24545=CARTESIAN_POINT('Ctrl Pts',(79.1842280094488,-5.66011273856516,20.1467968815155));
#24546=CARTESIAN_POINT('Ctrl Pts',(79.2238462973634,-9.00235270271097,19.207816104191));
#24547=CARTESIAN_POINT('Ctrl Pts',(79.263464585278,-12.1059023904055,17.4192330769871));
#24548=CARTESIAN_POINT('Ctrl Pts',(79.3030828731926,-14.5940139439646,14.9981684815738));
#24549=CARTESIAN_POINT('Ctrl Pts',(79.3427011611072,-17.0821254975237,12.5771038861606));
#24550=CARTESIAN_POINT('Ctrl Pts',(79.3823194490217,-18.9547989169474,9.52355772253809));
#24551=CARTESIAN_POINT('Ctrl Pts',(79.4219377369363,-19.984705572149,6.2082077923363));
#24552=CARTESIAN_POINT('Ctrl Pts',(79.4459062089069,-20.6077837034092,4.20247064271143));
#24553=CARTESIAN_POINT('Ctrl Pts',(79.4698746808775,-20.9224033728877,2.1009115046599));
#24554=CARTESIAN_POINT('Ctrl Pts',(79.4938431528481,-20.9235342978811,-0.000316448518974899));
#24555=CARTESIAN_POINT('Origin',(80.4,0.,0.));
#24556=CARTESIAN_POINT('',(81.2061568471518,-20.9255032265546,0.000505554818943099));
#24557=CARTESIAN_POINT('',(80.9938431528482,-20.9250582860856,0.000536067210225428));
#24558=CARTESIAN_POINT('',(80.4,-20.925,-2.56257342721584E-15));
#24559=CARTESIAN_POINT('Ctrl Pts',(81.2061568471518,-20.9255032265546,0.000505554818943099));
#24560=CARTESIAN_POINT('Ctrl Pts',(81.1988403645412,-20.9261523161782,0.641741347385084));
#24561=CARTESIAN_POINT('Ctrl Pts',(81.1915238819306,-20.8972595484565,1.28291886862289));
#24562=CARTESIAN_POINT('Ctrl Pts',(81.1842073993199,-20.8383967471104,1.92133310540693));
#24563=CARTESIAN_POINT('Ctrl Pts',(81.1445891114053,-20.5196584222495,5.37830558626897));
#24564=CARTESIAN_POINT('Ctrl Pts',(81.1049708234908,-19.3221526752348,8.75425432232823));
#24565=CARTESIAN_POINT('Ctrl Pts',(81.0653525355762,-17.3912478004877,11.639364236673));
#24566=CARTESIAN_POINT('Ctrl Pts',(81.0257342476617,-15.4603429257406,14.5244741510179));
#24567=CARTESIAN_POINT('Ctrl Pts',(80.9861159597471,-12.7960389232611,16.9187452436483));
#24568=CARTESIAN_POINT('Ctrl Pts',(80.9464976718325,-9.72176249027052,18.5315308049465));
#24569=CARTESIAN_POINT('Ctrl Pts',(80.9068793839179,-6.64748605727993,20.1443163662447));
#24570=CARTESIAN_POINT('Ctrl Pts',(80.8672610960033,-3.16323719377827,20.9756163962107));
#24571=CARTESIAN_POINT('Ctrl Pts',(80.8276428080887,0.308022193045609,20.9245172517911));
#24572=CARTESIAN_POINT('Ctrl Pts',(80.7880245201741,3.77928157986949,20.8734181073715));
#24573=CARTESIAN_POINT('Ctrl Pts',(80.7484062322596,7.23755149001558,19.9399197885663));
#24574=CARTESIAN_POINT('Ctrl Pts',(80.708787944345,10.263023668083,18.2373420508659));
#24575=CARTESIAN_POINT('Ctrl Pts',(80.6691696564305,13.2884958461504,16.5347643131654));
#24576=CARTESIAN_POINT('Ctrl Pts',(80.6295513685158,15.8811702921392,14.0631071565697));
#24577=CARTESIAN_POINT('Ctrl Pts',(80.5899330806012,17.7263156044315,11.1224113835086));
#24578=CARTESIAN_POINT('Ctrl Pts',(80.5503147926867,19.5714609167237,8.18171561044757));
#24579=CARTESIAN_POINT('Ctrl Pts',(80.5106965047721,20.6690770953195,4.77198122092119));
#24580=CARTESIAN_POINT('Ctrl Pts',(80.4710782168576,20.8859216967403,1.30712461898108));
#24581=CARTESIAN_POINT('Ctrl Pts',(80.431459928943,21.102766298161,-2.15773198295897));
#24582=CARTESIAN_POINT('Ctrl Pts',(80.3918416410284,20.4388393224069,-5.67771079731262));
#24583=CARTESIAN_POINT('Ctrl Pts',(80.3522233531138,18.974736568142,-8.82551256650441));
#24584=CARTESIAN_POINT('Ctrl Pts',(80.3126050651992,17.5106338138771,-11.9733143356962));
#24585=CARTESIAN_POINT('Ctrl Pts',(80.2729867772846,15.2463552811015,-14.7489390597261));
#24586=CARTESIAN_POINT('Ctrl Pts',(80.2333684893701,12.4567675491407,-16.8154465334283));
#24587=CARTESIAN_POINT('Ctrl Pts',(80.1937502014555,9.66717981717998,-18.8819540071306));
#24588=CARTESIAN_POINT('Ctrl Pts',(80.1541319135409,6.35228288603402,-20.2393442305052));
#24589=CARTESIAN_POINT('Ctrl Pts',(80.1145136256263,2.91448059740862,-20.7228401224167));
#24590=CARTESIAN_POINT('Ctrl Pts',(80.0748953377118,-0.523321691216679,
-21.2063360143281));
#24591=CARTESIAN_POINT('Ctrl Pts',(80.0352770497972,-4.08402933732142,-20.8159375747763));
#24592=CARTESIAN_POINT('Ctrl Pts',(79.9956587618826,-7.33539890596775,-19.5990362717721));
#24593=CARTESIAN_POINT('Ctrl Pts',(79.956040473968,-10.5867684746141,-18.382134968768));
#24594=CARTESIAN_POINT('Ctrl Pts',(79.9164221860534,-13.5287999658021,-16.3387308023114));
#24595=CARTESIAN_POINT('Ctrl Pts',(79.8768038981389,-15.8043526300411,-13.7168778458229));
#24596=CARTESIAN_POINT('Ctrl Pts',(79.8371856102243,-18.0799052942802,-11.0950248893343));
#24597=CARTESIAN_POINT('Ctrl Pts',(79.7975673223097,-19.6889791315702,-7.89472314281364));
#24598=CARTESIAN_POINT('Ctrl Pts',(79.7579490343951,-20.4362445412743,-4.50446544455035));
#24599=CARTESIAN_POINT('Ctrl Pts',(79.7406849719807,-20.7618728647668,-3.02712698333307));
#24600=CARTESIAN_POINT('Ctrl Pts',(79.7234209095663,-20.9238552147395,-1.51371840994956));
#24601=CARTESIAN_POINT('Ctrl Pts',(79.7061568471518,-20.923342133494,-0.000201647965826224));
#24602=CARTESIAN_POINT('Ctrl Pts',(79.4938431528481,-20.9235342978811,-0.000316448518974899));
#24603=CARTESIAN_POINT('Ctrl Pts',(79.5094929687921,-20.9242727165845,-1.37227836431806));
#24604=CARTESIAN_POINT('Ctrl Pts',(79.5251427847361,-20.7913639781663,-2.74409908871077));
#24605=CARTESIAN_POINT('Ctrl Pts',(79.54079260068,-20.5234078536779,-4.08901343479093));
#24606=CARTESIAN_POINT('Ctrl Pts',(79.5804108885946,-19.8450635890258,-7.49373103493513));
#24607=CARTESIAN_POINT('Ctrl Pts',(79.6200291765092,-18.3012351687421,-10.7260125384424));
#24608=CARTESIAN_POINT('Ctrl Pts',(79.6596474644238,-16.0793318849288,-13.3934830022897));
#24609=CARTESIAN_POINT('Ctrl Pts',(79.6992657523384,-13.8574286011154,-16.0609534661369));
#24610=CARTESIAN_POINT('Ctrl Pts',(79.738884040253,-10.9574504537723,-18.1636128903242));
#24611=CARTESIAN_POINT('Ctrl Pts',(79.7785023281675,-7.73143322910731,-19.446214053696));
#24612=CARTESIAN_POINT('Ctrl Pts',(79.8181206160821,-4.50541600444238,-20.7288152170678));
#24613=CARTESIAN_POINT('Ctrl Pts',(79.8577389039966,-0.953359702455491,
-21.1913581196242));
#24614=CARTESIAN_POINT('Ctrl Pts',(79.8973571919113,2.49354245077003,-20.7776934919282));
#24615=CARTESIAN_POINT('Ctrl Pts',(79.9369754798258,5.94044460399564,-20.3640288642323));
#24616=CARTESIAN_POINT('Ctrl Pts',(79.9765937677405,9.28219260845988,-19.074156706284));
#24617=CARTESIAN_POINT('Ctrl Pts',(80.0162120556551,12.1131231017896,-17.0646579080625));
#24618=CARTESIAN_POINT('Ctrl Pts',(80.0558303435696,14.9440535951194,-15.0551591098409));
#24619=CARTESIAN_POINT('Ctrl Pts',(80.0954486314841,17.2641665773147,-12.3260336713461));
#24620=CARTESIAN_POINT('Ctrl Pts',(80.1350669193987,18.7918175820108,-9.20857713019443));
#24621=CARTESIAN_POINT('Ctrl Pts',(80.1746852073133,20.3194685867068,-6.09112058904278));
#24622=CARTESIAN_POINT('Ctrl Pts',(80.2143034952279,21.0546576139037,-2.58533294523431));
#24623=CARTESIAN_POINT('Ctrl Pts',(80.2539217831425,20.908138181714,0.883209246250315));
#24624=CARTESIAN_POINT('Ctrl Pts',(80.2935400710571,20.7616187495243,4.35175143773489));
#24625=CARTESIAN_POINT('Ctrl Pts',(80.3331583589716,19.7333908579481,7.78304817689562));
#24626=CARTESIAN_POINT('Ctrl Pts',(80.3727766468862,17.9482737283106,10.760565550748));
#24627=CARTESIAN_POINT('Ctrl Pts',(80.4123949348008,16.1631565986731,13.7380829246004));
#24628=CARTESIAN_POINT('Ctrl Pts',(80.4520132227154,13.6211502309744,16.2618209331444));
#24629=CARTESIAN_POINT('Ctrl Pts',(80.49163151063,10.6308352988371,18.0254165457365));
#24630=CARTESIAN_POINT('Ctrl Pts',(80.5312497985445,7.64052036669963,19.7890121583286));
#24631=CARTESIAN_POINT('Ctrl Pts',(80.5708680864591,4.20189687012352,20.7924653749687));
#24632=CARTESIAN_POINT('Ctrl Pts',(80.6104863743737,0.732388135970209,20.9139644356731));
#24633=CARTESIAN_POINT('Ctrl Pts',(80.6501046622882,-2.7371205981831,21.0354634963775));
#24634=CARTESIAN_POINT('Ctrl Pts',(80.6897229502028,-6.23751456991377,20.275008401146));
#24635=CARTESIAN_POINT('Ctrl Pts',(80.7293412381174,-9.34387197592999,18.7249127446763));
#24636=CARTESIAN_POINT('Ctrl Pts',(80.768959526032,-12.4502293819462,17.1748170882065));
#24637=CARTESIAN_POINT('Ctrl Pts',(80.8085778139465,-15.1625502222479,14.8350808704987));
#24638=CARTESIAN_POINT('Ctrl Pts',(80.8481961018611,-17.1515789125002,11.9897306728128));
#24639=CARTESIAN_POINT('Ctrl Pts',(80.8878143897757,-19.1406076027525,9.14438047512686));
#24640=CARTESIAN_POINT('Ctrl Pts',(80.9274326776903,-20.4063441429551,5.79341629746302));
#24641=CARTESIAN_POINT('Ctrl Pts',(80.9670509656049,-20.7951375276788,2.34362027709995));
#24642=CARTESIAN_POINT('Ctrl Pts',(80.975981694686,-20.8827790833909,1.56596946822868));
#24643=CARTESIAN_POINT('Ctrl Pts',(80.9849124237671,-20.9258597481872,0.783296629213236));
#24644=CARTESIAN_POINT('Ctrl Pts',(80.9938431528482,-20.9250582860856,0.000536067210225428));
#24645=CARTESIAN_POINT('Origin',(80.4,0.,0.));
#24646=CARTESIAN_POINT('',(82.7061568471518,-20.9253923844606,-0.000516496948829159));
#24647=CARTESIAN_POINT('',(82.4938431528481,-20.925825242932,-0.000460001030962829));
#24648=CARTESIAN_POINT('',(80.4,-20.925,-2.56257342721584E-15));
#24649=CARTESIAN_POINT('Ctrl Pts',(82.7061568471518,-20.9253923844606,-0.000516496948829159));
#24650=CARTESIAN_POINT('Ctrl Pts',(82.6742598195161,-20.9225376980426,2.7950656564594));
#24651=CARTESIAN_POINT('Ctrl Pts',(82.6423627918805,-20.3586526388534,5.59176473337593));
#24652=CARTESIAN_POINT('Ctrl Pts',(82.6104657642448,-19.2680752408653,8.16526646253917));
#24653=CARTESIAN_POINT('Ctrl Pts',(82.5708474763302,-17.913503591114,11.361731462952));
#24654=CARTESIAN_POINT('Ctrl Pts',(82.5312291884156,-15.7463858988448,14.2138623839457));
#24655=CARTESIAN_POINT('Ctrl Pts',(82.491610900501,-13.0297941397213,16.3754317368549));
#24656=CARTESIAN_POINT('Ctrl Pts',(82.4519926125865,-10.3132023805979,18.5370010897641));
#24657=CARTESIAN_POINT('Ctrl Pts',(82.4123743246719,-7.04713655462023,20.0080088745887));
#24658=CARTESIAN_POINT('Ctrl Pts',(82.3727560367573,-3.62807277037813,20.6098856829618));
#24659=CARTESIAN_POINT('Ctrl Pts',(82.3331377488427,-0.209008986136022,
21.2117624913349));
#24660=CARTESIAN_POINT('Ctrl Pts',(82.2935194609282,3.36305275637049,20.9445083232563));
#24661=CARTESIAN_POINT('Ctrl Pts',(82.2539011730136,6.65449071931628,19.8405658477385));
#24662=CARTESIAN_POINT('Ctrl Pts',(82.214282885099,9.94592868226207,18.7366233722206));
#24663=CARTESIAN_POINT('Ctrl Pts',(82.1746645971844,12.9567428656471,16.7959925892633));
#24664=CARTESIAN_POINT('Ctrl Pts',(82.1350463092699,15.3214428125367,14.2542516476342));
#24665=CARTESIAN_POINT('Ctrl Pts',(82.0954280213553,17.6861427594262,11.712510706005));
#24666=CARTESIAN_POINT('Ctrl Pts',(82.0558097334407,19.4047284698202,8.56965960570394));
#24667=CARTESIAN_POINT('Ctrl Pts',(82.0161914455261,20.2685764158903,5.20721710370577));
#24668=CARTESIAN_POINT('Ctrl Pts',(81.9765731576115,21.1324243619604,1.84477460170779));
#24669=CARTESIAN_POINT('Ctrl Pts',(81.9369548696969,21.1415345437067,-1.73725930198728));
#24670=CARTESIAN_POINT('Ctrl Pts',(81.8973365817824,20.2948010527979,-5.10405232332752));
#24671=CARTESIAN_POINT('Ctrl Pts',(81.8577182938678,19.4480675618891,-8.47084534466805));
#24672=CARTESIAN_POINT('Ctrl Pts',(81.8181000059532,17.745490398325,-11.6223974836537));
#24673=CARTESIAN_POINT('Ctrl Pts',(81.7784817180386,15.3937497713701,-14.1761337419043));
#24674=CARTESIAN_POINT('Ctrl Pts',(81.7388634301241,13.0420091444152,-16.7298700001546));
#24675=CARTESIAN_POINT('Ctrl Pts',(81.6992451422095,10.0411050540696,-18.68579037767));
#24676=CARTESIAN_POINT('Ctrl Pts',(81.6596268542949,6.75532494565278,-19.8064606825791));
#24677=CARTESIAN_POINT('Ctrl Pts',(81.6200085663803,3.46954483723591,-20.9271309874884));
#24678=CARTESIAN_POINT('Ctrl Pts',(81.5803902784657,-0.101111289252063,
-21.2125512197913));
#24679=CARTESIAN_POINT('Ctrl Pts',(81.5407719905512,-3.52319232732012,-20.6280734853409));
#24680=CARTESIAN_POINT('Ctrl Pts',(81.5011537026366,-6.94527336538818,-20.0435957508905));
#24681=CARTESIAN_POINT('Ctrl Pts',(81.461535414722,-10.2187793150363,-18.5892200496866));
#24682=CARTESIAN_POINT('Ctrl Pts',(81.4219171268074,-12.9463308919772,-16.4414967788018));
#24683=CARTESIAN_POINT('Ctrl Pts',(81.3822988388929,-15.6738824689181,-14.2937735079169));
#24684=CARTESIAN_POINT('Ctrl Pts',(81.3426805509783,-17.8554796731518,-11.452702667351));
#24685=CARTESIAN_POINT('Ctrl Pts',(81.3030622630637,-19.2262928239151,-8.26316913423555));
#24686=CARTESIAN_POINT('Ctrl Pts',(81.2707604577598,-20.3439519110395,-5.66266071703114));
#24687=CARTESIAN_POINT('Ctrl Pts',(81.2384586524558,-20.9226375371568,-2.83050967855002));
#24688=CARTESIAN_POINT('Ctrl Pts',(81.2061568471518,-20.9255032265546,0.000505554818943099));
#24689=CARTESIAN_POINT('Ctrl Pts',(80.9938431528482,-20.9250582860856,0.000536067210225428));
#24690=CARTESIAN_POINT('Ctrl Pts',(81.0245307116816,-20.9223043210767,-2.68916715644739));
#24691=CARTESIAN_POINT('Ctrl Pts',(81.0552182705152,-20.4014206134196,-5.37990615234729));
#24692=CARTESIAN_POINT('Ctrl Pts',(81.0859058293486,-19.3899459682665,-7.8714862729993));
#24693=CARTESIAN_POINT('Ctrl Pts',(81.1255241172632,-18.0841107948856,-11.0881689396731));
#24694=CARTESIAN_POINT('Ctrl Pts',(81.1651424051778,-15.960590218879,-13.9729064099583));
#24695=CARTESIAN_POINT('Ctrl Pts',(81.2047606930923,-13.2771638501336,-16.1755130025299));
#24696=CARTESIAN_POINT('Ctrl Pts',(81.2443789810069,-10.5937374813882,-18.3781195951016));
#24697=CARTESIAN_POINT('Ctrl Pts',(81.2839972689215,-7.35040531990409,-19.8985953099598));
#24698=CARTESIAN_POINT('Ctrl Pts',(81.3236155568361,-3.94088377642275,-20.5523656998175));
#24699=CARTESIAN_POINT('Ctrl Pts',(81.3632338447507,-0.531362232941471,
-21.2061360896753));
#24700=CARTESIAN_POINT('Ctrl Pts',(81.4028521326652,3.04434869253702,-20.9932011545327));
#24701=CARTESIAN_POINT('Ctrl Pts',(81.4424704205798,6.35218427850588,-19.9394096123785));
#24702=CARTESIAN_POINT('Ctrl Pts',(81.4820887084944,9.66001986447484,-18.8856180702242));
#24703=CARTESIAN_POINT('Ctrl Pts',(81.521706996409,12.6999801109342,-16.9909699210582));
#24704=CARTESIAN_POINT('Ctrl Pts',(81.5613252843236,15.1030364455882,-14.4854613637793));
#24705=CARTESIAN_POINT('Ctrl Pts',(81.6009435722382,17.5060927802421,-11.9799528065006));
#24706=CARTESIAN_POINT('Ctrl Pts',(81.6405618601527,19.2722452030907,-8.86358384110923));
#24707=CARTESIAN_POINT('Ctrl Pts',(81.6801801480673,20.1870959410649,-5.51465849029216));
#24708=CARTESIAN_POINT('Ctrl Pts',(81.7197984359819,21.1019466790391,-2.16573313947484));
#24709=CARTESIAN_POINT('Ctrl Pts',(81.7594167238965,21.1654957321386,1.4157485967681));
#24710=CARTESIAN_POINT('Ctrl Pts',(81.799035011811,20.3700287177943,4.79502146340806));
#24711=CARTESIAN_POINT('Ctrl Pts',(81.8386532997256,19.5745617034501,8.17429433004782));
#24712=CARTESIAN_POINT('Ctrl Pts',(81.8782715876402,17.9200786216621,11.3513583270846));
#24713=CARTESIAN_POINT('Ctrl Pts',(81.9178898755548,15.607421417739,13.9405415062475));
#24714=CARTESIAN_POINT('Ctrl Pts',(81.9575081634694,13.2947642138159,16.5297246854105));
#24715=CARTESIAN_POINT('Ctrl Pts',(81.9971264513839,10.3239328877575,18.5310270466995));
#24716=CARTESIAN_POINT('Ctrl Pts',(82.0367447392985,7.05556427488541,19.7015053628211));
#24717=CARTESIAN_POINT('Ctrl Pts',(82.0763630272131,3.78719566201337,20.8719836789428));
#24718=CARTESIAN_POINT('Ctrl Pts',(82.1159813151277,0.221289762327655,21.2116379498971));
#24719=CARTESIAN_POINT('Ctrl Pts',(82.1555996030423,-3.20927895989728,20.6792366724662));
#24720=CARTESIAN_POINT('Ctrl Pts',(82.1952178909568,-6.63984768212221,20.1468353950352));
#24721=CARTESIAN_POINT('Ctrl Pts',(82.2348361788714,-9.93507922688639,18.7423785692189));
#24722=CARTESIAN_POINT('Ctrl Pts',(82.274454466786,-12.6949569841818,16.6363568117567));
#24723=CARTESIAN_POINT('Ctrl Pts',(82.3140727547005,-15.4548347414771,14.5303350542944));
#24724=CARTESIAN_POINT('Ctrl Pts',(82.3536910426151,-17.6793587113037,11.7227483651862));
#24725=CARTESIAN_POINT('Ctrl Pts',(82.3933093305297,-19.0984882227091,8.5544168945259));
#24726=CARTESIAN_POINT('Ctrl Pts',(82.4268206046358,-20.2988641236403,5.87447210232992));
#24727=CARTESIAN_POINT('Ctrl Pts',(82.460331878742,-20.9230057193434,2.93642580920009));
#24728=CARTESIAN_POINT('Ctrl Pts',(82.4938431528481,-20.925825242932,-0.000460001030962829));
#24729=CARTESIAN_POINT('Origin',(80.4,0.,0.));
#24730=CARTESIAN_POINT('',(84.2061568471519,-20.9233820813322,0.00023179675235574));
#24731=CARTESIAN_POINT('',(83.9938431528481,-20.9232570769787,0.000107667472307858));
#24732=CARTESIAN_POINT('',(80.4,-20.925,-2.56257342721584E-15));
#24733=CARTESIAN_POINT('Ctrl Pts',(84.2061568471519,-20.9233820813322,0.00023179675235574));
#24734=CARTESIAN_POINT('Ctrl Pts',(84.1892975624057,-20.923959414903,1.4782541776566));
#24735=CARTESIAN_POINT('Ctrl Pts',(84.1724382776596,-20.7695434732479,2.95615766785475));
#24736=CARTESIAN_POINT('Ctrl Pts',(84.1555789929134,-20.4588924176437,4.40045690073148));
#24737=CARTESIAN_POINT('Ctrl Pts',(84.1159607049988,-19.7288814386964,7.79447175393849));
#24738=CARTESIAN_POINT('Ctrl Pts',(84.0763424170842,-18.1361069579233,11.0029167567447));
#24739=CARTESIAN_POINT('Ctrl Pts',(84.0367241291696,-15.8739199552632,13.6363105400914));
#24740=CARTESIAN_POINT('Ctrl Pts',(83.997105841255,-13.6117329526033,16.2697043234381));
#24741=CARTESIAN_POINT('Ctrl Pts',(83.9574875533405,-10.6801334280564,18.3280468873253));
#24742=CARTESIAN_POINT('Ctrl Pts',(83.9178692654259,-7.43499576792306,19.5614707479493));
#24743=CARTESIAN_POINT('Ctrl Pts',(83.8782509775113,-4.18985810778959,20.7948946085734));
#24744=CARTESIAN_POINT('Ctrl Pts',(83.8386326895967,-0.631182312069551,
21.2033997659342));
#24745=CARTESIAN_POINT('Ctrl Pts',(83.7990144016822,2.8090348358294,20.7373967310993));
#24746=CARTESIAN_POINT('Ctrl Pts',(83.7593961137676,6.24925198372836,20.2713936962645));
#24747=CARTESIAN_POINT('Ctrl Pts',(83.719777825853,9.57101048380623,18.9308824692342));
#24748=CARTESIAN_POINT('Ctrl Pts',(83.6801595379384,12.3710735509036,16.8785911464804));
#24749=CARTESIAN_POINT('Ctrl Pts',(83.6405412500238,15.1711366180009,14.8262998237266));
#24750=CARTESIAN_POINT('Ctrl Pts',(83.6009229621092,17.4495042521178,12.0622284052495));
#24751=CARTESIAN_POINT('Ctrl Pts',(83.5613046741946,18.9295995617761,8.92191461081752));
#24752=CARTESIAN_POINT('Ctrl Pts',(83.5216863862801,20.4096948714344,5.78160081638541));
#24753=CARTESIAN_POINT('Ctrl Pts',(83.4820680983655,21.0915178566342,2.26504464599836));
#24754=CARTESIAN_POINT('Ctrl Pts',(83.442449810451,20.8923002762184,-1.20087012629864));
#24755=CARTESIAN_POINT('Ctrl Pts',(83.4028315225364,20.6930826958026,-4.66678489859564));
#24756=CARTESIAN_POINT('Ctrl Pts',(83.3632132346218,19.6128245497712,-8.08205827280259));
#24757=CARTESIAN_POINT('Ctrl Pts',(83.3235949467072,17.7826611455037,-11.0321014533091));
#24758=CARTESIAN_POINT('Ctrl Pts',(83.2839766587926,15.9524977412362,-13.9821446338157));
#24759=CARTESIAN_POINT('Ctrl Pts',(83.244358370878,13.3724290787325,-16.4669576206218));
#24760=CARTESIAN_POINT('Ctrl Pts',(83.2047400829634,10.3556563112174,-18.1849025913216));
#24761=CARTESIAN_POINT('Ctrl Pts',(83.1651217950489,7.33888354370234,-19.9028475620214));
#24762=CARTESIAN_POINT('Ctrl Pts',(83.1255035071344,3.88540667117585,-20.8539245166148));
#24763=CARTESIAN_POINT('Ctrl Pts',(83.0858852192198,0.414452109907308,-20.9226797839212));
#24764=CARTESIAN_POINT('Ctrl Pts',(83.0462669313052,-3.05650245136114,-20.9914350512277));
#24765=CARTESIAN_POINT('Ctrl Pts',(83.0066486433905,-6.54493470137163,-20.1778686312471));
#24766=CARTESIAN_POINT('Ctrl Pts',(82.967030355476,-9.62737490091601,-18.5807414386274));
#24767=CARTESIAN_POINT('Ctrl Pts',(82.9274120675614,-12.7098151004605,-16.9836142460076));
#24768=CARTESIAN_POINT('Ctrl Pts',(82.8877937796469,-15.3862632495388,-14.6029262807486));
#24769=CARTESIAN_POINT('Ctrl Pts',(82.8481754917323,-17.3318184418224,-11.7276753617935));
#24770=CARTESIAN_POINT('Ctrl Pts',(82.8085572038177,-19.2773736341059,-8.85242444283849));
#24771=CARTESIAN_POINT('Ctrl Pts',(82.7689389159031,-20.4920358695947,-5.48261057018744));
#24772=CARTESIAN_POINT('Ctrl Pts',(82.7293206279885,-20.8283541837223,-2.02730409394606));
#24773=CARTESIAN_POINT('Ctrl Pts',(82.7215993677096,-20.8938997026386,-1.3538948667747));
#24774=CARTESIAN_POINT('Ctrl Pts',(82.7138781074307,-20.9260834136405,-0.677238406088404));
#24775=CARTESIAN_POINT('Ctrl Pts',(82.7061568471518,-20.9253923844606,-0.000516496948829159));
#24776=CARTESIAN_POINT('Ctrl Pts',(82.4938431528481,-20.925825242932,-0.000460001030962829));
#24777=CARTESIAN_POINT('Ctrl Pts',(82.4999501666566,-20.9263390661139,-0.535670991221695));
#24778=CARTESIAN_POINT('Ctrl Pts',(82.506057180465,-20.9062184484103,-1.0708434411499));
#24779=CARTESIAN_POINT('Ctrl Pts',(82.5121641942734,-20.8651905092526,-1.60440824321744));
#24780=CARTESIAN_POINT('Ctrl Pts',(82.551782482188,-20.5990282314065,-5.06582565808811));
#24781=CARTESIAN_POINT('Ctrl Pts',(82.5914007701026,-19.4529686227302,-8.45958423561709));
#24782=CARTESIAN_POINT('Ctrl Pts',(82.6310190580172,-17.5661347989447,-11.3737069165516));
#24783=CARTESIAN_POINT('Ctrl Pts',(82.6706373459318,-15.6793009751592,-14.2878295974861));
#24784=CARTESIAN_POINT('Ctrl Pts',(82.7102556338464,-13.0516929362646,-16.7223163818261));
#24785=CARTESIAN_POINT('Ctrl Pts',(82.749873921761,-10.0022827623316,-18.3816386739777));
#24786=CARTESIAN_POINT('Ctrl Pts',(82.7894922096756,-6.95287258839857,-20.0409609661294));
#24787=CARTESIAN_POINT('Ctrl Pts',(82.8291104975901,-3.48166027942724,-20.9251187660927));
#24788=CARTESIAN_POINT('Ctrl Pts',(82.8687287855047,-0.0100252018111283,
-20.9267818905258));
#24789=CARTESIAN_POINT('Ctrl Pts',(82.9083470734192,3.46160987580508,-20.9284450149589));
#24790=CARTESIAN_POINT('Ctrl Pts',(82.9479653613338,6.93366772206606,-20.0476134638616));
#24791=CARTESIAN_POINT('Ctrl Pts',(82.9875836492484,9.98466632863772,-18.3912136386938));
#24792=CARTESIAN_POINT('Ctrl Pts',(83.027201937163,13.0356649352094,-16.734813813526));
#24793=CARTESIAN_POINT('Ctrl Pts',(83.0668202250775,15.6656043020917,-14.3028457142875));
#24794=CARTESIAN_POINT('Ctrl Pts',(83.1064385129921,17.5552293433292,-11.3905321869272));
#24795=CARTESIAN_POINT('Ctrl Pts',(83.1460568009067,19.4448543845667,-8.47821865956675));
#24796=CARTESIAN_POINT('Ctrl Pts',(83.1856750888213,20.5941651001593,-5.08555970408439));
#24797=CARTESIAN_POINT('Ctrl Pts',(83.2252933767359,20.8636437141779,-1.62439889379187));
#24798=CARTESIAN_POINT('Ctrl Pts',(83.2649116646505,21.1331223281966,1.83676191650065));
#24799=CARTESIAN_POINT('Ctrl Pts',(83.304529952565,20.5227688406411,5.36642458160333));
#24800=CARTESIAN_POINT('Ctrl Pts',(83.3441482404796,19.1066756270191,8.5361142964574));
#24801=CARTESIAN_POINT('Ctrl Pts',(83.3837665283941,17.690582413397,11.7058040113115));
#24802=CARTESIAN_POINT('Ctrl Pts',(83.4233848163088,15.4687494737083,14.5155207759169));
#24803=CARTESIAN_POINT('Ctrl Pts',(83.4630031042234,12.710890807854,16.6241858648513));
#24804=CARTESIAN_POINT('Ctrl Pts',(83.502621392138,9.9530321419997,18.7328509537856));
#24805=CARTESIAN_POINT('Ctrl Pts',(83.5422396800525,6.65914774997982,20.1404643670489));
#24806=CARTESIAN_POINT('Ctrl Pts',(83.5818579679671,3.22909070747509,20.6761523016544));
#24807=CARTESIAN_POINT('Ctrl Pts',(83.6214762558816,-0.200966335029539,
21.2118402362598));
#24808=CARTESIAN_POINT('Ctrl Pts',(83.6610945437962,-3.76719602801901,20.8756026922076));
#24809=CARTESIAN_POINT('Ctrl Pts',(83.7007128317108,-7.0366846011192,19.7082564074725));
#24810=CARTESIAN_POINT('Ctrl Pts',(83.7403311196254,-10.3061731742194,18.5409101227374));
#24811=CARTESIAN_POINT('Ctrl Pts',(83.77994940754,-13.2789206274303,16.5424550973195));
#24812=CARTESIAN_POINT('Ctrl Pts',(83.8195676954546,-15.5940575218402,13.9554889131069));
#24813=CARTESIAN_POINT('Ctrl Pts',(83.8591859833692,-17.90919441625,11.3685227288943));
#24814=CARTESIAN_POINT('Ctrl Pts',(83.8988042712837,-19.5667207518589,8.19304538588687));
#24815=CARTESIAN_POINT('Ctrl Pts',(83.9384225591983,-20.3654251549704,4.81453622435309));
#24816=CARTESIAN_POINT('Ctrl Pts',(83.9568960904149,-20.7378514131556,3.23917803129373));
#24817=CARTESIAN_POINT('Ctrl Pts',(83.9753696216315,-20.9235487635752,1.61967575168914));
#24818=CARTESIAN_POINT('Ctrl Pts',(83.9938431528481,-20.9232570769787,0.000107667472307858));
#24819=CARTESIAN_POINT('Origin',(80.4,0.,0.));
#24820=CARTESIAN_POINT('',(85.7061568471519,-20.9266764847855,0.000165093697623506));
#24821=CARTESIAN_POINT('',(85.4938431528481,-20.9264318713289,0.000296857018782903));
#24822=CARTESIAN_POINT('',(80.4,-20.925,-2.56257342721584E-15));
#24823=CARTESIAN_POINT('Ctrl Pts',(85.7061568471519,-20.9266764847855,0.000165093697623506));
#24824=CARTESIAN_POINT('Ctrl Pts',(85.7043353052952,-20.9267437401954,0.159783909494946));
#24825=CARTESIAN_POINT('Ctrl Pts',(85.7025137634386,-20.924955439811,0.319401214298244));
#24826=CARTESIAN_POINT('Ctrl Pts',(85.700692221582,-20.9213021118419,0.478975820845309));
#24827=CARTESIAN_POINT('Ctrl Pts',(85.6610739336674,-20.8418427248384,3.94970183408668));
#24828=CARTESIAN_POINT('Ctrl Pts',(85.6214556457528,-19.8801197477881,7.40022915582282));
#24829=CARTESIAN_POINT('Ctrl Pts',(85.5818373578382,-18.1528791998465,10.4116894233209));
#24830=CARTESIAN_POINT('Ctrl Pts',(85.5422190699236,-16.4256386519049,13.4231496908189));
#24831=CARTESIAN_POINT('Ctrl Pts',(85.502600782009,-13.932880533072,15.9955429040789));
#24832=CARTESIAN_POINT('Ctrl Pts',(85.4629824940945,-10.977207145711,17.8165996523485));
#24833=CARTESIAN_POINT('Ctrl Pts',(85.4233642061799,-8.02153375834987,19.6376564006182));
#24834=CARTESIAN_POINT('Ctrl Pts',(85.3837459182653,-4.60294510246061,20.7073766838974));
#24835=CARTESIAN_POINT('Ctrl Pts',(85.3441276303508,-1.13643242420114,20.8959044129977));
#24836=CARTESIAN_POINT('Ctrl Pts',(85.3045093424362,2.33008025405834,21.0844321420979));
#24837=CARTESIAN_POINT('Ctrl Pts',(85.2648910545216,5.84451695468797,20.3917673170192));
#24838=CARTESIAN_POINT('Ctrl Pts',(85.225272766607,8.98025119151343,18.9019942976723));
#24839=CARTESIAN_POINT('Ctrl Pts',(85.1856544786924,12.1159854283389,17.4122212783253));
#24840=CARTESIAN_POINT('Ctrl Pts',(85.1460361907778,14.8730172013601,15.1253400647103));
#24841=CARTESIAN_POINT('Ctrl Pts',(85.1064179028633,16.9166633514284,12.3189610335593));
#24842=CARTESIAN_POINT('Ctrl Pts',(85.0667996149487,18.9603095014967,9.51258200240819));
#24843=CARTESIAN_POINT('Ctrl Pts',(85.0271813270341,20.290570028612,6.1867051537211));
#24844=CARTESIAN_POINT('Ctrl Pts',(84.9875630391195,20.7459611950595,2.74506720955921));
#24845=CARTESIAN_POINT('Ctrl Pts',(84.9479447512049,21.2013523615071,-0.696570734602592));
#24846=CARTESIAN_POINT('Ctrl Pts',(84.9083264632903,20.7818741672868,-4.2539697742394));
#24847=CARTESIAN_POINT('Ctrl Pts',(84.8687081753757,19.538448146423,-7.49528811463913));
#24848=CARTESIAN_POINT('Ctrl Pts',(84.8290898874612,18.2950221255592,-10.7366064550388));
#24849=CARTESIAN_POINT('Ctrl Pts',(84.7894715995466,16.227648278052,-13.6618440962017));
#24850=CARTESIAN_POINT('Ctrl Pts',(84.7498533116321,13.5872904183904,-15.9158989371707));
#24851=CARTESIAN_POINT('Ctrl Pts',(84.7102350237175,10.9469325587286,-18.1699537781397));
#24852=CARTESIAN_POINT('Ctrl Pts',(84.6706167358029,7.73359068691255,-19.7528258189148));
#24853=CARTESIAN_POINT('Ctrl Pts',(84.6309984478883,4.33734061549098,-20.4723661621495));
#24854=CARTESIAN_POINT('Ctrl Pts',(84.5913801599737,0.941090544069511,-21.1919065053843));
#24855=CARTESIAN_POINT('Ctrl Pts',(84.5517618720591,-2.63806772695736,-21.0481151510788));
#24856=CARTESIAN_POINT('Ctrl Pts',(84.5121435841446,-5.96565099396377,-20.0584473005797));
#24857=CARTESIAN_POINT('Ctrl Pts',(84.47252529623,-9.29323426097029,-19.0687794500805));
#24858=CARTESIAN_POINT('Ctrl Pts',(84.4329070083154,-12.3692425239563,-17.2332351033878));
#24859=CARTESIAN_POINT('Ctrl Pts',(84.3932887204009,-14.8202712494312,-14.7746356972074));
#24860=CARTESIAN_POINT('Ctrl Pts',(84.3536704324863,-17.271299974906,-12.3160362910271));
#24861=CARTESIAN_POINT('Ctrl Pts',(84.3140521445717,-19.0973491628698,-9.23438182535918));
#24862=CARTESIAN_POINT('Ctrl Pts',(84.2744338566571,-20.076750018291,-5.90376224072128));
#24863=CARTESIAN_POINT('Ctrl Pts',(84.2516748534887,-20.6393737040934,-3.99046447674405));
#24864=CARTESIAN_POINT('Ctrl Pts',(84.2289158503203,-20.9226027163257,-1.99500801065722));
#24865=CARTESIAN_POINT('Ctrl Pts',(84.2061568471519,-20.9233820813322,0.00023179675235574));
#24866=CARTESIAN_POINT('Ctrl Pts',(83.9938431528481,-20.9232570769787,0.000107667472307858));
#24867=CARTESIAN_POINT('Ctrl Pts',(84.0149879095461,-20.9229232132446,-1.85364582962594));
#24868=CARTESIAN_POINT('Ctrl Pts',(84.0361326662441,-20.6789244947364,-3.70748553756512));
#24869=CARTESIAN_POINT('Ctrl Pts',(84.0572774229421,-20.192370387916,-5.49531426904058));
#24870=CARTESIAN_POINT('Ctrl Pts',(84.0968957108566,-19.2807287471359,-8.84511462083977));
#24871=CARTESIAN_POINT('Ctrl Pts',(84.1365139987711,-17.5175629949616,-11.9631743443778));
#24872=CARTESIAN_POINT('Ctrl Pts',(84.1761322866857,-15.1169083448479,-14.4709841714991));
#24873=CARTESIAN_POINT('Ctrl Pts',(84.2157505746003,-12.7162536947343,-16.9787939986203));
#24874=CARTESIAN_POINT('Ctrl Pts',(84.255368862515,-9.6781101466813,-18.8763539293247));
#24875=CARTESIAN_POINT('Ctrl Pts',(84.2949871504296,-6.37128573930498,-19.9333142960833));
#24876=CARTESIAN_POINT('Ctrl Pts',(84.3346054383442,-3.06446133192865,-20.9902746628419));
#24877=CARTESIAN_POINT('Ctrl Pts',(84.3742237262587,0.511043934770997,-21.2066354656546));
#24878=CARTESIAN_POINT('Ctrl Pts',(84.4138420141732,3.92119030473388,-20.5561321116685));
#24879=CARTESIAN_POINT('Ctrl Pts',(84.4534603020878,7.33133667469677,-19.9056287576824));
#24880=CARTESIAN_POINT('Ctrl Pts',(84.4930785900024,10.5761241479228,-18.3882612468975));
#24881=CARTESIAN_POINT('Ctrl Pts',(84.532696877917,13.2616596496451,-16.188226713735));
#24882=CARTESIAN_POINT('Ctrl Pts',(84.5723151658316,15.9471951513673,-13.9881921805726));
#24883=CARTESIAN_POINT('Ctrl Pts',(84.6119334537461,18.0734786815857,-11.1054906250329));
#24884=CARTESIAN_POINT('Ctrl Pts',(84.6515517416607,19.3823952283142,-7.89006058352727));
#24885=CARTESIAN_POINT('Ctrl Pts',(84.6911700295753,20.6913117750429,-4.67463054202134));
#24886=CARTESIAN_POINT('Ctrl Pts',(84.7307883174899,21.1828613382816,-1.12647201454918));
#24887=CARTESIAN_POINT('Ctrl Pts',(84.7704066054045,20.7973734556465,2.32369493365209));
#24888=CARTESIAN_POINT('Ctrl Pts',(84.8100248933191,20.4118855730113,5.77386188185326));
#24889=CARTESIAN_POINT('Ctrl Pts',(84.8496431812336,19.1493602445025,9.12603725078375));
#24890=CARTESIAN_POINT('Ctrl Pts',(84.8892614691482,17.1630586583245,11.9732918735502));
#24891=CARTESIAN_POINT('Ctrl Pts',(84.9288797570627,15.1767570721465,14.8205464963164));
#24892=CARTESIAN_POINT('Ctrl Pts',(84.9684980449774,12.4666792282994,17.1628803729186));
#24893=CARTESIAN_POINT('Ctrl Pts',(85.0081163328919,9.36180842802518,18.7159515856198));
#24894=CARTESIAN_POINT('Ctrl Pts',(85.0477346208065,6.25693762775077,20.2690227983212));
#24895=CARTESIAN_POINT('Ctrl Pts',(85.0873529087211,2.75727387104925,21.0328313471215));
#24896=CARTESIAN_POINT('Ctrl Pts',(85.1269711966357,-0.712349681463435,
20.9146565529924));
#24897=CARTESIAN_POINT('Ctrl Pts',(85.1665894845502,-4.18197323397612,20.7964817588633));
#24898=CARTESIAN_POINT('Ctrl Pts',(85.2062077724648,-7.62155658229993,19.7963236218048));
#24899=CARTESIAN_POINT('Ctrl Pts',(85.2458260603794,-10.6135598807076,18.035593903638));
#24900=CARTESIAN_POINT('Ctrl Pts',(85.285444348294,-13.6055631791152,16.2748641854711));
#24901=CARTESIAN_POINT('Ctrl Pts',(85.3250626362085,-16.1499864276067,13.7535628861959));
#24902=CARTESIAN_POINT('Ctrl Pts',(85.3646809241231,-17.9379555612003,10.7777572380672));
#24903=CARTESIAN_POINT('Ctrl Pts',(85.4042992120377,-19.725924694794,7.80195158993853));
#24904=CARTESIAN_POINT('Ctrl Pts',(85.4439174999523,-20.7574397134897,4.37164159295638));
#24905=CARTESIAN_POINT('Ctrl Pts',(85.4835357878669,-20.9072823631693,0.903241376941042));
#24906=CARTESIAN_POINT('Ctrl Pts',(85.4869715761939,-20.9202770596534,0.602453796176518));
#24907=CARTESIAN_POINT('Ctrl Pts',(85.490407364521,-20.9266409150071,0.301379748239037));
#24908=CARTESIAN_POINT('Ctrl Pts',(85.4938431528481,-20.9264318713289,0.000296857018782903));
#24909=CARTESIAN_POINT('Origin',(80.4,0.,0.));
#24910=CARTESIAN_POINT('',(87.2061568471519,-20.9239756446721,-0.00045287493121049));
#24911=CARTESIAN_POINT('',(86.9938431528481,-20.9243500731069,-0.000510630017847893));
#24912=CARTESIAN_POINT('',(80.4,-20.925,-2.56257342721584E-15));
#24913=CARTESIAN_POINT('Ctrl Pts',(87.2061568471519,-20.9239756446721,-0.00045287493121049));
#24914=CARTESIAN_POINT('Ctrl Pts',(87.1797547602702,-20.9221409849285,2.3139812699255));
#24915=CARTESIAN_POINT('Ctrl Pts',(87.1533526733885,-20.5391101652039,4.62900771036594));
#24916=CARTESIAN_POINT('Ctrl Pts',(87.1269505865068,-19.7855330252692,6.81637607515132));
#24917=CARTESIAN_POINT('Ctrl Pts',(87.0873322985922,-18.6547346823365,10.0986844032635));
#24918=CARTESIAN_POINT('Ctrl Pts',(87.0477140106776,-16.6895687983901,13.093542151339));
#24919=CARTESIAN_POINT('Ctrl Pts',(87.008095722763,-14.1285919010428,15.437395855056));
#24920=CARTESIAN_POINT('Ctrl Pts',(86.9684774348485,-11.5676150036958,17.7812495587728));
#24921=CARTESIAN_POINT('Ctrl Pts',(86.9288591469339,-8.41082709294795,19.4740992181312));
#24922=CARTESIAN_POINT('Ctrl Pts',(86.8892408590193,-5.04143875094444,20.310445470555));
#24923=CARTESIAN_POINT('Ctrl Pts',(86.8496225711047,-1.67205040894083,21.1467917229788));
#24924=CARTESIAN_POINT('Ctrl Pts',(86.8100042831901,1.90993836431854,21.1266345684681));
#24925=CARTESIAN_POINT('Ctrl Pts',(86.7703859952755,5.26970076328099,20.252420935715));
#24926=CARTESIAN_POINT('Ctrl Pts',(86.730767707361,8.62946316224335,19.378207302962));
#24927=CARTESIAN_POINT('Ctrl Pts',(86.6911494194465,11.7669991869089,17.6499371919668));
#24928=CARTESIAN_POINT('Ctrl Pts',(86.6515311315319,14.3014352909681,15.2774097447887));
#24929=CARTESIAN_POINT('Ctrl Pts',(86.6119128436173,16.8358713950276,12.9048822976105));
#24930=CARTESIAN_POINT('Ctrl Pts',(86.5722945557027,18.7672075784806,9.88809751424954));
#24931=CARTESIAN_POINT('Ctrl Pts',(86.5326762677881,19.8609939878359,6.59327063808692));
#24932=CARTESIAN_POINT('Ctrl Pts',(86.4930579798735,20.9547803971911,3.29844376192457));
#24933=CARTESIAN_POINT('Ctrl Pts',(86.453439691959,21.2110170324486,-0.274425207039511));
#24934=CARTESIAN_POINT('Ctrl Pts',(86.4138214040444,20.598598671167,-3.69161653968933));
#24935=CARTESIAN_POINT('Ctrl Pts',(86.3742031161298,19.9861803098854,-7.10880787233935));
#24936=CARTESIAN_POINT('Ctrl Pts',(86.3345848282152,18.5051069520648,-10.3703215686751));
#24937=CARTESIAN_POINT('Ctrl Pts',(86.2949665403006,16.3351698917978,-13.0802341148015));
#24938=CARTESIAN_POINT('Ctrl Pts',(86.255348252386,14.1652328315308,-15.7901466609278));
#24939=CARTESIAN_POINT('Ctrl Pts',(86.2157299644714,11.3064320688171,-17.9484580568446));
#24940=CARTESIAN_POINT('Ctrl Pts',(86.1761116765569,8.10580476151847,-19.2931653457917));
#24941=CARTESIAN_POINT('Ctrl Pts',(86.1364933886423,4.90517745421972,-20.6378726347388));
#24942=CARTESIAN_POINT('Ctrl Pts',(86.0968751007277,1.36272360233598,-21.1689758167164));
#24943=CARTESIAN_POINT('Ctrl Pts',(86.0572568128131,-2.09152923409976,-20.8220029141007));
#24944=CARTESIAN_POINT('Ctrl Pts',(86.0176385248986,-5.5457820705354,-20.475030011485));
#24945=CARTESIAN_POINT('Ctrl Pts',(85.978020236984,-8.9118338915228,-19.2499810242761));
#24946=CARTESIAN_POINT('Ctrl Pts',(85.9384019490694,-11.7810710320579,-17.2955677914753));
#24947=CARTESIAN_POINT('Ctrl Pts',(85.8987836611549,-14.650308172593,-15.3411545586745));
#24948=CARTESIAN_POINT('Ctrl Pts',(85.8591653732403,-17.0227306326758,-12.6573770802819));
#24949=CARTESIAN_POINT('Ctrl Pts',(85.8195470853257,-18.6103439642389,-9.57002598871229));
#24950=CARTESIAN_POINT('Ctrl Pts',(85.7817503392677,-20.1249631234685,-6.62462296040961));
#24951=CARTESIAN_POINT('Ctrl Pts',(85.7439535932098,-20.9252809441659,-3.31190364893342));
#24952=CARTESIAN_POINT('Ctrl Pts',(85.7061568471519,-20.9266764847855,0.000165093697623506));
#24953=CARTESIAN_POINT('Ctrl Pts',(85.4938431528481,-20.9264318713289,0.000296857018782903));
#24954=CARTESIAN_POINT('Ctrl Pts',(85.5300256524356,-20.9242304194112,-3.17042571092434));
#24955=CARTESIAN_POINT('Ctrl Pts',(85.5662081520231,-20.1930730044325,-6.34212902779996));
#24956=CARTESIAN_POINT('Ctrl Pts',(85.6023906516106,-18.8006318920486,-9.19056805959208));
#24957=CARTESIAN_POINT('Ctrl Pts',(85.6420089395252,-17.2759684905849,-12.3094868450616));
#24958=CARTESIAN_POINT('Ctrl Pts',(85.6816272274398,-14.9584714069941,-15.0408339809522));
#24959=CARTESIAN_POINT('Ctrl Pts',(85.7212455153544,-12.1294675569991,-17.0530442321017));
#24960=CARTESIAN_POINT('Ctrl Pts',(85.7608638032689,-9.30046370700389,-19.0652544832512));
#24961=CARTESIAN_POINT('Ctrl Pts',(85.8004820911835,-5.95995309060449,-20.3583278496595));
#24962=CARTESIAN_POINT('Ctrl Pts',(85.8401003790981,-2.51344886046267,-20.7752948384409));
#24963=CARTESIAN_POINT('Ctrl Pts',(85.8797186670126,0.93305536967895,-21.1922618272222));
#24964=CARTESIAN_POINT('Ctrl Pts',(85.9193369549272,4.48555321356299,-20.7331224383767));
#24965=CARTESIAN_POINT('Ctrl Pts',(85.9589552428418,7.71279784520256,-19.4536127800814));
#24966=CARTESIAN_POINT('Ctrl Pts',(85.9985735307564,10.9400424768422,-18.1741031217861));
#24967=CARTESIAN_POINT('Ctrl Pts',(86.038191818671,13.8420338962374,-16.0742231940409));
#24968=CARTESIAN_POINT('Ctrl Pts',(86.0778101065855,16.0664919209217,-13.4088828077982));
#24969=CARTESIAN_POINT('Ctrl Pts',(86.1174283945001,18.2909499456059,-10.7435424215556));
#24970=CARTESIAN_POINT('Ctrl Pts',(86.1570466824147,19.8378745755793,-7.5127415768156));
#24971=CARTESIAN_POINT('Ctrl Pts',(86.1966649703293,20.5194806619033,-4.10867547563538));
#24972=CARTESIAN_POINT('Ctrl Pts',(86.2362832582439,21.2010867482273,-0.704609374455165));
#24973=CARTESIAN_POINT('Ctrl Pts',(86.2759015461584,21.0173742909019,2.87272198316526));
#24974=CARTESIAN_POINT('Ctrl Pts',(86.315519834073,19.9906446163735,6.18905716730465));
#24975=CARTESIAN_POINT('Ctrl Pts',(86.3551381219876,18.9639149418451,9.50539235144405));
#24976=CARTESIAN_POINT('Ctrl Pts',(86.3947564099022,17.0941680501136,12.5607313621024));
#24977=CARTESIAN_POINT('Ctrl Pts',(86.4343746978168,14.6083773125621,14.9841787593491));
#24978=CARTESIAN_POINT('Ctrl Pts',(86.4739929857313,12.1225865750108,17.4076261565957));
#24979=CARTESIAN_POINT('Ctrl Pts',(86.5136112736459,9.02075199163955,19.1991819404306));
#24980=CARTESIAN_POINT('Ctrl Pts',(86.5532295615605,5.67941321921927,20.1413645586307));
#24981=CARTESIAN_POINT('Ctrl Pts',(86.5928478494751,2.33807444679899,21.0835471768309));
#24982=CARTESIAN_POINT('Ctrl Pts',(86.6324661373897,-1.24276851467036,21.1763566293961));
#24983=CARTESIAN_POINT('Ctrl Pts',(86.6720844253043,-4.62842795266854,20.4085265388089));
#24984=CARTESIAN_POINT('Ctrl Pts',(86.7117027132188,-8.01408739066692,19.6406964482215));
#24985=CARTESIAN_POINT('Ctrl Pts',(86.7513210011334,-11.2045633051941,18.0122268144815));
#24986=CARTESIAN_POINT('Ctrl Pts',(86.7909392890479,-13.8125556409113,15.7208017437101));
#24987=CARTESIAN_POINT('Ctrl Pts',(86.8305575769625,-16.4205479766283,13.4293766729389));
#24988=CARTESIAN_POINT('Ctrl Pts',(86.8701758648772,-18.4460567335353,10.4749961651365));
#24989=CARTESIAN_POINT('Ctrl Pts',(86.9097941527917,-19.6432002078817,7.21630004859733));
#24990=CARTESIAN_POINT('Ctrl Pts',(86.9378104861439,-20.4897681039995,4.91189161754273));
#24991=CARTESIAN_POINT('Ctrl Pts',(86.965826819496,-20.9220950074049,2.45530394562074));
#24992=CARTESIAN_POINT('Ctrl Pts',(86.9938431528481,-20.9243500731069,-0.000510630017847893));
#24993=CARTESIAN_POINT('Origin',(80.4,0.,0.));
#24994=CARTESIAN_POINT('',(88.7061568471518,-20.924409432792,0.000516573290169631));
#24995=CARTESIAN_POINT('',(88.4938431528482,-20.9240272266393,0.000463189924240194));
#24996=CARTESIAN_POINT('',(80.4,-20.925,-2.56257342721584E-15));
#24997=CARTESIAN_POINT('Ctrl Pts',(88.7061568471518,-20.924409432792,0.000516573290169631));
#24998=CARTESIAN_POINT('Ctrl Pts',(88.6947925031596,-20.9253390160846,0.996667419708051));
#24999=CARTESIAN_POINT('Ctrl Pts',(88.6834281591675,-20.8554826568381,1.99268898101036));
#25000=CARTESIAN_POINT('Ctrl Pts',(88.6720638151753,-20.71375329641,2.97837611248698));
#25001=CARTESIAN_POINT('Ctrl Pts',(88.6324455272608,-20.2196574989527,6.41467094793555));
#25002=CARTESIAN_POINT('Ctrl Pts',(88.5928272393462,-18.852050566816,9.72536591451949));
#25003=CARTESIAN_POINT('Ctrl Pts',(88.5532089514317,-16.7769498136232,12.5085672578046));
#25004=CARTESIAN_POINT('Ctrl Pts',(88.5135906635171,-14.7018490604304,15.2917686010898));
#25005=CARTESIAN_POINT('Ctrl Pts',(88.4739723756024,-11.9192544861816,17.5474763210762));
#25006=CARTESIAN_POINT('Ctrl Pts',(88.4343540876879,-8.76695238403727,19.0018642713807));
#25007=CARTESIAN_POINT('Ctrl Pts',(88.3947357997733,-5.61465028189307,20.4562522216852));
#25008=CARTESIAN_POINT('Ctrl Pts',(88.3551175118588,-2.09264065185337,21.1093204023079));
#25009=CARTESIAN_POINT('Ctrl Pts',(88.3154992239442,1.3715307225796,20.881791191584));
#25010=CARTESIAN_POINT('Ctrl Pts',(88.2758809360296,4.83570209701267,20.65426198086));
#25011=CARTESIAN_POINT('Ctrl Pts',(88.2362626481149,8.24203521583906,19.5461353787892));
#25012=CARTESIAN_POINT('Ctrl Pts',(88.1966443602004,11.1770265639827,17.6919297161148));
#25013=CARTESIAN_POINT('Ctrl Pts',(88.1570260722858,14.1120179121264,15.8377240534403));
#25014=CARTESIAN_POINT('Ctrl Pts',(88.1174077843713,16.5756674895873,13.2374393301622));
#25015=CARTESIAN_POINT('Ctrl Pts',(88.0777894964567,18.2689065545072,10.2067307789809));
#25016=CARTESIAN_POINT('Ctrl Pts',(88.0381712085422,19.962145619427,7.17602222779963));
#25017=CARTESIAN_POINT('Ctrl Pts',(87.9985529206275,20.8849741718059,3.71488984871517));
#25018=CARTESIAN_POINT('Ctrl Pts',(87.9589346327129,20.9253676864696,0.243489379575099));
#25019=CARTESIAN_POINT('Ctrl Pts',(87.9193163447983,20.9657612011333,-3.22791108956507));
#25020=CARTESIAN_POINT('Ctrl Pts',(87.8796980568838,20.123719678082,-6.70957964876064));
#25021=CARTESIAN_POINT('Ctrl Pts',(87.8400797689692,18.501460697768,-9.77886762058159));
#25022=CARTESIAN_POINT('Ctrl Pts',(87.8004614810546,16.8792017174542,-12.8481555924023));
#25023=CARTESIAN_POINT('Ctrl Pts',(87.76084319314,14.4767252798779,-15.5050629768482));
#25024=CARTESIAN_POINT('Ctrl Pts',(87.7212249052254,11.5856741625279,-17.4270609711346));
#25025=CARTESIAN_POINT('Ctrl Pts',(87.6816066173109,8.69462304517777,-19.3490589654212));
#25026=CARTESIAN_POINT('Ctrl Pts',(87.6419883293963,5.31499724805383,-20.5361475695483));
#25027=CARTESIAN_POINT('Ctrl Pts',(87.6023700414818,1.85705821594267,-20.8442230527912));
#25028=CARTESIAN_POINT('Ctrl Pts',(87.5627517535672,-1.60088081616848,-21.1522985360341));
#25029=CARTESIAN_POINT('Ctrl Pts',(87.5231334656526,-5.13713308326719,-20.5813608983927));
#25030=CARTESIAN_POINT('Ctrl Pts',(87.483515177738,-8.32242385160441,-19.2007177242456));
#25031=CARTESIAN_POINT('Ctrl Pts',(87.4438968898234,-11.5077146199416,-17.8200745500985));
#25032=CARTESIAN_POINT('Ctrl Pts',(87.4042786019088,-14.3420438895175,-15.6297258394458));
#25033=CARTESIAN_POINT('Ctrl Pts',(87.3646603139942,-16.4813451597965,-12.8955636408637));
#25034=CARTESIAN_POINT('Ctrl Pts',(87.3250420260797,-18.6206464300755,-10.1614014422816));
#25035=CARTESIAN_POINT('Ctrl Pts',(87.2854237381651,-20.0649197010575,-6.88342575577012));
#25036=CARTESIAN_POINT('Ctrl Pts',(87.2458054502505,-20.6388409355891,-3.45955845844006));
#25037=CARTESIAN_POINT('Ctrl Pts',(87.2325892492176,-20.8302943984184,-2.31739606593537));
#25038=CARTESIAN_POINT('Ctrl Pts',(87.2193730481847,-20.9248940278327,-1.15899867749903));
#25039=CARTESIAN_POINT('Ctrl Pts',(87.2061568471519,-20.9239756446721,-0.00045287493121049));
#25040=CARTESIAN_POINT('Ctrl Pts',(86.9938431528481,-20.9243500731069,-0.000510630017847893));
#25041=CARTESIAN_POINT('Ctrl Pts',(87.0054451074106,-20.9252839272798,-1.01749771259551));
#25042=CARTESIAN_POINT('Ctrl Pts',(87.017047061973,-20.8524646044492,-2.03435221660832));
#25043=CARTESIAN_POINT('Ctrl Pts',(87.0286490165354,-20.7047678525638,-3.04021199421177));
#25044=CARTESIAN_POINT('Ctrl Pts',(87.06826730445,-20.2004138311137,-6.47501619520576));
#25045=CARTESIAN_POINT('Ctrl Pts',(87.1078855923646,-18.8229275964278,-9.78161287191766));
#25046=CARTESIAN_POINT('Ctrl Pts',(87.1475038802792,-16.7395257360041,-12.5586057718189));
#25047=CARTESIAN_POINT('Ctrl Pts',(87.1871221681938,-14.6561238755806,-15.3355986717201));
#25048=CARTESIAN_POINT('Ctrl Pts',(87.2267404561083,-11.8668063894195,-17.5829877948106));
#25049=CARTESIAN_POINT('Ctrl Pts',(87.2663587440229,-8.71017568220549,-19.0279568105308));
#25050=CARTESIAN_POINT('Ctrl Pts',(87.3059770319375,-5.55354497499143,-20.472925826251));
#25051=CARTESIAN_POINT('Ctrl Pts',(87.3455953198521,-2.0296010467245,-21.1154747346007));
#25052=CARTESIAN_POINT('Ctrl Pts',(87.3852136077667,1.43387550967048,-20.8776028753561));
#25053=CARTESIAN_POINT('Ctrl Pts',(87.4248318956813,4.89735206606537,-20.6397310161114));
#25054=CARTESIAN_POINT('Ctrl Pts',(87.4644501835958,8.30036125058831,-19.5214383892724));
#25055=CARTESIAN_POINT('Ctrl Pts',(87.5040684715104,11.2298030490743,-17.6584774054081));
#25056=CARTESIAN_POINT('Ctrl Pts',(87.5436867594249,14.1592448475604,-15.7955164215438));
#25057=CARTESIAN_POINT('Ctrl Pts',(87.5833050473396,16.6151192600096,-13.1878870806542));
#25058=CARTESIAN_POINT('Ctrl Pts',(87.6229233352542,18.299301391789,-10.1521361974108));
#25059=CARTESIAN_POINT('Ctrl Pts',(87.6625416231687,19.9834835235684,-7.11638531416741));
#25060=CARTESIAN_POINT('Ctrl Pts',(87.7021599110832,20.8959733746781,-3.65251288857022));
#25061=CARTESIAN_POINT('Ctrl Pts',(87.7417781989978,20.9260014614113,-0.181007279742066));
#25062=CARTESIAN_POINT('Ctrl Pts',(87.7813964869124,20.9560295481446,3.29049832908599));
#25063=CARTESIAN_POINT('Ctrl Pts',(87.8210147748271,20.1035958705014,6.769637121145));
#25064=CARTESIAN_POINT('Ctrl Pts',(87.8606330627417,18.4721795392379,9.8340675139267));
#25065=CARTESIAN_POINT('Ctrl Pts',(87.9002513506563,16.8407632079744,12.8984979067085));
#25066=CARTESIAN_POINT('Ctrl Pts',(87.9398696385707,14.4303642230905,15.5482199002129));
#25067=CARTESIAN_POINT('Ctrl Pts',(87.9794879264853,11.5335871004151,17.4615769446934));
#25068=CARTESIAN_POINT('Ctrl Pts',(88.0191062143999,8.63680997773975,19.3749339891738));
#25069=CARTESIAN_POINT('Ctrl Pts',(88.0587245023145,5.25365471727298,20.5519260846302));
#25070=CARTESIAN_POINT('Ctrl Pts',(88.0983427902291,1.79481121441017,20.8496751414245));
#25071=CARTESIAN_POINT('Ctrl Pts',(88.1379610781437,-1.66403228845263,21.1474241982189));
#25072=CARTESIAN_POINT('Ctrl Pts',(88.1775793660582,-5.19856403371147,20.5659302163512));
#25073=CARTESIAN_POINT('Ctrl Pts',(88.2171976539728,-8.37971814617746,19.1757822419043));
#25074=CARTESIAN_POINT('Ctrl Pts',(88.2568159418873,-11.5608722586435,17.7856342674574));
#25075=CARTESIAN_POINT('Ctrl Pts',(88.296434229802,-14.3886487383166,15.5868323004313));
#25076=CARTESIAN_POINT('Ctrl Pts',(88.3360525177166,-16.5197765446363,12.8462945518773));
#25077=CARTESIAN_POINT('Ctrl Pts',(88.3756708056312,-18.650904350956,10.1057568033234));
#25078=CARTESIAN_POINT('Ctrl Pts',(88.4152890935457,-20.0853834839222,6.82348327324171));
#25079=CARTESIAN_POINT('Ctrl Pts',(88.4549073814603,-20.6490788419189,3.39791756499875));
#25080=CARTESIAN_POINT('Ctrl Pts',(88.4678859719229,-20.8337403096959,2.27573342302018));
#25081=CARTESIAN_POINT('Ctrl Pts',(88.4808645623856,-20.9249529238808,1.13817176694133));
#25082=CARTESIAN_POINT('Ctrl Pts',(88.4938431528482,-20.9240272266393,0.000463189924240194));
#25083=CARTESIAN_POINT('Origin',(80.4,0.,0.));
#25084=CARTESIAN_POINT('',(90.2061568471519,-20.9263865279884,-0.000314477239331534));
#25085=CARTESIAN_POINT('',(89.9938431528482,-20.9266482192657,-0.000185637335865005));
#25086=CARTESIAN_POINT('',(80.4,-20.925,-2.56257342721584E-15));
#25087=CARTESIAN_POINT('Ctrl Pts',(90.2061568471519,-20.9263865279884,-0.000314477239331534));
#25088=CARTESIAN_POINT('Ctrl Pts',(90.1702119581346,-20.9240965220108,3.14960571920385));
#25089=CARTESIAN_POINT('Ctrl Pts',(90.1342670691174,-20.2028316475124,6.30053922034308));
#25090=CARTESIAN_POINT('Ctrl Pts',(90.0983221801002,-18.8279901652861,9.13439032196935));
#25091=CARTESIAN_POINT('Ctrl Pts',(90.0587038921856,-17.3126463384168,12.257847701334));
#25092=CARTESIAN_POINT('Ctrl Pts',(90.019085604271,-15.0033151063425,14.9961024454623));
#25093=CARTESIAN_POINT('Ctrl Pts',(89.9794673163564,-12.1803321236277,17.0167508358796));
#25094=CARTESIAN_POINT('Ctrl Pts',(89.9398490284419,-9.35734914091304,19.0373992262967));
#25095=CARTESIAN_POINT('Ctrl Pts',(89.9002307405273,-6.02071440755794,20.3404412630028));
#25096=CARTESIAN_POINT('Ctrl Pts',(89.8606124526128,-2.57547056647811,20.7676973057411));
#25097=CARTESIAN_POINT('Ctrl Pts',(89.8209941646982,0.86977327460192,21.1949533484794));
#25098=CARTESIAN_POINT('Ctrl Pts',(89.7813758767836,4.42362622340663,20.7464233972499));
#25099=CARTESIAN_POINT('Ctrl Pts',(89.741757588869,7.65467695105084,19.4765556660559));
#25100=CARTESIAN_POINT('Ctrl Pts',(89.7021393009544,10.885727678695,18.2066879348619));
#25101=CARTESIAN_POINT('Ctrl Pts',(89.6625210130398,13.7939761851787,16.1154824237035));
#25102=CARTESIAN_POINT('Ctrl Pts',(89.6229027251253,16.0263827258295,13.4567959274051));
#25103=CARTESIAN_POINT('Ctrl Pts',(89.5832844372107,18.2587892664803,10.7981094311067));
#25104=CARTESIAN_POINT('Ctrl Pts',(89.5436661492961,19.8153538412981,7.57194194966831));
#25105=CARTESIAN_POINT('Ctrl Pts',(89.5040478613815,20.5071210828747,4.16992623257053));
#25106=CARTESIAN_POINT('Ctrl Pts',(89.464429573467,21.1988883244512,0.767910515472837));
#25107=CARTESIAN_POINT('Ctrl Pts',(89.4248112855524,21.0258582327863,-2.80995343728448));
#25108=CARTESIAN_POINT('Ctrl Pts',(89.3851929976378,20.0090353749829,-6.12933954435845));
#25109=CARTESIAN_POINT('Ctrl Pts',(89.3455747097232,18.9922125171794,-9.44872565143252));
#25110=CARTESIAN_POINT('Ctrl Pts',(89.3059564218086,17.1315968932374,-12.5096339128235));
#25111=CARTESIAN_POINT('Ctrl Pts',(89.266338133894,14.653053406303,-14.9404928221193));
#25112=CARTESIAN_POINT('Ctrl Pts',(89.2267198459794,12.1745099193687,-17.3713517314152));
#25113=CARTESIAN_POINT('Ctrl Pts',(89.1871015580649,9.07803856944216,-19.172161288616));
#25114=CARTESIAN_POINT('Ctrl Pts',(89.1474832701503,5.73952795673904,-20.1243166026441));
#25115=CARTESIAN_POINT('Ctrl Pts',(89.1078649822357,2.40101734403591,-21.0764719166722));
#25116=CARTESIAN_POINT('Ctrl Pts',(89.0682466943211,-1.17953253144373,-21.1799729875277));
#25117=CARTESIAN_POINT('Ctrl Pts',(89.0286284064066,-4.5674695356959,-20.4222555545031));
#25118=CARTESIAN_POINT('Ctrl Pts',(88.989010118492,-7.95540653994797,-19.6645381214785));
#25119=CARTESIAN_POINT('Ctrl Pts',(88.9493918305774,-11.1507306729725,-18.0456021845738));
#25120=CARTESIAN_POINT('Ctrl Pts',(88.9097735426628,-13.7655533417224,-15.761974530108));
#25121=CARTESIAN_POINT('Ctrl Pts',(88.8701552547482,-16.3803760104724,-13.4783468756422));
#25122=CARTESIAN_POINT('Ctrl Pts',(88.8305369668336,-18.4146972149476,-10.5300275036151));
#25123=CARTESIAN_POINT('Ctrl Pts',(88.7909186789191,-19.6215654857963,-7.27492046544498));
#25124=CARTESIAN_POINT('Ctrl Pts',(88.7626647349967,-20.4822485248974,-4.95352757950775));
#25125=CARTESIAN_POINT('Ctrl Pts',(88.7344107910742,-20.9220983100175,-2.47610593764071));
#25126=CARTESIAN_POINT('Ctrl Pts',(88.7061568471518,-20.924409432792,0.000516573290169631));
#25127=CARTESIAN_POINT('Ctrl Pts',(88.4938431528482,-20.9240272266393,0.000463189924240194));
#25128=CARTESIAN_POINT('Ctrl Pts',(88.5204828503002,-20.922127151703,-2.33478364350704));
#25129=CARTESIAN_POINT('Ctrl Pts',(88.5471225477521,-20.5320375909792,-4.67064947204017));
#25130=CARTESIAN_POINT('Ctrl Pts',(88.5737622452041,-19.7650918416665,-6.87542328070042));
#25131=CARTESIAN_POINT('Ctrl Pts',(88.6133805331186,-18.6244979003904,-10.1543405317518));
#25132=CARTESIAN_POINT('Ctrl Pts',(88.6529988210332,-16.6503984348114,-13.1433171474505));
#25133=CARTESIAN_POINT('Ctrl Pts',(88.6926171089477,-14.0824344429329,-15.479513589219));
#25134=CARTESIAN_POINT('Ctrl Pts',(88.7322353968623,-11.5144704510542,-17.8157100309874));
#25135=CARTESIAN_POINT('Ctrl Pts',(88.771853684777,-8.35264193287629,-19.4991262988255));
#25136=CARTESIAN_POINT('Ctrl Pts',(88.8114719726915,-4.98077136280933,-20.3254081737541));
#25137=CARTESIAN_POINT('Ctrl Pts',(88.8510902606061,-1.60890079274246,-21.1516900486826));
#25138=CARTESIAN_POINT('Ctrl Pts',(88.8907085485206,1.97301182921349,-21.1208375307015));
#25139=CARTESIAN_POINT('Ctrl Pts',(88.9303268364352,5.33014894170708,-20.2365958861061));
#25140=CARTESIAN_POINT('Ctrl Pts',(88.9699451243498,8.68728605420077,-19.3523542415107));
#25141=CARTESIAN_POINT('Ctrl Pts',(89.0095634122645,11.8196476572324,-17.614723470301));
#25142=CARTESIAN_POINT('Ctrl Pts',(89.049181700179,14.3469883408086,-15.2346390290992));
#25143=CARTESIAN_POINT('Ctrl Pts',(89.0887999880936,16.8743290243847,-12.8545545878973));
#25144=CARTESIAN_POINT('Ctrl Pts',(89.1284182760081,18.7966487885054,-9.83201647670317));
#25145=CARTESIAN_POINT('Ctrl Pts',(89.1680365639226,19.8805923059492,-6.53393835010704));
#25146=CARTESIAN_POINT('Ctrl Pts',(89.2076548518372,20.964535823393,-3.23586022351083));
#25147=CARTESIAN_POINT('Ctrl Pts',(89.2472731397519,21.2101030941599,0.337757918487176));
#25148=CARTESIAN_POINT('Ctrl Pts',(89.2868914276665,20.5874840773349,3.75310540270599));
#25149=CARTESIAN_POINT('Ctrl Pts',(89.3265097155811,19.96486506051,7.16845288692471));
#25150=CARTESIAN_POINT('Ctrl Pts',(89.3661280034956,18.4740597560931,10.425529713364));
#25151=CARTESIAN_POINT('Ctrl Pts',(89.4057462914102,16.2960408441341,13.1289509712044));
#25152=CARTESIAN_POINT('Ctrl Pts',(89.4453645793247,14.1180219321752,15.8323722290448));
#25153=CARTESIAN_POINT('Ctrl Pts',(89.4849828672394,11.252789412674,17.9821379182864));
#25154=CARTESIAN_POINT('Ctrl Pts',(89.5246011551539,8.04816121095532,19.3172824673091));
#25155=CARTESIAN_POINT('Ctrl Pts',(89.5642194430685,4.84353300923676,20.6524270163317));
#25156=CARTESIAN_POINT('Ctrl Pts',(89.6038377309831,1.29950912530069,21.1729504251357));
#25157=CARTESIAN_POINT('Ctrl Pts',(89.6434560188976,-2.15369229061819,20.8156650221266));
#25158=CARTESIAN_POINT('Ctrl Pts',(89.6830743068122,-5.60689370653718,20.4583796191175));
#25159=CARTESIAN_POINT('Ctrl Pts',(89.7226925947269,-8.96927265443904,19.2232854042953));
#25160=CARTESIAN_POINT('Ctrl Pts',(89.7623108826414,-11.8326613287715,17.2603136321663));
#25161=CARTESIAN_POINT('Ctrl Pts',(89.801929170556,-14.6960500031039,15.2973418600373));
#25162=CARTESIAN_POINT('Ctrl Pts',(89.8415474584705,-17.0604484038671,12.6064925306015));
#25163=CARTESIAN_POINT('Ctrl Pts',(89.8811657463851,-18.6388361442031,9.5144147472828));
#25164=CARTESIAN_POINT('Ctrl Pts',(89.9187248818728,-20.1351875039382,6.58304707555306));
#25165=CARTESIAN_POINT('Ctrl Pts',(89.9562840173605,-20.9251103774838,3.29107461363035));
#25166=CARTESIAN_POINT('Ctrl Pts',(89.9938431528482,-20.9266482192657,-0.000185637335865005));
#25167=CARTESIAN_POINT('Origin',(80.4,0.,0.));
#25168=CARTESIAN_POINT('',(91.7061568471519,-20.9232794228044,4.20060754047213E-5));
#25169=CARTESIAN_POINT('',(91.4938431528482,-20.9233577741311,-0.000216749186123405));
#25170=CARTESIAN_POINT('',(80.4,-20.925,-2.56257342721584E-15));
#25171=CARTESIAN_POINT('Ctrl Pts',(91.7061568471519,-20.9232794228044,4.20060754047213E-5));
#25172=CARTESIAN_POINT('Ctrl Pts',(91.6852497010242,-20.9229908458237,1.83290267080309));
#25173=CARTESIAN_POINT('Ctrl Pts',(91.6643425548965,-20.6844852225557,3.66579445525847));
#25174=CARTESIAN_POINT('Ctrl Pts',(91.6434354087688,-20.2086692594407,5.43492192001744));
#25175=CARTESIAN_POINT('Ctrl Pts',(91.6038171208542,-19.307015169212,8.78735466374625));
#25176=CARTESIAN_POINT('Ctrl Pts',(91.5641988329397,-17.5532061518,11.9108168567498));
#25177=CARTESIAN_POINT('Ctrl Pts',(91.5245805450251,-15.1600597681339,14.4258209515636));
#25178=CARTESIAN_POINT('Ctrl Pts',(91.4849622571105,-12.7669133844678,16.9408250463774));
#25179=CARTESIAN_POINT('Ctrl Pts',(91.4453439691959,-9.73442963454778,18.8473710430013));
#25180=CARTESIAN_POINT('Ctrl Pts',(91.4057256812813,-6.43077111619045,19.9141816026769));
#25181=CARTESIAN_POINT('Ctrl Pts',(91.3661073933667,-3.12711259783322,20.9809921623526));
#25182=CARTESIAN_POINT('Ctrl Pts',(91.3264891054521,0.447720688961312,21.2080672850801));
#25183=CARTESIAN_POINT('Ctrl Pts',(91.2868708175375,3.85979173246923,20.5677588081614));
#25184=CARTESIAN_POINT('Ctrl Pts',(91.247252529623,7.27186277597725,19.9274503312428));
#25185=CARTESIAN_POINT('Ctrl Pts',(91.2076342417084,10.5211715761986,18.4197582546779));
#25186=CARTESIAN_POINT('Ctrl Pts',(91.1680159537938,13.2132654327391,16.2277473692253));
#25187=CARTESIAN_POINT('Ctrl Pts',(91.1283976658792,15.9053592892796,14.0357364837727));
#25188=CARTESIAN_POINT('Ctrl Pts',(91.0887793779647,18.0402382021391,11.1594067894323));
#25189=CARTESIAN_POINT('Ctrl Pts',(91.0491610900501,19.3587492228123,7.94790186760101));
#25190=CARTESIAN_POINT('Ctrl Pts',(91.0095428021355,20.6772602434854,4.73639694576969));
#25191=CARTESIAN_POINT('Ctrl Pts',(90.969924514221,21.179403371972,1.18971679644736));
#25192=CARTESIAN_POINT('Ctrl Pts',(90.9303062263064,20.8042193785163,-2.26158706287777));
#25193=CARTESIAN_POINT('Ctrl Pts',(90.8906879383918,20.4290353850607,-5.71289092220279));
#25194=CARTESIAN_POINT('Ctrl Pts',(90.8510696504772,19.1765242696626,-9.06881849153062));
#25195=CARTESIAN_POINT('Ctrl Pts',(90.8114513625626,17.1987329874818,-11.9219906681495));
#25196=CARTESIAN_POINT('Ctrl Pts',(90.7718330746481,15.220941705301,-14.7751628447684));
#25197=CARTESIAN_POINT('Ctrl Pts',(90.7322147867335,12.5178702563374,-17.1255796286783));
#25198=CARTESIAN_POINT('Ctrl Pts',(90.692596498819,9.41765069622895,-18.6879150721364));
#25199=CARTESIAN_POINT('Ctrl Pts',(90.6529782109044,6.31743113612043,-20.2502505155946));
#25200=CARTESIAN_POINT('Ctrl Pts',(90.6133599229898,2.82006346486707,-21.024504618601));
#25201=CARTESIAN_POINT('Ctrl Pts',(90.5737416350752,-0.649897517646015,
-20.9166901267311));
#25202=CARTESIAN_POINT('Ctrl Pts',(90.5341233471605,-4.11985850015881,-20.8088756348612));
#25203=CARTESIAN_POINT('Ctrl Pts',(90.494505059246,-7.56241279393134,-19.8189925481151));
#25204=CARTESIAN_POINT('Ctrl Pts',(90.4548867713314,-10.5596600892345,-18.0672045824493));
#25205=CARTESIAN_POINT('Ctrl Pts',(90.4152684834168,-13.5569073845378,-16.3154166167835));
#25206=CARTESIAN_POINT('Ctrl Pts',(90.3756501955023,-16.1088476813718,-13.8017237721979));
#25207=CARTESIAN_POINT('Ctrl Pts',(90.3360319075877,-17.9056943060018,-10.8312700430694));
#25208=CARTESIAN_POINT('Ctrl Pts',(90.2964136196731,-19.7025409306319,-7.86081631394061));
#25209=CARTESIAN_POINT('Ctrl Pts',(90.2567953317585,-20.7442938830579,-4.43360170026879));
#25210=CARTESIAN_POINT('Ctrl Pts',(90.217177043844,-20.9044921484388,-0.965664386132399));
#25211=CARTESIAN_POINT('Ctrl Pts',(90.2135036449466,-20.9193456961912,-0.644118004993295));
#25212=CARTESIAN_POINT('Ctrl Pts',(90.2098302460492,-20.9266205558477,-0.322221532532826));
#25213=CARTESIAN_POINT('Ctrl Pts',(90.2061568471519,-20.9263865279884,-0.000314477239331534));
#25214=CARTESIAN_POINT('Ctrl Pts',(89.9938431528482,-20.9266482192657,-0.000185637335865005));
#25215=CARTESIAN_POINT('Ctrl Pts',(89.9959023052751,-20.9267325303287,-0.180626599178571));
#25216=CARTESIAN_POINT('Ctrl Pts',(89.997961457702,-20.9244471914867,-0.361065420327887));
#25217=CARTESIAN_POINT('Ctrl Pts',(90.0000206101289,-20.9197786974978,-0.541442561017874));
#25218=CARTESIAN_POINT('Ctrl Pts',(90.0396388980435,-20.8299564305474,-4.01191584879784));
#25219=CARTESIAN_POINT('Ctrl Pts',(90.079257185958,-19.8579348167377,-7.45955618715585));
#25220=CARTESIAN_POINT('Ctrl Pts',(90.1188754738726,-18.121710053413,-10.4658456683132));
#25221=CARTESIAN_POINT('Ctrl Pts',(90.1584937617872,-16.3854852900884,-13.4721351494706));
#25222=CARTESIAN_POINT('Ctrl Pts',(90.1981120497018,-13.8850573772488,-16.0370737734273));
#25223=CARTESIAN_POINT('Ctrl Pts',(90.2377303376164,-10.9239596727245,-17.8492970677619));
#25224=CARTESIAN_POINT('Ctrl Pts',(90.2773486255309,-7.96286196820022,-19.6615203620964));
#25225=CARTESIAN_POINT('Ctrl Pts',(90.3169669134455,-4.54109447199126,-20.7210283268088));
#25226=CARTESIAN_POINT('Ctrl Pts',(90.3565852013601,-1.07403431882255,-20.8992045592561));
#25227=CARTESIAN_POINT('Ctrl Pts',(90.3962034892746,2.39302583434616,-21.0773807917034));
#25228=CARTESIAN_POINT('Ctrl Pts',(90.4358217771892,5.90537864447457,-20.3742252918856));
#25229=CARTESIAN_POINT('Ctrl Pts',(90.4754400651038,9.03665059614102,-18.875095935191));
#25230=CARTESIAN_POINT('Ctrl Pts',(90.5150583530184,12.1679225478073,-17.3759665784964));
#25231=CARTESIAN_POINT('Ctrl Pts',(90.554676640933,14.9181136410116,-15.0808633649252));
#25232=CARTESIAN_POINT('Ctrl Pts',(90.5942949288476,16.9533711204631,-12.2683947106227));
#25233=CARTESIAN_POINT('Ctrl Pts',(90.6339132167621,18.9886285999148,-9.45592605631999));
#25234=CARTESIAN_POINT('Ctrl Pts',(90.6735315046767,20.3089524656136,-6.12609196128567));
#25235=CARTESIAN_POINT('Ctrl Pts',(90.7131497925913,20.7540652241585,-2.68310962666201));
#25236=CARTESIAN_POINT('Ctrl Pts',(90.7527680805059,21.1991779827034,0.75987270796175));
#25237=CARTESIAN_POINT('Ctrl Pts',(90.7923863684204,20.7690796340944,4.31600328217511));
#25238=CARTESIAN_POINT('Ctrl Pts',(90.832004656335,19.5159809054035,7.55359447776977));
#25239=CARTESIAN_POINT('Ctrl Pts',(90.8716229442496,18.2628821767127,10.7911856733641));
#25240=CARTESIAN_POINT('Ctrl Pts',(90.9112412321641,16.1867830679401,13.7102374903398));
#25241=CARTESIAN_POINT('Ctrl Pts',(90.9508595200787,13.5397066043922,15.956398358946));
#25242=CARTESIAN_POINT('Ctrl Pts',(90.9904778079933,10.8926301408442,18.2025592275522));
#25243=CARTESIAN_POINT('Ctrl Pts',(91.0300960959079,7.67457632252076,19.7758291477888));
#25244=CARTESIAN_POINT('Ctrl Pts',(91.0697143838225,4.27619290028805,20.4852255990882));
#25245=CARTESIAN_POINT('Ctrl Pts',(91.1093326717371,0.877809478055243,21.1946220503876));
#25246=CARTESIAN_POINT('Ctrl Pts',(91.1489509596516,-2.70090354808683,21.0401450327498));
#25247=CARTESIAN_POINT('Ctrl Pts',(91.1885692475662,-6.02551691195499,20.0405454316577));
#25248=CARTESIAN_POINT('Ctrl Pts',(91.2281875354808,-9.35013027582305,19.0409458305656));
#25249=CARTESIAN_POINT('Ctrl Pts',(91.2678058233954,-12.4206439774172,17.1962236460193));
#25250=CARTESIAN_POINT('Ctrl Pts',(91.30742411131,-14.8643207022932,14.7303173377137));
#25251=CARTESIAN_POINT('Ctrl Pts',(91.3470423992245,-17.3079974271691,12.2644110294083));
#25252=CARTESIAN_POINT('Ctrl Pts',(91.3866606871391,-19.1248371753269,9.17732059734364));
#25253=CARTESIAN_POINT('Ctrl Pts',(91.4262789750536,-20.0942886764528,5.84379016318228));
#25254=CARTESIAN_POINT('Ctrl Pts',(91.4488003676518,-20.6453826032978,3.94881308069201));
#25255=CARTESIAN_POINT('Ctrl Pts',(91.47132176025,-20.9226462243581,1.97419984397363));
#25256=CARTESIAN_POINT('Ctrl Pts',(91.4938431528482,-20.9233577741311,-0.000216749186123405));
#25257=CARTESIAN_POINT('Origin',(65.9521295958992,0.,0.));
#25258=CARTESIAN_POINT('',(90.7021295958993,-20.0672796057963,-0.000301566765486798));
#25259=CARTESIAN_POINT('',(90.9978704041008,-20.0643751936834,-0.000207850816367205));
#25260=CARTESIAN_POINT('',(65.9521295958992,-20.06595,-1.45722292471193E-12));
#25261=CARTESIAN_POINT('',(92.,-13.2931882197129,15.0310843373919));
#25262=CARTESIAN_POINT('Ctrl Pts',(90.7021295958993,-20.0672796057963,-0.000301566765486157));
#25263=CARTESIAN_POINT('Ctrl Pts',(90.7058029947966,-20.0675040259313,-0.308993125960923));
#25264=CARTESIAN_POINT('Ctrl Pts',(90.7490946816086,-19.9852882243807,-3.94686076179615));
#25265=CARTESIAN_POINT('Ctrl Pts',(90.8320046563349,-17.8946924029286,-10.8246147761969));
#25266=CARTESIAN_POINT('Ctrl Pts',(90.9508595200788,-10.5531717722109,-18.05610365574));
#25267=CARTESIAN_POINT('Ctrl Pts',(91.0697143838226,-0.649498319719339,
-20.9038376377461));
#25268=CARTESIAN_POINT('Ctrl Pts',(91.1885692475662,9.41186437891623,-18.6764334630907));
#25269=CARTESIAN_POINT('Ctrl Pts',(91.30742411131,17.1881649583186,-11.9146634752632));
#25270=CARTESIAN_POINT('Ctrl Pts',(91.4262789750537,20.7914374193968,-2.26020113694711));
#25271=CARTESIAN_POINT('Ctrl Pts',(91.5451338387974,19.3468526295679,7.94302560746775));
#25272=CARTESIAN_POINT('Ctrl Pts',(91.6639887025412,13.2051503325794,16.2177622139406));
#25273=CARTESIAN_POINT('Ctrl Pts',(91.7828435662849,3.85741299640702,20.5551491420764));
#25274=CARTESIAN_POINT('Ctrl Pts',(91.8948473321045,-5.83399714535016,19.9395461276724));
#25275=CARTESIAN_POINT('Ctrl Pts',(91.9672328100095,-11.2292638125539,16.8535785943549));
#25276=CARTESIAN_POINT('Ctrl Pts',(92.,-13.2939520371393,15.0312716283105));
#25277=CARTESIAN_POINT('',(92.,9.87756200380559,17.4664283201654));
#25278=CARTESIAN_POINT('Origin',(92.,0.,0.));
#25279=CARTESIAN_POINT('Ctrl Pts',(90.9978704041008,-20.0643751936834,-0.000207850816367205));
#25280=CARTESIAN_POINT('Ctrl Pts',(91.0149672994172,-20.064893183897,-1.4375331253234));
#25281=CARTESIAN_POINT('Ctrl Pts',(91.0716824826482,-19.5596239647444,-6.20518254004424));
#25282=CARTESIAN_POINT('Ctrl Pts',(91.1680159537938,-15.8234056085072,-13.6752200512566));
#25283=CARTESIAN_POINT('Ctrl Pts',(91.2868708175377,-7.37201867707368,-19.5715898806077));
#25284=CARTESIAN_POINT('Ctrl Pts',(91.4057256812812,2.86917222790772,-20.7161033751214));
#25285=CARTESIAN_POINT('Ctrl Pts',(91.5245805450251,12.4137954244847,-16.8313801312361));
#25286=CARTESIAN_POINT('Ctrl Pts',(91.6434354087687,18.9444853649975,-8.85960809395612));
#25287=CARTESIAN_POINT('Ctrl Pts',(91.7622902725126,20.8758294198323,1.26187795552705));
#25288=CARTESIAN_POINT('Ctrl Pts',(91.8811451362562,17.7386656817295,11.0795895560304));
#25289=CARTESIAN_POINT('Ctrl Pts',(91.9603817120854,12.7761628790883,15.8272202722995));
#25290=CARTESIAN_POINT('Ctrl Pts',(92.,9.87756200380534,17.4664283201656));
#25291=CARTESIAN_POINT('Origin',(65.9521295958992,0.,0.));
#25292=CARTESIAN_POINT('',(89.2021295958992,-20.0653836777985,0.000495366012167058));
#25293=CARTESIAN_POINT('',(89.4978704041008,-20.0675305536619,-0.00017801622778868));
#25294=CARTESIAN_POINT('',(65.9521295958992,-20.06595,-1.45722292471193E-12));
#25295=CARTESIAN_POINT('Ctrl Pts',(89.2021295958992,-20.0653836777985,0.000495366012166348));
#25296=CARTESIAN_POINT('Ctrl Pts',(89.2303835398216,-20.0631674353115,-2.37445247022255));
#25297=CARTESIAN_POINT('Ctrl Pts',(89.2982557716587,-19.0499289088233,-8.08144412695439));
#25298=CARTESIAN_POINT('Ctrl Pts',(89.4057462914101,-13.7570952656821,-15.7522897774154));
#25299=CARTESIAN_POINT('Ctrl Pts',(89.524601155154,-4.56466310983042,-20.4097073491906));
#25300=CARTESIAN_POINT('Ctrl Pts',(89.6434560188976,5.73600137388006,-20.1119514620605));
#25301=CARTESIAN_POINT('Ctrl Pts',(89.7623108826413,14.6440500167558,-14.9313128191482));
#25302=CARTESIAN_POINT('Ctrl Pts',(89.8811657463853,19.996741067543,-6.12557344600731));
#25303=CARTESIAN_POINT('Ctrl Pts',(90.0000206101288,20.4945207331834,4.16736407124383));
#25304=CARTESIAN_POINT('Ctrl Pts',(90.1188754738726,16.0165355102348,13.4485275657482));
#25305=CARTESIAN_POINT('Ctrl Pts',(90.2377303376165,7.64997362942123,19.4645885301395));
#25306=CARTESIAN_POINT('Ctrl Pts',(90.3565852013599,-2.57388810220134,20.7549368562865));
#25307=CARTESIAN_POINT('Ctrl Pts',(90.475440065104,-12.172848063172,17.0062950847534));
#25308=CARTESIAN_POINT('Ctrl Pts',(90.59062152995,-18.6110913235361,9.37224505906302));
#25309=CARTESIAN_POINT('Ctrl Pts',(90.666184706882,-20.0650836131825,3.02030255107542));
#25310=CARTESIAN_POINT('Ctrl Pts',(90.7021295958993,-20.0672796057963,-0.000301566765486157));
#25311=CARTESIAN_POINT('Ctrl Pts',(89.4978704041008,-20.0675305536619,-0.000178016227787951));
#25312=CARTESIAN_POINT('Ctrl Pts',(89.4999295565277,-20.0676114034384,-0.173211197506917));
#25313=CARTESIAN_POINT('Ctrl Pts',(89.5416069968692,-20.0232548899331,-3.67537764220059));
#25314=CARTESIAN_POINT('Ctrl Pts',(89.6229027251253,-18.1105753899303,-10.4594150595525));
#25315=CARTESIAN_POINT('Ctrl Pts',(89.7417575888689,-10.9172475795155,-17.8383297808979));
#25316=CARTESIAN_POINT('Ctrl Pts',(89.8606124526128,-1.07337439090547,-20.886363306994));
#25317=CARTESIAN_POINT('Ctrl Pts',(89.9794673163564,9.03109813531615,-18.8634983461956));
#25318=CARTESIAN_POINT('Ctrl Pts',(90.0983221801003,16.9429543312567,-12.2608565786884));
#25319=CARTESIAN_POINT('Ctrl Pts',(90.2171770438438,20.7413131374097,-2.68146095729082));
#25320=CARTESIAN_POINT('Ctrl Pts',(90.3360319075878,19.5039895591631,7.5489531352732));
#25321=CARTESIAN_POINT('Ctrl Pts',(90.4548867713314,13.531387277919,15.9465943979035));
#25322=CARTESIAN_POINT('Ctrl Pts',(90.5737416350752,4.2735654835411,20.4726382052112));
#25323=CARTESIAN_POINT('Ctrl Pts',(90.6925964988188,-6.021814680891,20.0282327411152));
#25324=CARTESIAN_POINT('Ctrl Pts',(90.8114513625627,-14.8551873562319,14.7212645520118));
#25325=CARTESIAN_POINT('Ctrl Pts',(90.9132093309899,-19.330090149826,7.11771580065352));
#25326=CARTESIAN_POINT('Ctrl Pts',(90.9753490115026,-20.0636928557065,1.89315151059409));
#25327=CARTESIAN_POINT('Ctrl Pts',(90.9978704041008,-20.0643751936834,-0.000207850816367205));
#25328=CARTESIAN_POINT('Origin',(65.9521295958992,0.,0.));
#25329=CARTESIAN_POINT('',(87.7021295958992,-20.0649676983134,-0.000434282711544843));
#25330=CARTESIAN_POINT('',(87.9978704041009,-20.0650171626467,0.000444174233464878));
#25331=CARTESIAN_POINT('',(65.9521295958992,-20.06595,-1.45722292471193E-12));
#25332=CARTESIAN_POINT('Ctrl Pts',(87.7021295958992,-20.0649676983134,-0.000434282711544581));
#25333=CARTESIAN_POINT('Ctrl Pts',(87.7153457969321,-20.065848378389,-1.11141741996506));
#25334=CARTESIAN_POINT('Ctrl Pts',(87.7681802858796,-19.7031926272816,-5.55223264921002));
#25335=CARTESIAN_POINT('Ctrl Pts',(87.8606330627416,-16.4712183986482,-12.887640119355));
#25336=CARTESIAN_POINT('Ctrl Pts',(87.9794879264853,-8.3173102399601,-19.1889200778529));
#25337=CARTESIAN_POINT('Ctrl Pts',(88.0983427902292,1.85591716921299,-20.8314155746315));
#25338=CARTESIAN_POINT('Ctrl Pts',(88.2171976539728,11.5785554866035,-17.4163531264618));
#25339=CARTESIAN_POINT('Ctrl Pts',(88.3360525177166,18.4900927013111,-9.77285911485978));
#25340=CARTESIAN_POINT('Ctrl Pts',(88.4549073814602,20.9125103499811,0.243339770501251));
#25341=CARTESIAN_POINT('Ctrl Pts',(88.5737622452041,18.2576814481021,10.2004593779692));
#25342=CARTESIAN_POINT('Ctrl Pts',(88.6926171089477,11.170158976582,17.6810591260786));
#25343=CARTESIAN_POINT('Ctrl Pts',(88.8114719726915,1.37068800228615,20.868960630139));
#25344=CARTESIAN_POINT('Ctrl Pts',(88.9303268364353,-8.76156563726881,18.9901888080648));
#25345=CARTESIAN_POINT('Ctrl Pts',(89.049181700179,-16.766641421806,12.5008815214899));
#25346=CARTESIAN_POINT('Ctrl Pts',(89.1397826200003,-19.7657518411832,5.24065233111284));
#25347=CARTESIAN_POINT('Ctrl Pts',(89.190765251907,-20.0662750981985,0.955750471229892));
#25348=CARTESIAN_POINT('Ctrl Pts',(89.2021295958992,-20.0653836777985,0.000495366012166348));
#25349=CARTESIAN_POINT('Ctrl Pts',(87.9978704041009,-20.0650171626467,0.000444174233465294));
#25350=CARTESIAN_POINT('Ctrl Pts',(88.0245101015528,-20.0631950929372,-2.23893198812163));
#25351=CARTESIAN_POINT('Ctrl Pts',(88.0907680869193,-19.1327997546737,-7.8101620247403));
#25352=CARTESIAN_POINT('Ctrl Pts',(88.1966443602004,-14.0737816631622,-15.4700023912384));
#25353=CARTESIAN_POINT('Ctrl Pts',(88.3154992239441,-4.97771098870528,-20.312919475056));
#25354=CARTESIAN_POINT('Ctrl Pts',(88.4343540876879,5.32687389681903,-20.2241617570368));
#25355=CARTESIAN_POINT('Ctrl Pts',(88.5532089514316,14.3381730091277,-15.2252782912942));
#25356=CARTESIAN_POINT('Ctrl Pts',(88.6720638151754,19.868376918928,-6.52992365153576));
#25357=CARTESIAN_POINT('Ctrl Pts',(88.790918678919,20.5748343493,3.75079935297009));
#25358=CARTESIAN_POINT('Ctrl Pts',(88.9097735426629,16.2860279409612,13.1208840476639));
#25359=CARTESIAN_POINT('Ctrl Pts',(89.0286284064065,8.04321611663378,19.3054131992102));
#25360=CARTESIAN_POINT('Ctrl Pts',(89.1474832701505,-2.15236898069497,20.8028750909506));
#25361=CARTESIAN_POINT('Ctrl Pts',(89.2663381338938,-11.8253908946233,17.2497082436515));
#25362=CARTESIAN_POINT('Ctrl Pts',(89.383133845211,-18.5095396758491,9.64268344613609));
#25363=CARTESIAN_POINT('Ctrl Pts',(89.4603112686131,-20.0660558460732,3.15596361497391));
#25364=CARTESIAN_POINT('Ctrl Pts',(89.4978704041008,-20.0675305536619,-0.000178016227787951));
#25365=CARTESIAN_POINT('Origin',(65.9521295958992,0.,0.));
#25366=CARTESIAN_POINT('',(86.2021295958992,-20.0675576587757,0.000158315979958626));
#25367=CARTESIAN_POINT('',(86.4978704041008,-20.0653267550518,-0.000489666735370431));
#25368=CARTESIAN_POINT('',(65.9521295958992,-20.06595,-1.45722292471193E-12));
#25369=CARTESIAN_POINT('Ctrl Pts',(86.2021295958992,-20.0675576587757,0.000158315979958117));
#25370=CARTESIAN_POINT('Ctrl Pts',(86.2399263419571,-20.0662194103506,-3.17593753999125));
#25371=CARTESIAN_POINT('Ctrl Pts',(86.3173413759297,-18.4943095347506,-9.68247290148306));
#25372=CARTESIAN_POINT('Ctrl Pts',(86.4343746978168,-11.7738322969147,-17.28494074118));
#25373=CARTESIAN_POINT('Ctrl Pts',(86.5532295615605,-2.09024411951815,-20.8092090888336));
#25374=CARTESIAN_POINT('Ctrl Pts',(86.6720844253043,8.10082424882741,-19.2813108960876));
#25375=CARTESIAN_POINT('Ctrl Pts',(86.7909392890479,16.3251329462566,-13.0721971247768));
#25376=CARTESIAN_POINT('Ctrl Pts',(86.9097941527918,20.5859421139072,-3.68934827101431));
#25377=CARTESIAN_POINT('Ctrl Pts',(87.0286490165353,19.8487906427609,6.58921948350647));
#25378=CARTESIAN_POINT('Ctrl Pts',(87.1475038802793,14.2926479488024,15.2680227270453));
#25379=CARTESIAN_POINT('Ctrl Pts',(87.2663587440228,5.26646286003707,20.2399770831349));
#25380=CARTESIAN_POINT('Ctrl Pts',(87.3852136077667,-5.03834110050527,20.2979659655083));
#25381=CARTESIAN_POINT('Ctrl Pts',(87.5040684715104,-14.1199107603864,15.4279105358017));
#25382=CARTESIAN_POINT('Ctrl Pts',(87.6097071342212,-19.144732578109,7.77022286859828));
#25383=CARTESIAN_POINT('Ctrl Pts',(87.6757275090175,-20.063208358257,2.21898363026297));
#25384=CARTESIAN_POINT('Ctrl Pts',(87.7021295958992,-20.0649676983134,-0.000434282711544581));
#25385=CARTESIAN_POINT('Ctrl Pts',(86.4978704041008,-20.0653267550518,-0.000489666735369598));
#25386=CARTESIAN_POINT('Ctrl Pts',(86.5094723586633,-20.0662222709964,-0.975725602202006));
#25387=CARTESIAN_POINT('Ctrl Pts',(86.5606926011403,-19.7579380015879,-5.28063034010222));
#25388=CARTESIAN_POINT('Ctrl Pts',(86.6515311315318,-16.7292403389556,-12.5508892899555));
#25389=CARTESIAN_POINT('Ctrl Pts',(86.7703859952756,-8.70482382118687,-19.0162653149707));
#25390=CARTESIAN_POINT('Ctrl Pts',(86.8892408590193,1.432994482384,-20.8647748873721));
#25391=CARTESIAN_POINT('Ctrl Pts',(87.0080957227631,11.2229030338076,-17.6476273697347));
#25392=CARTESIAN_POINT('Ctrl Pts',(87.1269505865067,18.2880576096475,-10.1458983413729));
#25393=CARTESIAN_POINT('Ctrl Pts',(87.2458054502506,20.9131437355076,-0.180896062030789));
#25394=CARTESIAN_POINT('Ctrl Pts',(87.3646603139942,18.460829534231,9.82802509130509));
#25395=CARTESIAN_POINT('Ctrl Pts',(87.4835151777381,11.5265004287498,17.4508478921023));
#25396=CARTESIAN_POINT('Ctrl Pts',(87.6023700414816,1.79370841459017,20.8368643132955));
#25397=CARTESIAN_POINT('Ctrl Pts',(87.7212249052256,-8.37456933075415,19.1639999168141));
#25398=CARTESIAN_POINT('Ctrl Pts',(87.8400797689691,-16.5096261697931,12.8384013031585));
#25399=CARTESIAN_POINT('Ctrl Pts',(87.932294935261,-19.7114331280202,5.51225344509298));
#25400=CARTESIAN_POINT('Ctrl Pts',(87.9848918136382,-20.0659048565327,1.09144553246543));
#25401=CARTESIAN_POINT('Ctrl Pts',(87.9978704041009,-20.0650171626467,0.000444174233465294));
#25402=CARTESIAN_POINT('Origin',(65.9521295958992,0.,0.));
#25403=CARTESIAN_POINT('',(84.7021295958992,-20.0643985029825,0.000222280623257588));
#25404=CARTESIAN_POINT('',(84.9978704041008,-20.0673230876221,0.00028466991946835));
#25405=CARTESIAN_POINT('',(65.9521295958992,-20.06595,-1.45722292471193E-12));
#25406=CARTESIAN_POINT('Ctrl Pts',(84.7021295958992,-20.0643985029825,0.000222280623257826));
#25407=CARTESIAN_POINT('Ctrl Pts',(84.7248885990676,-20.0636511338426,-1.91310542372513));
#25408=CARTESIAN_POINT('Ctrl Pts',(84.7872658901506,-19.3192530083258,-7.1576742664364));
#25409=CARTESIAN_POINT('Ctrl Pts',(84.8892614691482,-14.8111651148504,-14.7655576028342));
#25410=CARTESIAN_POINT('Ctrl Pts',(85.0081163328919,-5.96198547260468,-20.0461226327294));
#25411=CARTESIAN_POINT('Ctrl Pts',(85.1269711966356,4.33467558954779,-20.4597871669124));
#25412=CARTESIAN_POINT('Ctrl Pts',(85.2458260603795,13.5789418738155,-15.9061196075446));
#25413=CARTESIAN_POINT('Ctrl Pts',(85.364680924123,19.5264429856993,-7.49068272644153));
#25414=CARTESIAN_POINT('Ctrl Pts',(85.483535787867,20.7332140926975,2.74338053655433));
#25415=CARTESIAN_POINT('Ctrl Pts',(85.6023906516105,16.9062691143363,12.3113917984773));
#25416=CARTESIAN_POINT('Ctrl Pts',(85.7212455153543,8.97473338589818,18.890380198239));
#25417=CARTESIAN_POINT('Ctrl Pts',(85.8401003790982,-1.13573415718418,20.8830651798576));
#25418=CARTESIAN_POINT('Ctrl Pts',(85.9589552428418,-10.9704623349105,17.8056524603926));
#25419=CARTESIAN_POINT('Ctrl Pts',(86.0778101065857,-18.1417253850317,10.4052920879747));
#25420=CARTESIAN_POINT('Ctrl Pts',(86.1588682242713,-20.0286087768165,3.63541879634039));
#25421=CARTESIAN_POINT('Ctrl Pts',(86.2003080540426,-20.0676221530979,0.153224178672827));
#25422=CARTESIAN_POINT('Ctrl Pts',(86.2021295958992,-20.0675576587757,0.000158315979958117));
#25423=CARTESIAN_POINT('Ctrl Pts',(84.9978704041008,-20.0673230876221,0.000284669919469217));
#25424=CARTESIAN_POINT('Ctrl Pts',(85.0340529036883,-20.0652120135904,-3.04026780378225));
#25425=CARTESIAN_POINT('Ctrl Pts',(85.1098536911904,-18.596352367802,-9.4120653334657));
#25426=CARTESIAN_POINT('Ctrl Pts',(85.225272766607,-12.122014753868,-17.0425661974441));
#25427=CARTESIAN_POINT('Ctrl Pts',(85.3441276303508,-2.51190450252216,-20.7625297123801));
#25428=CARTESIAN_POINT('Ctrl Pts',(85.4629824940945,7.70805881080918,-19.4416597454118));
#25429=CARTESIAN_POINT('Ctrl Pts',(85.5818373578382,16.0566200612769,-13.4006438835997));
#25430=CARTESIAN_POINT('Ctrl Pts',(85.700692221582,20.5068727177375,-4.10615095019311));
#25431=CARTESIAN_POINT('Ctrl Pts',(85.8195470853257,19.9783616090541,6.18525437675218));
#25432=CARTESIAN_POINT('Ctrl Pts',(85.9384019490693,14.5994013736218,14.9749719138016));
#25433=CARTESIAN_POINT('Ctrl Pts',(86.0572568128132,5.67592357316316,20.1289889432845));
#25434=CARTESIAN_POINT('Ctrl Pts',(86.1761116765568,-4.62558407166802,20.3959867690482));
#25435=CARTESIAN_POINT('Ctrl Pts',(86.2949665403008,-13.8040686848729,15.7111422891708));
#25436=CARTESIAN_POINT('Ctrl Pts',(86.4022194494818,-19.0623251133496,8.04151842586029));
#25437=CARTESIAN_POINT('Ctrl Pts',(86.4698540707486,-20.0631642682839,2.35450447826081));
#25438=CARTESIAN_POINT('Ctrl Pts',(86.4978704041008,-20.0653267550518,-0.000489666735369598));
#25439=CARTESIAN_POINT('Origin',(65.9521295958992,0.,0.));
#25440=CARTESIAN_POINT('',(83.2021295958992,-20.0663262756018,-0.000495292805329403));
#25441=CARTESIAN_POINT('',(83.4978704041008,-20.0642786305281,0.000103247315883515));
#25442=CARTESIAN_POINT('',(65.9521295958992,-20.06595,-1.45722292471193E-12));
#25443=CARTESIAN_POINT('Ctrl Pts',(83.2021295958992,-20.0663262756018,-0.000495292805329922));
#25444=CARTESIAN_POINT('Ctrl Pts',(83.2098508561781,-20.0669889354332,-0.649435220771842));
#25445=CARTESIAN_POINT('Ctrl Pts',(83.2571904043715,-19.8777692591846,-4.62774326658148));
#25446=CARTESIAN_POINT('Ctrl Pts',(83.3441482404796,-17.3211691177578,-11.7204694349677));
#25447=CARTESIAN_POINT('Ctrl Pts',(83.4630031042234,-9.62145947804478,-18.5693247290879));
#25448=CARTESIAN_POINT('Ctrl Pts',(83.581857967967,0.41419745487271,-20.9098240989816));
#25449=CARTESIAN_POINT('Ctrl Pts',(83.7007128317109,10.3492934047325,-18.1737291001251));
#25450=CARTESIAN_POINT('Ctrl Pts',(83.8195676954545,17.7717348066487,-11.025322913372));
#25451=CARTESIAN_POINT('Ctrl Pts',(83.9384225591984,20.8794632575961,-1.20013226632287));
#25452=CARTESIAN_POINT('Ctrl Pts',(84.057277422942,18.9179685006256,8.91643264940149));
#25453=CARTESIAN_POINT('Ctrl Pts',(84.1761322866858,12.3634722959219,16.8682203023895));
#25454=CARTESIAN_POINT('Ctrl Pts',(84.2949871504295,2.80730885869799,20.7246548910676));
#25455=CARTESIAN_POINT('Ctrl Pts',(84.4138420141732,-7.43042742562143,19.5494514412693));
#25456=CARTESIAN_POINT('Ctrl Pts',(84.532696877917,-15.8641664191098,13.6279318757016));
#25457=CARTESIAN_POINT('Ctrl Pts',(84.6287927384923,-19.5689046288147,6.16520005828642));
#25458=CARTESIAN_POINT('Ctrl Pts',(84.685270311153,-20.0649521348374,1.41756628034156));
#25459=CARTESIAN_POINT('Ctrl Pts',(84.7021295958992,-20.0643985029825,0.000222280623257826));
#25460=CARTESIAN_POINT('Ctrl Pts',(83.4978704041008,-20.0642786305281,0.000103247315884208));
#25461=CARTESIAN_POINT('Ctrl Pts',(83.5190151607988,-20.0639584731567,-1.77754669223435));
#25462=CARTESIAN_POINT('Ctrl Pts',(83.5797782054113,-19.3915725094379,-6.88616286129953));
#25463=CARTESIAN_POINT('Ctrl Pts',(83.6801595379384,-15.1076199452285,-14.4620926520955));
#25464=CARTESIAN_POINT('Ctrl Pts',(83.7990144016822,-6.36737098063297,-19.9210665146787));
#25465=CARTESIAN_POINT('Ctrl Pts',(83.9178692654259,3.91878097726412,-20.5435016474673));
#25466=CARTESIAN_POINT('Ctrl Pts',(84.0367241291697,13.2535111849172,-16.1782800556342));
#25467=CARTESIAN_POINT('Ctrl Pts',(84.1555789929134,19.3704859523993,-7.88521263220971));
#25468=CARTESIAN_POINT('Ctrl Pts',(84.2744338566571,20.7845947636492,2.32226716769303));
#25469=CARTESIAN_POINT('Ctrl Pts',(84.3932887204008,17.152513026647,11.9659350306595));
#25470=CARTESIAN_POINT('Ctrl Pts',(84.5121435841446,9.3560561792281,18.7044517978578));
#25471=CARTESIAN_POINT('Ctrl Pts',(84.6309984478883,-0.711911986905901,
20.901805797829));
#25472=CARTESIAN_POINT('Ctrl Pts',(84.7498533116321,-10.6070385085257,18.0245121533403));
#25473=CARTESIAN_POINT('Ctrl Pts',(84.8687081753758,-17.9269338035892,10.7711349768254));
#25474=CARTESIAN_POINT('Ctrl Pts',(84.951380539532,-19.9910515517318,3.90689779358534));
#25475=CARTESIAN_POINT('Ctrl Pts',(84.9944346157737,-20.0675235492706,0.289006975347951));
#25476=CARTESIAN_POINT('Ctrl Pts',(84.9978704041008,-20.0673230876221,0.000284669919469217));
#25477=CARTESIAN_POINT('Origin',(65.9521295958992,0.,0.));
#25478=CARTESIAN_POINT('',(81.7021295958993,-20.0664325672107,0.000484799890657325));
#25479=CARTESIAN_POINT('',(81.9978704041008,-20.0667413636039,-0.000441116259225494));
#25480=CARTESIAN_POINT('',(65.9521295958992,-20.06595,-1.45722292471193E-12));
#25481=CARTESIAN_POINT('Ctrl Pts',(81.7021295958993,-20.0664325672107,0.000484799890658819));
#25482=CARTESIAN_POINT('Ctrl Pts',(81.7344314012032,-20.0636845251475,-2.71430660379001));
#25483=CARTESIAN_POINT('Ctrl Pts',(81.8063514944216,-18.8281343099021,-8.76122511579918));
#25484=CARTESIAN_POINT('Ctrl Pts',(81.9178898755548,-12.9383761771515,-16.4313945020042));
#25485=CARTESIAN_POINT('Ctrl Pts',(82.0367447392985,-3.52102754484433,-20.6153988176417));
#25486=CARTESIAN_POINT('Ctrl Pts',(82.1555996030423,6.75117421878302,-19.7942908448273));
#25487=CARTESIAN_POINT('Ctrl Pts',(82.274454466786,15.3842912699189,-14.1674233897442));
#25488=CARTESIAN_POINT('Ctrl Pts',(82.3933093305298,20.2823311602726,-5.10091620074396));
#25489=CARTESIAN_POINT('Ctrl Pts',(82.5121641942734,20.2561226367727,5.20401759278348));
#25490=CARTESIAN_POINT('Ctrl Pts',(82.6310190580173,15.3120287392127,14.2454932968817));
#25491=CARTESIAN_POINT('Ctrl Pts',(82.7498739217609,6.65040194880476,19.8283750544846));
#25492=CARTESIAN_POINT('Ctrl Pts',(82.8687287855047,-3.62584354539574,20.5972221905355));
#25493=CARTESIAN_POINT('Ctrl Pts',(82.9875836492484,-13.0217881419229,16.3653700529151));
#25494=CARTESIAN_POINT('Ctrl Pts',(83.0987172527133,-18.8512229442922,8.69328500138972));
#25495=CARTESIAN_POINT('Ctrl Pts',(83.1702325682635,-20.0635887848047,2.68031769219749));
#25496=CARTESIAN_POINT('Ctrl Pts',(83.2021295958992,-20.0663262756018,-0.000495292805329922));
#25497=CARTESIAN_POINT('Ctrl Pts',(81.9978704041008,-20.0667413636039,-0.000441116259225702));
#25498=CARTESIAN_POINT('Ctrl Pts',(82.0039774179092,-20.0672340924104,-0.513679681067149));
#25499=CARTESIAN_POINT('Ctrl Pts',(82.0497027196323,-19.9227688913182,-4.35619568812115));
#25500=CARTESIAN_POINT('Ctrl Pts',(82.1350463092699,-17.5553415020576,-11.3667184813117));
#25501=CARTESIAN_POINT('Ctrl Pts',(82.2539011730136,-9.99613698190578,-18.3703443006992));
#25502=CARTESIAN_POINT('Ctrl Pts',(82.3727560367574,-0.0100190419482207,
-20.9139236850969));
#25503=CARTESIAN_POINT('Ctrl Pts',(82.4916109005011,9.9785313724145,-18.3799133821952));
#25504=CARTESIAN_POINT('Ctrl Pts',(82.6104657642448,17.544442747166,-11.3835334136054));
#25505=CARTESIAN_POINT('Ctrl Pts',(82.7293206279886,20.8508243032301,-1.62340080174));
#25506=CARTESIAN_POINT('Ctrl Pts',(82.8481754917323,19.0949357636439,8.53086938533054));
#25507=CARTESIAN_POINT('Ctrl Pts',(82.9670303554759,12.7030807563111,16.6139713369771));
#25508=CARTESIAN_POINT('Ctrl Pts',(83.0858852192198,3.22710663214606,20.6634480925139));
#25509=CARTESIAN_POINT('Ctrl Pts',(83.2047400829634,-7.03236099624711,19.6961469101375));
#25510=CARTESIAN_POINT('Ctrl Pts',(83.3235949467073,-15.5844759437393,13.9469141334658));
#25511=CARTESIAN_POINT('Ctrl Pts',(83.4213050537529,-19.5045880027386,6.43679091069946));
#25512=CARTESIAN_POINT('Ctrl Pts',(83.4793968728842,-20.0645583422922,1.5531819665273));
#25513=CARTESIAN_POINT('Ctrl Pts',(83.4978704041008,-20.0642786305281,0.000103247315884208));
#25514=CARTESIAN_POINT('Origin',(65.9521295958992,0.,0.));
#25515=CARTESIAN_POINT('',(80.2021295958992,-20.0643601951534,-0.000193369559137528));
#25516=CARTESIAN_POINT('',(80.4978704041008,-20.0660058932225,0.000514059632016062));
#25517=CARTESIAN_POINT('',(65.9521295958992,-20.06595,-1.45722292471193E-12));
#25518=CARTESIAN_POINT('Ctrl Pts',(80.2021295958992,-20.0643601951534,-0.000193369559138151));
#25519=CARTESIAN_POINT('Ctrl Pts',(80.2193936583136,-20.0648522124826,-1.45157457243224));
#25520=CARTESIAN_POINT('Ctrl Pts',(80.2762760086426,-19.5530566810888,-6.23330384825486));
#25521=CARTESIAN_POINT('Ctrl Pts',(80.3727766468861,-15.7946418386806,-13.7084496778365));
#25522=CARTESIAN_POINT('Ctrl Pts',(80.49163151063,-7.33089175974107,-19.586993883415));
#25523=CARTESIAN_POINT('Ctrl Pts',(80.6104863743736,2.91268983041759,-20.7101072265152));
#25524=CARTESIAN_POINT('Ctrl Pts',(80.7293412381174,12.4491136405291,-16.8051144877733));
#25525=CARTESIAN_POINT('Ctrl Pts',(80.8481961018612,18.9630777731095,-8.82008983814658));
#25526=CARTESIAN_POINT('Ctrl Pts',(80.9670509656049,20.8730885973582,1.30632147223087));
#25527=CARTESIAN_POINT('Ctrl Pts',(81.0859058293486,17.7154238864056,11.1155773537385));
#25528=CARTESIAN_POINT('Ctrl Pts',(81.2047606930925,10.2567176785937,18.2261363388843));
#25529=CARTESIAN_POINT('Ctrl Pts',(81.323615556836,0.307832932572739,20.9116604378418));
#25530=CARTESIAN_POINT('Ctrl Pts',(81.44247042058,-9.71578907209836,18.5201443322797));
#25531=CARTESIAN_POINT('Ctrl Pts',(81.5613252843235,-17.3805619607799,11.6322125715389));
#25532=CARTESIAN_POINT('Ctrl Pts',(81.6478783427634,-19.8893188630231,4.55964969297058));
#25533=CARTESIAN_POINT('Ctrl Pts',(81.6948131132886,-20.0670550092625,0.615395449919073));
#25534=CARTESIAN_POINT('Ctrl Pts',(81.7021295958993,-20.0664325672107,0.000484799890658819));
#25535=CARTESIAN_POINT('Ctrl Pts',(80.4978704041008,-20.0660058932225,0.00051405963201627));
#25536=CARTESIAN_POINT('Ctrl Pts',(80.5285579629343,-20.0633649888413,-2.57876672415488));
#25537=CARTESIAN_POINT('Ctrl Pts',(80.5988638096823,-18.9190011292246,-8.490229143316));
#25538=CARTESIAN_POINT('Ctrl Pts',(80.708787944345,-13.2690058590392,-16.1655741562136));
#25539=CARTESIAN_POINT('Ctrl Pts',(80.8276428080888,-3.93846234853991,-20.5397375498421));
#25540=CARTESIAN_POINT('Ctrl Pts',(80.9464976718324,6.34828125649317,-19.9271580857812));
#25541=CARTESIAN_POINT('Ctrl Pts',(81.0653525355762,15.0937565693877,-14.4765609490419));
#25542=CARTESIAN_POINT('Ctrl Pts',(81.1842073993199,20.1746922266295,-5.51127007576585));
#25543=CARTESIAN_POINT('Ctrl Pts',(81.3030622630637,20.3575126025494,4.7920752210601));
#25544=CARTESIAN_POINT('Ctrl Pts',(81.4219171268074,15.5978316283554,13.9319759108582));
#25545=CARTESIAN_POINT('Ctrl Pts',(81.5407719905512,7.05122906962834,19.6894000135831));
#25546=CARTESIAN_POINT('Ctrl Pts',(81.6596268542949,-3.20730705765452,20.6665305681718));
#25547=CARTESIAN_POINT('Ctrl Pts',(81.7784817180386,-12.6871567229822,16.6261348055928));
#25548=CARTESIAN_POINT('Ctrl Pts',(81.891229567974,-18.7579286033266,8.96417271615029));
#25549=CARTESIAN_POINT('Ctrl Pts',(81.9643591299947,-20.06403759207,2.81587447866636));
#25550=CARTESIAN_POINT('Ctrl Pts',(81.9978704041008,-20.0667413636039,-0.000441116259225702));
#25551=CARTESIAN_POINT('Origin',(65.9521295958992,0.,0.));
#25552=CARTESIAN_POINT('',(78.7021295958992,-20.0675097952894,-0.000191679329453545));
#25553=CARTESIAN_POINT('',(78.9978704041008,-20.0645444704692,-0.000303457117966088));
#25554=CARTESIAN_POINT('',(65.9521295958992,-20.06595,-1.45722292471193E-12));
#25555=CARTESIAN_POINT('Ctrl Pts',(78.7021295958992,-20.0675097952894,-0.000191679329453777));
#25556=CARTESIAN_POINT('Ctrl Pts',(78.7043559154241,-20.0676030240896,-0.187272685098598));
#25557=CARTESIAN_POINT('Ctrl Pts',(78.7462005228635,-20.0194521966627,-3.70349040917738));
#25558=CARTESIAN_POINT('Ctrl Pts',(78.8276634182176,-18.0885635049867,-10.4974365303172));
#25559=CARTESIAN_POINT('Ctrl Pts',(78.9465182819614,-10.8797508184065,-17.8612240765116));
#25560=CARTESIAN_POINT('Ctrl Pts',(79.0653731457051,-1.02949641157685,-20.8885720076918));
#25561=CARTESIAN_POINT('Ctrl Pts',(79.1842280094488,9.07070441569705,-18.8444852618751));
#25562=CARTESIAN_POINT('Ctrl Pts',(79.3030828731926,16.9686730893506,-12.2252377060213));
#25563=CARTESIAN_POINT('Ctrl Pts',(79.4219377369363,20.7469002557211,-2.63788422057037));
#25564=CARTESIAN_POINT('Ctrl Pts',(79.5407926006801,19.488088539859,7.58990832912952));
#25565=CARTESIAN_POINT('Ctrl Pts',(79.6596474644237,13.4978587082429,15.9749839960573));
#25566=CARTESIAN_POINT('Ctrl Pts',(79.7785023281676,4.23054949116273,20.4815710917107));
#25567=CARTESIAN_POINT('Ctrl Pts',(79.8973571919112,-6.06387423543652,20.0155372807922));
#25568=CARTESIAN_POINT('Ctrl Pts',(80.0162120556551,-14.8860794655671,14.6900286428174));
#25569=CARTESIAN_POINT('Ctrl Pts',(80.1178028569843,-19.3376741497113,7.0895961574771));
#25570=CARTESIAN_POINT('Ctrl Pts',(80.179775370399,-20.0637231106675,1.87911533061271));
#25571=CARTESIAN_POINT('Ctrl Pts',(80.2021295958992,-20.0643601951534,-0.000193369559138151));
#25572=CARTESIAN_POINT('Ctrl Pts',(78.9978704041008,-20.0645444704692,-0.000303457117966088));
#25573=CARTESIAN_POINT('Ctrl Pts',(79.0135202200448,-20.0652525743057,-1.31594117297544));
#25574=CARTESIAN_POINT('Ctrl Pts',(79.0687883239033,-19.6151483119908,-5.96170308847767));
#25575=CARTESIAN_POINT('Ctrl Pts',(79.1636747156764,-16.0694521359249,-13.3852535403135));
#25576=CARTESIAN_POINT('Ctrl Pts',(79.2825295794202,-7.72668274442983,-19.4342655650835));
#25577=CARTESIAN_POINT('Ctrl Pts',(79.401384443164,2.49201032407988,-20.7649268920441));
#25578=CARTESIAN_POINT('Ctrl Pts',(79.5202393069076,12.1056803413097,-17.0541727375234));
#25579=CARTESIAN_POINT('Ctrl Pts',(79.6390941706514,18.7802711793142,-9.20291903249607));
#25580=CARTESIAN_POINT('Ctrl Pts',(79.7579490343951,20.8952914316842,0.882666569120876));
#25581=CARTESIAN_POINT('Ctrl Pts',(79.8768038981389,17.9372456308276,10.7539538527284));
#25582=CARTESIAN_POINT('Ctrl Pts',(79.9956587618826,10.6243033119855,18.014341048792));
#25583=CARTESIAN_POINT('Ctrl Pts',(80.1145136256262,0.731938129029032,20.9011141057727));
#25584=CARTESIAN_POINT('Ctrl Pts',(80.2333684893701,-9.33813074796676,18.7134074508395));
#25585=CARTESIAN_POINT('Ctrl Pts',(80.3522233531138,-17.1410403344121,11.982363729303));
#25586=CARTESIAN_POINT('Ctrl Pts',(80.4403906580241,-19.842194915655,4.83121342860229));
#25587=CARTESIAN_POINT('Ctrl Pts',(80.4889396750197,-20.0667744522885,0.751139354692291));
#25588=CARTESIAN_POINT('Ctrl Pts',(80.4978704041008,-20.0660058932225,0.00051405963201627));
#25589=CARTESIAN_POINT('Origin',(65.9521295958992,0.,0.));
#25590=CARTESIAN_POINT('',(77.2021295958992,-20.0650526848319,0.000450787506038296));
#25591=CARTESIAN_POINT('',(77.4978704041008,-20.0676486395731,-5.41331433023817E-5));
#25592=CARTESIAN_POINT('',(65.9521295958992,-20.06595,-1.45722292471193E-12));
#25593=CARTESIAN_POINT('Ctrl Pts',(77.2021295958992,-20.0650526848319,0.00045078750603833));
#25594=CARTESIAN_POINT('Ctrl Pts',(77.2289364604492,-20.0631870683403,-2.25296626175112));
#25595=CARTESIAN_POINT('Ctrl Pts',(77.2953616129137,-19.1243638779595,-7.83825946812389));
#25596=CARTESIAN_POINT('Ctrl Pts',(77.4014050532927,-14.0412530376615,-15.4995327837435));
#25597=CARTESIAN_POINT('Ctrl Pts',(77.5202599170366,-4.93502901298443,-20.323331223571));
#25598=CARTESIAN_POINT('Ctrl Pts',(77.6391147807802,5.3693466737219,-20.2129270438343));
#25599=CARTESIAN_POINT('Ctrl Pts',(77.7579696445241,14.3701248285384,-15.1951247376979));
#25600=CARTESIAN_POINT('Ctrl Pts',(77.8768245082677,19.8820503542049,-6.48817209195593));
#25601=CARTESIAN_POINT('Ctrl Pts',(77.9956793720115,20.566909693682,3.79401226064252));
#25602=CARTESIAN_POINT('Ctrl Pts',(78.1145342357552,16.2584291829867,13.1550668521213));
#25603=CARTESIAN_POINT('Ctrl Pts',(78.2333890994989,8.002643824371,19.3222668235958));
#25604=CARTESIAN_POINT('Ctrl Pts',(78.3522439632428,-2.19606445801497,20.7983077263084));
#25605=CARTESIAN_POINT('Ctrl Pts',(78.4710988269864,-11.8616009447801,17.2248287773426));
#25606=CARTESIAN_POINT('Ctrl Pts',(78.5877273712053,-18.5202110494551,9.61468733910552));
#25607=CARTESIAN_POINT('Ctrl Pts',(78.6647376275095,-20.0659439785636,3.14191212734159));
#25608=CARTESIAN_POINT('Ctrl Pts',(78.7021295958992,-20.0675097952894,-0.000191679329453777));
#25609=CARTESIAN_POINT('Ctrl Pts',(77.4978704041008,-20.0676486395731,-5.41331433030149E-5));
#25610=CARTESIAN_POINT('Ctrl Pts',(77.4984824771553,-20.0676566429987,-0.051486524418573));
#25611=CARTESIAN_POINT('Ctrl Pts',(77.5387128381243,-20.0549310784319,-3.43203271481463));
#25612=CARTESIAN_POINT('Ctrl Pts',(77.6185614870079,-18.2977702184867,-10.1283715037868));
#25613=CARTESIAN_POINT('Ctrl Pts',(77.7374163507516,-11.2398064531836,-17.636866365152));
#25614=CARTESIAN_POINT('Ctrl Pts',(77.8562712144954,-1.45298481342087,-20.8633923276927));
#25615=CARTESIAN_POINT('Ctrl Pts',(77.975126078239,8.68659993361501,-19.0245968651264));
#25616=CARTESIAN_POINT('Ctrl Pts',(78.0939809419828,16.7172073837676,-12.5669121734563));
#25617=CARTESIAN_POINT('Ctrl Pts',(78.2128358057265,20.6891254607372,-3.05816807208725));
#25618=CARTESIAN_POINT('Ctrl Pts',(78.3316906694703,19.6380315166033,7.19305376319089));
#25619=CARTESIAN_POINT('Ctrl Pts',(78.450545533214,13.8191155315665,15.6979091032047));
#25620=CARTESIAN_POINT('Ctrl Pts',(78.5694003969578,4.6451237813503,20.3915455359125));
#25621=CARTESIAN_POINT('Ctrl Pts',(78.6882552607015,-5.65663495145375,20.1344179283447));
#25622=CARTESIAN_POINT('Ctrl Pts',(78.8071101244452,-14.5850468304206,14.9889530402125));
#25623=CARTESIAN_POINT('Ctrl Pts',(78.910315172245,-19.2630610848218,7.36107071340815));
#25624=CARTESIAN_POINT('Ctrl Pts',(78.9739019321302,-20.0634599742031,2.01466118073625));
#25625=CARTESIAN_POINT('Ctrl Pts',(78.9978704041008,-20.0645444704692,-0.000303457117966088));
#25626=CARTESIAN_POINT('Origin',(65.9521295958992,0.,0.));
#25627=CARTESIAN_POINT('',(75.7021295958992,-20.0652872327308,-0.000485265228740224));
#25628=CARTESIAN_POINT('',(75.9978704041008,-20.0647373073215,0.000375534437402902));
#25629=CARTESIAN_POINT('',(65.9521295958992,-20.06595,-1.45722292471193E-12));
#25630=CARTESIAN_POINT('Ctrl Pts',(75.7021295958992,-20.0652872327308,-0.000485265228740428));
#25631=CARTESIAN_POINT('Ctrl Pts',(75.7138987175596,-20.0661846979473,-0.989778505806707));
#25632=CARTESIAN_POINT('Ctrl Pts',(75.7652861271346,-19.752403164384,-5.30875635559926));
#25633=CARTESIAN_POINT('Ctrl Pts',(75.8562918246243,-16.7028379804262,-12.5860044009848));
#25634=CARTESIAN_POINT('Ctrl Pts',(75.9751466883679,-8.66485747623899,-19.0345094052471));
#25635=CARTESIAN_POINT('Ctrl Pts',(76.0940015521117,1.47682157948402,-20.8617185630606));
#25636=CARTESIAN_POINT('Ctrl Pts',(76.2128564158554,11.2599503155789,-17.6240126609314));
#25637=CARTESIAN_POINT('Ctrl Pts',(76.3317112795992,18.3093305469575,-10.1074585482319));
#25638=CARTESIAN_POINT('Ctrl Pts',(76.4505661433428,20.9134775754992,-0.136963794739155));
#25639=CARTESIAN_POINT('Ctrl Pts',(76.5694210070867,18.4401432255183,9.86678373150789));
#25640=CARTESIAN_POINT('Ctrl Pts',(76.6882758708303,11.4898162994893,17.4750228837036));
#25641=CARTESIAN_POINT('Ctrl Pts',(76.8071307345741,1.74993282588505,20.8405863278091));
#25642=CARTESIAN_POINT('Ctrl Pts',(76.9259855983178,-8.41480831689548,19.1463653044614));
#25643=CARTESIAN_POINT('Ctrl Pts',(77.0448404620616,-16.5365591258767,12.8036914855974));
#25644=CARTESIAN_POINT('Ctrl Pts',(77.1368884612554,-19.7171928032765,5.4841267812297));
#25645=CARTESIAN_POINT('Ctrl Pts',(77.1893181725346,-20.0659442923776,1.07739433610062));
#25646=CARTESIAN_POINT('Ctrl Pts',(77.2021295958992,-20.0650526848319,0.00045078750603833));
#25647=CARTESIAN_POINT('Ctrl Pts',(75.9978704041008,-20.0647373073215,0.000375534437402764));
#25648=CARTESIAN_POINT('Ctrl Pts',(76.0230630221803,-20.0633086611632,-2.11744145806295));
#25649=CARTESIAN_POINT('Ctrl Pts',(76.0878739281744,-19.2044230293602,-7.566900804634));
#25650=CARTESIAN_POINT('Ctrl Pts',(76.192303122083,-14.352754093941,-15.2115335915258));
#25651=CARTESIAN_POINT('Ctrl Pts',(76.3111579858267,-5.34624865537712,-20.2190486819271));
#25652=CARTESIAN_POINT('Ctrl Pts',(76.4300128495705,4.95824645968282,-20.3176794032267));
#25653=CARTESIAN_POINT('Ctrl Pts',(76.5488677133142,14.0589530618911,-15.4834796829007));
#25654=CARTESIAN_POINT('Ctrl Pts',(76.667722577058,19.7463549128656,-6.8901213300209));
#25655=CARTESIAN_POINT('Ctrl Pts',(76.7865774408017,20.6396354130593,3.3760560278593));
#25656=CARTESIAN_POINT('Ctrl Pts',(76.9054323045454,16.5219193398244,12.8225771830625));
#25657=CARTESIAN_POINT('Ctrl Pts',(77.0242871682892,8.39292692660435,19.1559672658923));
#25658=CARTESIAN_POINT('Ctrl Pts',(77.1431420320329,-1.77374334422174,20.8385733397488));
#25659=CARTESIAN_POINT('Ctrl Pts',(77.2619968957766,-11.5097751060743,17.4618836697204));
#25660=CARTESIAN_POINT('Ctrl Pts',(77.380239686466,-18.4156569494689,9.88492971059405));
#25661=CARTESIAN_POINT('Ctrl Pts',(77.4588641892407,-20.0671385969634,3.27763125149108));
#25662=CARTESIAN_POINT('Ctrl Pts',(77.4978704041008,-20.0676486395731,-5.41331433030149E-5));
#25663=CARTESIAN_POINT('Origin',(65.9521295958992,0.,0.));
#25664=CARTESIAN_POINT('',(74.2021295958992,-20.0673524071727,0.000272503390984278));
#25665=CARTESIAN_POINT('',(74.4978704041008,-20.0656858399569,-0.000513895107878692));
#25666=CARTESIAN_POINT('',(65.9521295958992,-20.06595,-1.45722292471193E-12));
#25667=CARTESIAN_POINT('Ctrl Pts',(74.2021295958992,-20.0673524071727,0.000272503390984676));
#25668=CARTESIAN_POINT('Ctrl Pts',(74.2384792625847,-20.0653052780391,-3.05431469277528));
#25669=CARTESIAN_POINT('Ctrl Pts',(74.3144472171848,-18.5859398545859,-9.44007767698859));
#25670=CARTESIAN_POINT('Ctrl Pts',(74.4300334596993,-12.0861869801001,-17.0679930766342));
#25671=CARTESIAN_POINT('Ctrl Pts',(74.5488883234432,-2.46828348179083,-20.7677605926949));
#25672=CARTESIAN_POINT('Ctrl Pts',(74.6677431871868,7.74888254330118,-19.4254246468925));
#25673=CARTESIAN_POINT('Ctrl Pts',(74.7865980509306,16.0847351103166,-13.3668844467559));
#25674=CARTESIAN_POINT('Ctrl Pts',(74.9054529146743,20.5154531674799,-4.06306346429831));
#25675=CARTESIAN_POINT('Ctrl Pts',(75.024307778418,19.9653242538903,6.22720891081994));
#25676=CARTESIAN_POINT('Ctrl Pts',(75.1431626421618,14.5679114895243,15.0056075590215));
#25677=CARTESIAN_POINT('Ctrl Pts',(75.2620175059054,5.63362643574612,20.1408678205393));
#25678=CARTESIAN_POINT('Ctrl Pts',(75.3808723696493,-4.66841934638479,20.3862248635758));
#25679=CARTESIAN_POINT('Ctrl Pts',(75.499727233393,-13.8370423291352,15.6821096464633));
#25680=CARTESIAN_POINT('Ctrl Pts',(75.6068129754763,-19.0710051864169,8.01342804802537));
#25681=CARTESIAN_POINT('Ctrl Pts',(75.6742804296451,-20.0631635688974,2.34047039194829));
#25682=CARTESIAN_POINT('Ctrl Pts',(75.7021295958992,-20.0652872327308,-0.000485265228740428));
#25683=CARTESIAN_POINT('Ctrl Pts',(74.4978704041009,-20.0656858399569,-0.000513895107878137));
#25684=CARTESIAN_POINT('Ctrl Pts',(74.5080252792908,-20.0665335258616,-0.854067493707957));
#25685=CARTESIAN_POINT('Ctrl Pts',(74.5577984423954,-19.8045579242786,-5.03716326470863));
#25686=CARTESIAN_POINT('Ctrl Pts',(74.6471898934143,-16.9546939409116,-12.2446174973853));
#25687=CARTESIAN_POINT('Ctrl Pts',(74.7660447571583,-9.04916751458383,-18.8548368218943));
#25688=CARTESIAN_POINT('Ctrl Pts',(74.8848996209018,1.05336222602103,-20.8873821315178));
#25689=CARTESIAN_POINT('Ctrl Pts',(75.0037544846458,10.9001512813116,-17.8487816483865));
#25690=CARTESIAN_POINT('Ctrl Pts',(75.1226093483893,18.1005456873079,-10.4767623867747));
#25691=CARTESIAN_POINT('Ctrl Pts',(75.2414642121331,20.9063967498254,-0.561141003802912));
#25692=CARTESIAN_POINT('Ctrl Pts',(75.3603190758769,18.6364855530042,9.4907170709027));
#25693=CARTESIAN_POINT('Ctrl Pts',(75.4791739396206,11.8419127825698,17.2383701647594));
#25694=CARTESIAN_POINT('Ctrl Pts',(75.5980288033644,2.1722996740317,20.8008033117344));
#25695=CARTESIAN_POINT('Ctrl Pts',(75.7168836671081,-8.02471549395103,19.3131107159981));
#25696=CARTESIAN_POINT('Ctrl Pts',(75.8357385308518,-16.2734490649882,13.1364820182761));
#25697=CARTESIAN_POINT('Ctrl Pts',(75.929400776516,-19.6602681817825,5.7557332003338));
#25698=CARTESIAN_POINT('Ctrl Pts',(75.9834447342657,-20.0655553714753,1.21306921353621));
#25699=CARTESIAN_POINT('Ctrl Pts',(75.9978704041008,-20.0647373073215,0.000375534437402764));
#25700=CARTESIAN_POINT('Origin',(65.9521295958992,0.,0.));
#25701=CARTESIAN_POINT('',(72.7021295958992,-20.0642869035746,0.000115967843645696));
#25702=CARTESIAN_POINT('',(72.9978704041008,-20.0670305035468,0.000378951515905696));
#25703=CARTESIAN_POINT('',(65.9521295958992,-20.06595,-1.45722292471193E-12));
#25704=CARTESIAN_POINT('Ctrl Pts',(72.7021295958992,-20.0642869035746,0.000115967843645898));
#25705=CARTESIAN_POINT('Ctrl Pts',(72.7234415196951,-20.0639242759761,-1.7915856698192));
#25706=CARTESIAN_POINT('Ctrl Pts',(72.7843717314056,-19.3842247051702,-6.91428185345562));
#25707=CARTESIAN_POINT('Ctrl Pts',(72.8849202310308,-15.0772063355693,-14.4937970351682));
#25708=CARTESIAN_POINT('Ctrl Pts',(73.0037750947745,-6.32550909580307,-19.9343983621499));
#25709=CARTESIAN_POINT('Ctrl Pts',(73.1226299585183,3.96192769410095,-20.5352241850118));
#25710=CARTESIAN_POINT('Ctrl Pts',(73.241484822262,13.2874673524912,-16.1504029280528));
#25711=CARTESIAN_POINT('Ctrl Pts',(73.3603396860058,19.3870075181409,-7.84450399155505));
#25712=CARTESIAN_POINT('Ctrl Pts',(73.4791945497494,20.7796705370668,2.36592386879463));
#25713=CARTESIAN_POINT('Ctrl Pts',(73.5980494134933,17.1273385367331,12.0019405943419));
#25714=CARTESIAN_POINT('Ctrl Pts',(73.7169042772369,9.31674341779712,18.7240646086503));
#25715=CARTESIAN_POINT('Ctrl Pts',(73.8357591409808,-0.75581846594697,20.9002641569074));
#25716=CARTESIAN_POINT('Ctrl Pts',(73.9546140047244,-10.6448788649411,18.0021903481967));
#25717=CARTESIAN_POINT('Ctrl Pts',(74.0734688684682,-17.9495209615153,10.7334524098305));
#25718=CARTESIAN_POINT('Ctrl Pts',(74.1559740655264,-19.9950700033997,3.87878284554617));
#25719=CARTESIAN_POINT('Ctrl Pts',(74.1988609746701,-20.0675364883585,0.274945958911929));
#25720=CARTESIAN_POINT('Ctrl Pts',(74.2021295958992,-20.0673524071727,0.000272503390984676));
#25721=CARTESIAN_POINT('Ctrl Pts',(72.9978704041008,-20.0670305035468,0.00037895151590521));
#25722=CARTESIAN_POINT('Ctrl Pts',(73.0326058243158,-20.0645045081021,-2.9186932831106));
#25723=CARTESIAN_POINT('Ctrl Pts',(73.1069595324454,-18.6850026481514,-9.16949023623251));
#25724=CARTESIAN_POINT('Ctrl Pts',(73.2209315284896,-12.429904644976,-16.8193274183025));
#25725=CARTESIAN_POINT('Ctrl Pts',(73.3397863922333,-2.88902535394313,-20.7134216582276));
#25726=CARTESIAN_POINT('Ctrl Pts',(73.4586412559771,7.35326633413225,-19.5786051215753));
#25727=CARTESIAN_POINT('Ctrl Pts',(73.5774961197208,15.8102942970291,-13.6903943890812));
#25728=CARTESIAN_POINT('Ctrl Pts',(73.6963509834645,20.4288178986918,-4.47835947076039));
#25729=CARTESIAN_POINT('Ctrl Pts',(73.8152058472083,20.0875282846243,5.82095453526969));
#25730=CARTESIAN_POINT('Ctrl Pts',(73.934060710952,14.8692854982535,14.7070273358924));
#25731=CARTESIAN_POINT('Ctrl Pts',(74.0529155746958,6.04100129448752,20.0224525882135));
#25732=CARTESIAN_POINT('Ctrl Pts',(74.1717704384394,-4.25394819579815,20.4767240796648));
#25733=CARTESIAN_POINT('Ctrl Pts',(74.2906253021834,-13.5161023190106,15.9595514469955));
#25734=CARTESIAN_POINT('Ctrl Pts',(74.3993252907369,-18.9857656765303,8.28463624677858));
#25735=CARTESIAN_POINT('Ctrl Pts',(74.4684069913762,-20.0632263592439,2.47599137823915));
#25736=CARTESIAN_POINT('Ctrl Pts',(74.4978704041009,-20.0656858399569,-0.000513895107878137));
#25737=CARTESIAN_POINT('Origin',(65.9521295958992,0.,0.));
#25738=CARTESIAN_POINT('',(71.2021295958992,-20.0666997414326,-0.000448233882077294));
#25739=CARTESIAN_POINT('',(71.4978704041008,-20.0642475748551,-8.67278534544269E-6));
#25740=CARTESIAN_POINT('',(65.9521295958992,-20.06595,-1.45722292471193E-12));
#25741=CARTESIAN_POINT('Ctrl Pts',(71.2021295958992,-20.0666997414326,-0.000448233882078958));
#25742=CARTESIAN_POINT('Ctrl Pts',(71.2084037768056,-20.0672110152629,-0.527738819280344));
#25743=CARTESIAN_POINT('Ctrl Pts',(71.2542962456266,-19.9182399737843,-4.38431536006082));
#25744=CARTESIAN_POINT('Ctrl Pts',(71.3398070023622,-17.5314248864508,-11.4035715815495));
#25745=CARTESIAN_POINT('Ctrl Pts',(71.458661866106,-9.95752466116282,-18.3913024557491));
#25746=CARTESIAN_POINT('Ctrl Pts',(71.5775167298497,0.0339144865576418,
-20.9138985648547));
#25747=CARTESIAN_POINT('Ctrl Pts',(71.6963715935934,10.017119701265,-18.3589110863466));
#25748=CARTESIAN_POINT('Ctrl Pts',(71.8152264573371,17.5683172038997,-11.3466529868452));
#25749=CARTESIAN_POINT('Ctrl Pts',(71.9340813210809,20.8541885247641,-1.57959626350904));
#25750=CARTESIAN_POINT('Ctrl Pts',(72.0529361848246,19.0769729670116,8.57096294462323));
#25751=CARTESIAN_POINT('Ctrl Pts',(72.1717910485684,12.6681520414353,16.640619797256));
#25752=CARTESIAN_POINT('Ctrl Pts',(72.2906459123121,3.18369217161882,20.670181603907));
#25753=CARTESIAN_POINT('Ctrl Pts',(72.4095007760559,-7.07372081696884,19.6813306761887));
#25754=CARTESIAN_POINT('Ctrl Pts',(72.5283556397995,-15.6137395751919,13.9141453154726));
#25755=CARTESIAN_POINT('Ctrl Pts',(72.6258985797474,-19.5113868904301,6.40866649789178));
#25756=CARTESIAN_POINT('Ctrl Pts',(72.6838232317806,-20.0645983908398,1.53913904642774));
#25757=CARTESIAN_POINT('Ctrl Pts',(72.7021295958992,-20.0642869035746,0.000115967843645898));
#25758=CARTESIAN_POINT('Ctrl Pts',(71.4978704041008,-20.0642475748551,-8.67278534502636E-6));
#25759=CARTESIAN_POINT('Ctrl Pts',(71.5175680814263,-20.064272580664,-1.65600928132531));
#25760=CARTESIAN_POINT('Ctrl Pts',(71.5768840466664,-19.4538205919808,-6.64273518489432));
#25761=CARTESIAN_POINT('Ctrl Pts',(71.6758182998211,-15.3680940867467,-14.1849916611866));
#25762=CARTESIAN_POINT('Ctrl Pts',(71.7946731635647,-6.72855361766429,-19.8019915791725));
#25763=CARTESIAN_POINT('Ctrl Pts',(71.9135280273086,3.54457961832131,-20.6113623910834));
#25764=CARTESIAN_POINT('Ctrl Pts',(72.0323828910522,12.9571416297572,-16.416600898898));
#25765=CARTESIAN_POINT('Ctrl Pts',(72.151237754796,19.2239023220937,-8.2361328181285));
#25766=CARTESIAN_POINT('Ctrl Pts',(72.2700926185397,20.8233853839836,1.94394584218601));
#25767=CARTESIAN_POINT('Ctrl Pts',(72.3889474822834,17.3672601118087,11.6520633578796));
#25768=CARTESIAN_POINT('Ctrl Pts',(72.5078023460272,9.69462233016103,18.5312331527829));
#25769=CARTESIAN_POINT('Ctrl Pts',(72.6266572097709,-0.331725597276454,
20.9112950917769));
#25770=CARTESIAN_POINT('Ctrl Pts',(72.7455120735146,-10.2775354823501,18.2144055268431));
#25771=CARTESIAN_POINT('Ctrl Pts',(72.8643669372584,-17.7281125760169,11.0953291424513));
#25772=CARTESIAN_POINT('Ctrl Pts',(72.9484863807871,-19.9550137979455,4.15028650086484));
#25773=CARTESIAN_POINT('Ctrl Pts',(72.9929875364012,-20.0673855907025,0.410722152746902));
#25774=CARTESIAN_POINT('Ctrl Pts',(72.9978704041008,-20.0670305035468,0.00037895151590521));
#25775=CARTESIAN_POINT('Origin',(65.9521295958992,0.,0.));
#25776=CARTESIAN_POINT('',(69.7021295958992,-20.0660502412321,0.000515820514980686));
#25777=CARTESIAN_POINT('',(69.9978704041008,-20.0670795681067,-0.000365800382556847));
#25778=CARTESIAN_POINT('',(65.9521295958992,-20.06595,-1.45722292471193E-12));
#25779=CARTESIAN_POINT('Ctrl Pts',(69.7021295958992,-20.0660502412321,0.000515820514980642));
#25780=CARTESIAN_POINT('Ctrl Pts',(69.7329843218307,-20.0633906478449,-2.59279908898246));
#25781=CARTESIAN_POINT('Ctrl Pts',(69.8034573356767,-18.9097406875408,-8.51830359478506));
#25782=CARTESIAN_POINT('Ctrl Pts',(69.9135486374375,-13.2350179122529,-16.1934098084835));
#25783=CARTESIAN_POINT('Ctrl Pts',(70.032403501181,-3.89530615487391,-20.5479670028002));
#25784=CARTESIAN_POINT('Ctrl Pts',(70.1512583649248,6.39012784832653,-19.9137776962236));
#25785=CARTESIAN_POINT('Ctrl Pts',(70.2701132286686,15.124133913895,-14.4448221531172));
#25786=CARTESIAN_POINT('Ctrl Pts',(70.3889680924123,20.1862251131474,-5.46887711782098));
#25787=CARTESIAN_POINT('Ctrl Pts',(70.5078229561561,20.3474010396572,4.83482921676092));
#25788=CARTESIAN_POINT('Ctrl Pts',(70.6266778198998,15.5685305420084,13.9647112886144));
#25789=CARTESIAN_POINT('Ctrl Pts',(70.7455326836435,7.00985233357066,19.7041689177776));
#25790=CARTESIAN_POINT('Ctrl Pts',(70.8643875473874,-3.25071379005506,20.6597474264871));
#25791=CARTESIAN_POINT('Ctrl Pts',(70.9832424111308,-12.7220549410739,16.599446414106));
#25792=CARTESIAN_POINT('Ctrl Pts',(71.0958230939684,-18.7677410467943,8.9361274774765));
#25793=CARTESIAN_POINT('Ctrl Pts',(71.168785488891,-20.063982578896,2.80183527788421));
#25794=CARTESIAN_POINT('Ctrl Pts',(71.2021295958992,-20.0666997414326,-0.000448233882078958));
#25795=CARTESIAN_POINT('Ctrl Pts',(69.9978704041008,-20.0670795681067,-0.000365800382557055));
#25796=CARTESIAN_POINT('Ctrl Pts',(70.0025303385367,-20.0674098044427,-0.391971507738714));
#25797=CARTESIAN_POINT('Ctrl Pts',(70.0468085608873,-19.9607121949208,-4.11278923178899));
#25798=CARTESIAN_POINT('Ctrl Pts',(70.1307050711525,-17.7591261183169,-11.0456210793205));
#25799=CARTESIAN_POINT('Ctrl Pts',(70.2495599348961,-10.3285220474192,-18.1855419414053));
#25800=CARTESIAN_POINT('Ctrl Pts',(70.36841479864,-0.390306419466782,-20.9102837301104));
#25801=CARTESIAN_POINT('Ctrl Pts',(70.4872696623836,9.64266981062011,-18.5583195092622));
#25802=CARTESIAN_POINT('Ctrl Pts',(70.6061245261274,17.3345491904711,-11.7006712929421));
#25803=CARTESIAN_POINT('Ctrl Pts',(70.724979389871,20.8178577880174,-2.00227405925465));
#25804=CARTESIAN_POINT('Ctrl Pts',(70.843834253615,19.2469000686554,8.18224553636222));
#25805=CARTESIAN_POINT('Ctrl Pts',(70.9626891173585,13.0030812084345,16.3802375864514));
#25806=CARTESIAN_POINT('Ctrl Pts',(71.0815439811024,3.602307582272,20.6013515178363));
#25807=CARTESIAN_POINT('Ctrl Pts',(71.200398844846,-6.67305275956469,19.8207636371352));
#25808=CARTESIAN_POINT('Ctrl Pts',(71.3192537085899,-15.3282951176304,14.2279890734018));
#25809=CARTESIAN_POINT('Ctrl Pts',(71.4184108950081,-19.4443890451087,6.68023871912706));
#25810=CARTESIAN_POINT('Ctrl Pts',(71.4779497935117,-20.0642222860368,1.6747341262207));
#25811=CARTESIAN_POINT('Ctrl Pts',(71.4978704041008,-20.0642475748551,-8.67278534502636E-6));
#25812=CARTESIAN_POINT('Origin',(157.6,0.,0.));
#25813=CARTESIAN_POINT('',(150.481156847152,-16.4244471060171,0.000374833880845693));
#25814=CARTESIAN_POINT('',(150.268843152848,-16.4246125179457,0.00027738966988146));
#25815=CARTESIAN_POINT('',(157.6,-16.425,-2.01148236759953E-15));
#25816=CARTESIAN_POINT('',(150.,7.06535955977556,14.8277213114857));
#25817=CARTESIAN_POINT('Ctrl Pts',(150.481156847152,-16.4244471060171,0.000374833880845693));
#25818=CARTESIAN_POINT('Ctrl Pts',(150.469297185807,-16.4251539191907,0.816394811968673));
#25819=CARTESIAN_POINT('Ctrl Pts',(150.457437524463,-16.3653909517533,1.63231199317137));
#25820=CARTESIAN_POINT('Ctrl Pts',(150.445577863118,-16.2442674552976,2.43901578219437));
#25821=CARTESIAN_POINT('Ctrl Pts',(150.406346587624,-15.8435958745298,5.10755897833262));
#25822=CARTESIAN_POINT('Ctrl Pts',(150.367115312129,-14.7714809451613,7.67528376569759));
#25823=CARTESIAN_POINT('Ctrl Pts',(150.327884036635,-13.1555893470951,9.83643486497512));
#25824=CARTESIAN_POINT('Ctrl Pts',(150.288652761141,-11.5396977490288,11.9975859642527));
#25825=CARTESIAN_POINT('Ctrl Pts',(150.249421485646,-9.3800294822648,13.7521633754428));
#25826=CARTESIAN_POINT('Ctrl Pts',(150.210190210152,-6.93376160152484,14.891209239928));
#25827=CARTESIAN_POINT('Ctrl Pts',(150.170958934657,-4.48749372078487,16.0302551044133));
#25828=CARTESIAN_POINT('Ctrl Pts',(150.131727659163,-1.75462622606894,16.5537694221937));
#25829=CARTESIAN_POINT('Ctrl Pts',(150.092496383669,0.939415135284274,16.399456771981));
#25830=CARTESIAN_POINT('Ctrl Pts',(150.061664255779,3.05668067779249,16.2781814041431));
#25831=CARTESIAN_POINT('Ctrl Pts',(150.03083212789,5.14996527585529,15.7382465032741));
#25832=CARTESIAN_POINT('Ctrl Pts',(150.,7.06578282810915,14.8277078846934));
#25833=CARTESIAN_POINT('',(150.,-7.06535955977601,14.8277213114855));
#25834=CARTESIAN_POINT('Origin',(150.,0.,0.));
#25835=CARTESIAN_POINT('Ctrl Pts',(150.,-7.06535955977558,14.8277213114857));
#25836=CARTESIAN_POINT('Ctrl Pts',(150.039231275494,-9.50202246794195,13.6666595940101));
#25837=CARTESIAN_POINT('Ctrl Pts',(150.078462550989,-11.6458626324014,11.8940710533159));
#25838=CARTESIAN_POINT('Ctrl Pts',(150.117693826483,-13.2424554823458,9.71901539710664));
#25839=CARTESIAN_POINT('Ctrl Pts',(150.156925101978,-14.8390483322902,7.54395974089736));
#25840=CARTESIAN_POINT('Ctrl Pts',(150.196156377472,-15.8883938677195,4.96643696917295));
#25841=CARTESIAN_POINT('Ctrl Pts',(150.235387652966,-16.2653432504906,2.29434249478256));
#25842=CARTESIAN_POINT('Ctrl Pts',(150.24653948626,-16.3724944104754,1.53477626226827));
#25843=CARTESIAN_POINT('Ctrl Pts',(150.257691319554,-16.4253139196711,0.767568349022371));
#25844=CARTESIAN_POINT('Ctrl Pts',(150.268843152848,-16.4246125179457,0.00027738966988146));
#25845=CARTESIAN_POINT('Origin',(157.6,0.,0.));
#25846=CARTESIAN_POINT('',(151.981156847152,-16.4262658875693,0.000126548556290129));
#25847=CARTESIAN_POINT('',(151.768843152848,-16.4263175731226,7.92183299041088E-5));
#25848=CARTESIAN_POINT('',(157.6,-16.425,-2.01148236759953E-15));
#25849=CARTESIAN_POINT('Ctrl Pts',(151.981156847152,-16.4262658875693,0.000126548556290129));
#25850=CARTESIAN_POINT('Ctrl Pts',(151.979303767234,-16.4263192176211,0.127589430577028));
#25851=CARTESIAN_POINT('Ctrl Pts',(151.977450687317,-16.4248658227487,0.255051093337995));
#25852=CARTESIAN_POINT('Ctrl Pts',(151.9755976074,-16.4218979730467,0.38247748338803));
#25853=CARTESIAN_POINT('Ctrl Pts',(151.936366331905,-16.3590660745457,3.08020237174462));
#25854=CARTESIAN_POINT('Ctrl Pts',(151.897135056411,-15.6174481672167,5.76211785977663));
#25855=CARTESIAN_POINT('Ctrl Pts',(151.857903780916,-14.285356483579,8.10886010496594));
#25856=CARTESIAN_POINT('Ctrl Pts',(151.818672505422,-12.9532647999413,10.4556023501552));
#25857=CARTESIAN_POINT('Ctrl Pts',(151.779441229928,-11.030699339995,12.4671713525018));
#25858=CARTESIAN_POINT('Ctrl Pts',(151.740209954433,-8.74660016284646,13.9040284681142));
#25859=CARTESIAN_POINT('Ctrl Pts',(151.700978678939,-6.46250098569791,15.3408855837265));
#25860=CARTESIAN_POINT('Ctrl Pts',(151.661747403444,-3.81686809134713,16.2030308126046));
#25861=CARTESIAN_POINT('Ctrl Pts',(151.62251612795,-1.12474477240116,16.3877994644907));
#25862=CARTESIAN_POINT('Ctrl Pts',(151.583284852456,1.56737854654481,16.5725681163767));
#25863=CARTESIAN_POINT('Ctrl Pts',(151.544053576961,4.30599229008596,16.0799601912707));
#25864=CARTESIAN_POINT('Ctrl Pts',(151.504822301467,6.76498096092394,14.9686356960831));
#25865=CARTESIAN_POINT('Ctrl Pts',(151.465591025972,9.22396963176194,13.8573112008954));
#25866=CARTESIAN_POINT('Ctrl Pts',(151.426359750478,11.4033332298968,12.127270135626));
#25867=CARTESIAN_POINT('Ctrl Pts',(151.387128474984,13.0435520428528,9.9845266415244));
#25868=CARTESIAN_POINT('Ctrl Pts',(151.347897199489,14.6837708558089,7.84178314742278));
#25869=CARTESIAN_POINT('Ctrl Pts',(151.308665923995,15.7848448835862,5.28633722448888));
#25870=CARTESIAN_POINT('Ctrl Pts',(151.2694346485,16.21565768281,2.62249268910952));
#25871=CARTESIAN_POINT('Ctrl Pts',(151.230203373006,16.6464704820338,-0.0413518462698437));
#25872=CARTESIAN_POINT('Ctrl Pts',(151.190972097512,16.407022052704,-2.81359499409468));
#25873=CARTESIAN_POINT('Ctrl Pts',(151.151740822017,15.5258260253638,-5.36411671960683));
#25874=CARTESIAN_POINT('Ctrl Pts',(151.112509546523,14.6446299980235,-7.91463844511896));
#25875=CARTESIAN_POINT('Ctrl Pts',(151.073278271028,13.1216863726727,-10.2434387483184));
#25876=CARTESIAN_POINT('Ctrl Pts',(151.034046995534,11.1383480576346,-12.0732027776573));
#25877=CARTESIAN_POINT('Ctrl Pts',(150.99481572004,9.15500974259645,-13.9029668069962));
#25878=CARTESIAN_POINT('Ctrl Pts',(150.955584444545,6.71127673787098,-15.2336945624745));
#25879=CARTESIAN_POINT('Ctrl Pts',(150.916353169051,4.0981499595583,-15.9069226094236));
#25880=CARTESIAN_POINT('Ctrl Pts',(150.877121893557,1.4850231812456,-16.5801506563726));
#25881=CARTESIAN_POINT('Ctrl Pts',(150.837890618062,-1.29749737065429,-16.5958789947925));
#25882=CARTESIAN_POINT('Ctrl Pts',(150.798659342568,-3.91806767946161,-15.9522340832658));
#25883=CARTESIAN_POINT('Ctrl Pts',(150.759428067073,-6.53863798826892,-15.3085891717391));
#25884=CARTESIAN_POINT('Ctrl Pts',(150.720196791579,-8.99725805398366,-14.0055710102659));
#25885=CARTESIAN_POINT('Ctrl Pts',(150.680965516085,-11.0011543169579,-12.198344892025));
#25886=CARTESIAN_POINT('Ctrl Pts',(150.64173424059,-13.0050505799322,-10.3911187737841));
#25887=CARTESIAN_POINT('Ctrl Pts',(150.602502965096,-14.554223040166,-8.0796846987755));
#25888=CARTESIAN_POINT('Ctrl Pts',(150.563271689601,-15.4641951541993,-5.53928685881544));
#25889=CARTESIAN_POINT('Ctrl Pts',(150.535900075452,-16.0990816134985,-3.76685431395997));
#25890=CARTESIAN_POINT('Ctrl Pts',(150.508528461302,-16.4228158100718,-1.88296595721331));
#25891=CARTESIAN_POINT('Ctrl Pts',(150.481156847152,-16.4244471060171,0.000374833880845693));
#25892=CARTESIAN_POINT('Ctrl Pts',(150.268843152848,-16.4246125179457,0.00027738966988146));
#25893=CARTESIAN_POINT('Ctrl Pts',(150.296922595049,-16.422846443374,-1.93170110895333));
#25894=CARTESIAN_POINT('Ctrl Pts',(150.325002037249,-16.0817615771842,-3.86420611402143));
#25895=CARTESIAN_POINT('Ctrl Pts',(150.35308147945,-15.4143001207446,-5.67657577670535));
#25896=CARTESIAN_POINT('Ctrl Pts',(150.392312754944,-14.4817543781148,-8.20873339674647));
#25897=CARTESIAN_POINT('Ctrl Pts',(150.431544030438,-12.9121096627423,-10.5063824597724));
#25898=CARTESIAN_POINT('Ctrl Pts',(150.470775305933,-10.892224580038,-12.2957350119018));
#25899=CARTESIAN_POINT('Ctrl Pts',(150.510006581427,-8.87233949733361,-14.0850875640313));
#25900=CARTESIAN_POINT('Ctrl Pts',(150.549237856922,-6.4022140472974,-15.3661436052642));
#25901=CARTESIAN_POINT('Ctrl Pts',(150.588469132416,-3.77601912020898,-15.9864431089081));
#25902=CARTESIAN_POINT('Ctrl Pts',(150.62770040791,-1.14982419312056,-16.6067426125519));
#25903=CARTESIAN_POINT('Ctrl Pts',(150.666931683405,1.63244021102008,-16.5662855786066));
#25904=CARTESIAN_POINT('Ctrl Pts',(150.706162958899,4.23947386602044,-15.8698463806454));
#25905=CARTESIAN_POINT('Ctrl Pts',(150.745394234394,6.84650752102081,-15.1734071826843));
#25906=CARTESIAN_POINT('Ctrl Pts',(150.784625509888,9.2783104268809,-13.8209858207073));
#25907=CARTESIAN_POINT('Ctrl Pts',(150.823856785382,11.2452958317145,-11.9736504010225));
#25908=CARTESIAN_POINT('Ctrl Pts',(150.863088060877,13.212281236548,-10.1263149813378));
#25909=CARTESIAN_POINT('Ctrl Pts',(150.902319336371,14.714449140355,-7.78406550394527));
#25910=CARTESIAN_POINT('Ctrl Pts',(150.941550611866,15.572923775988,-5.22580792961083));
#25911=CARTESIAN_POINT('Ctrl Pts',(150.98078188736,16.4313984116209,-2.6675503552764));
#25912=CARTESIAN_POINT('Ctrl Pts',(151.020013162854,16.6461797790798,0.10671531599998));
#25913=CARTESIAN_POINT('Ctrl Pts',(151.059244438349,16.1916900745551,2.7666231243286));
#25914=CARTESIAN_POINT('Ctrl Pts',(151.098475713843,15.7372003700303,5.42653093265725));
#25915=CARTESIAN_POINT('Ctrl Pts',(151.137706989338,14.6134395935219,7.97208087803814));
#25916=CARTESIAN_POINT('Ctrl Pts',(151.176938264832,12.9542264882274,10.1001500394191));
#25917=CARTESIAN_POINT('Ctrl Pts',(151.216169540326,11.2950133829329,12.2282192008));
#25918=CARTESIAN_POINT('Ctrl Pts',(151.255400815821,9.10034794885215,13.9388075781811));
#25919=CARTESIAN_POINT('Ctrl Pts',(151.294632091315,6.63157168295718,15.0282162584893));
#25920=CARTESIAN_POINT('Ctrl Pts',(151.333863366809,4.1627954170622,16.1176249387976));
#25921=CARTESIAN_POINT('Ctrl Pts',(151.373094642304,1.41990831935294,16.585853922033));
#25922=CARTESIAN_POINT('Ctrl Pts',(151.412325917798,-1.27046506139402,16.3771468466143));
#25923=CARTESIAN_POINT('Ctrl Pts',(151.451557193293,-3.96083844214098,16.1684397711956));
#25924=CARTESIAN_POINT('Ctrl Pts',(151.490788468787,-6.59869810592565,15.2827966371228));
#25925=CARTESIAN_POINT('Ctrl Pts',(151.530019744281,-8.86992648726269,13.8256799900127));
#25926=CARTESIAN_POINT('Ctrl Pts',(151.569251019776,-11.1411548685997,12.3685633429027));
#25927=CARTESIAN_POINT('Ctrl Pts',(151.60848229527,-13.0457519674892,10.3399731827554));
#25928=CARTESIAN_POINT('Ctrl Pts',(151.647713570765,-14.3569173638976,7.98147518136614));
#25929=CARTESIAN_POINT('Ctrl Pts',(151.686944846259,-15.6680827603059,5.62297717997691));
#25930=CARTESIAN_POINT('Ctrl Pts',(151.726176121753,-16.3858164542333,2.93457133734574));
#25931=CARTESIAN_POINT('Ctrl Pts',(151.765407397248,-16.4246503779292,0.236394302476631));
#25932=CARTESIAN_POINT('Ctrl Pts',(151.766552649115,-16.4257840301759,0.157628260661814));
#25933=CARTESIAN_POINT('Ctrl Pts',(151.767697900981,-16.4263391298596,0.078853891920753));
#25934=CARTESIAN_POINT('Ctrl Pts',(151.768843152848,-16.4263175731226,7.92183299041088E-5));
#25935=CARTESIAN_POINT('Origin',(157.6,0.,0.));
#25936=CARTESIAN_POINT('',(153.481156847152,-16.4251954303659,-0.000393763598601771));
#25937=CARTESIAN_POINT('',(153.268843152848,-16.4250464537185,-0.000400491521010713));
#25938=CARTESIAN_POINT('',(157.6,-16.425,-2.01148236759953E-15));
#25939=CARTESIAN_POINT('Ctrl Pts',(153.481156847152,-16.4251954303659,-0.000393763598601771));
#25940=CARTESIAN_POINT('Ctrl Pts',(153.450079073167,-16.4230658025619,2.13767372058375));
#25941=CARTESIAN_POINT('Ctrl Pts',(153.419001299182,-16.0032991920971,4.27655312283435));
#25942=CARTESIAN_POINT('Ctrl Pts',(153.387923525198,-15.1895390617785,6.25323317595138));
#25943=CARTESIAN_POINT('Ctrl Pts',(153.348692249703,-14.1622824804465,8.74851098337746));
#25944=CARTESIAN_POINT('Ctrl Pts',(153.309460974209,-12.5071784595547,10.9853164025025));
#25945=CARTESIAN_POINT('Ctrl Pts',(153.270229698715,-10.4213176161215,12.6972895220213));
#25946=CARTESIAN_POINT('Ctrl Pts',(153.23099842322,-8.33545677268826,14.4092626415401));
#25947=CARTESIAN_POINT('Ctrl Pts',(153.191767147726,-5.81883910671363,15.5964034614527));
#25948=CARTESIAN_POINT('Ctrl Pts',(153.152535872231,-3.17114471221293,16.1173466574469));
#25949=CARTESIAN_POINT('Ctrl Pts',(153.113304596737,-0.523450317712208,
16.6382898534412));
#25950=CARTESIAN_POINT('Ctrl Pts',(153.074073321243,2.25532080531457,16.4930354255172));
#25951=CARTESIAN_POINT('Ctrl Pts',(153.034842045748,4.83427119768834,15.6988803438118));
#25952=CARTESIAN_POINT('Ctrl Pts',(152.995610770254,7.41322159006212,14.9047252621064));
#25953=CARTESIAN_POINT('Ctrl Pts',(152.95637949476,9.79235125178288,13.4616695266198));
#25954=CARTESIAN_POINT('Ctrl Pts',(152.917148219265,11.6883522293468,11.5415529381808));
#25955=CARTESIAN_POINT('Ctrl Pts',(152.877916943771,13.5843532069107,9.6214363497418));
#25956=CARTESIAN_POINT('Ctrl Pts',(152.838685668276,14.9972255003178,7.22425890835048));
#25957=CARTESIAN_POINT('Ctrl Pts',(152.799454392782,15.7587235681631,4.63547770616391));
#25958=CARTESIAN_POINT('Ctrl Pts',(152.760223117288,16.5202216360085,2.04669650397737));
#25959=CARTESIAN_POINT('Ctrl Pts',(152.720991841793,16.6303454782922,-0.733688459004435));
#25960=CARTESIAN_POINT('Ctrl Pts',(152.681760566299,16.075981492637,-3.374587546725));
#25961=CARTESIAN_POINT('Ctrl Pts',(152.642529290804,15.5216175069818,-6.01548663444557));
#25962=CARTESIAN_POINT('Ctrl Pts',(152.60329801531,14.3027656933877,-8.51689984690491));
#25963=CARTESIAN_POINT('Ctrl Pts',(152.564066739816,12.5645675371996,-10.5809576440515));
#25964=CARTESIAN_POINT('Ctrl Pts',(152.524835464321,10.8263693810116,-12.645015441198));
#25965=CARTESIAN_POINT('Ctrl Pts',(152.485604188827,8.56882488222956,-14.2717178230318));
#25966=CARTESIAN_POINT('Ctrl Pts',(152.446372913332,6.06076357217012,-15.2673562539341));
#25967=CARTESIAN_POINT('Ctrl Pts',(152.407141637838,3.55270226211068,-16.2629946848364));
#25968=CARTESIAN_POINT('Ctrl Pts',(152.367910362344,0.794124140773821,-16.6275691648073));
#25969=CARTESIAN_POINT('Ctrl Pts',(152.328679086849,-1.8864779254381,-16.3176659819518));
#25970=CARTESIAN_POINT('Ctrl Pts',(152.289447811355,-4.56707999165003,-16.0077627990964));
#25971=CARTESIAN_POINT('Ctrl Pts',(152.25021653586,-7.16970600273701,-15.0233819534147));
#25972=CARTESIAN_POINT('Ctrl Pts',(152.210985260366,-9.3844339477921,-13.4817440096735));
#25973=CARTESIAN_POINT('Ctrl Pts',(152.171753984872,-11.5991618928472,-11.9401060659323));
#25974=CARTESIAN_POINT('Ctrl Pts',(152.132522709377,-13.4259917718704,-9.84121102413149));
#25975=CARTESIAN_POINT('Ctrl Pts',(152.093291433883,-14.6473837665455,-7.43499635889051));
#25976=CARTESIAN_POINT('Ctrl Pts',(152.055913238306,-15.8110836023985,-5.1424386680136));
#25977=CARTESIAN_POINT('Ctrl Pts',(152.018535042729,-16.4251901751372,-2.5709080237884));
#25978=CARTESIAN_POINT('Ctrl Pts',(151.981156847152,-16.4262658875693,0.000126548556290129));
#25979=CARTESIAN_POINT('Ctrl Pts',(151.768843152848,-16.4263175731226,7.92183299041088E-5));
#25980=CARTESIAN_POINT('Ctrl Pts',(151.806929176476,-16.4256006911727,-2.61961882950725));
#25981=CARTESIAN_POINT('Ctrl Pts',(151.845015200103,-15.7871398110322,-5.23965402112013));
#25982=CARTESIAN_POINT('Ctrl Pts',(151.883101223731,-14.5806721903752,-7.56498651285041));
#25983=CARTESIAN_POINT('Ctrl Pts',(151.922332499225,-13.3379259256609,-9.9602420662013));
#25984=CARTESIAN_POINT('Ctrl Pts',(151.96156377472,-11.4924992427678,-12.042804945796));
#25985=CARTESIAN_POINT('Ctrl Pts',(152.000795050214,-9.26414648165388,-13.5646825352884));
#25986=CARTESIAN_POINT('Ctrl Pts',(152.040026325709,-7.03579372053995,-15.0865601247808));
#25987=CARTESIAN_POINT('Ctrl Pts',(152.079257601203,-4.42451488120518,-16.0477524241709));
#25988=CARTESIAN_POINT('Ctrl Pts',(152.118488876697,-1.74126235529177,-16.3338001645162));
#25989=CARTESIAN_POINT('Ctrl Pts',(152.157720152192,0.941990170621638,-16.6198479048615));
#25990=CARTESIAN_POINT('Ctrl Pts',(152.196951427686,3.69721638311369,-16.230751086162));
#25991=CARTESIAN_POINT('Ctrl Pts',(152.236182703181,6.19632256160219,-15.2128435565597));
#25992=CARTESIAN_POINT('Ctrl Pts',(152.275413978675,8.69542874009068,-14.1949360269574));
#25993=CARTESIAN_POINT('Ctrl Pts',(152.314645254169,10.9384148845756,-12.5482177864524));
#25994=CARTESIAN_POINT('Ctrl Pts',(152.353876529664,12.6581850804413,-10.4687808672768));
#25995=CARTESIAN_POINT('Ctrl Pts',(152.393107805158,14.377955276307,-8.38934394810116));
#25996=CARTESIAN_POINT('Ctrl Pts',(152.432339080653,15.5745095235535,-5.87718835025486));
#25997=CARTESIAN_POINT('Ctrl Pts',(152.471570356147,16.1053615419439,-3.23146282334491));
#25998=CARTESIAN_POINT('Ctrl Pts',(152.510801631641,16.6362135603342,-0.585737296434967));
#25999=CARTESIAN_POINT('Ctrl Pts',(152.550032907136,16.5013633498685,2.19355815953864));
#26000=CARTESIAN_POINT('Ctrl Pts',(152.58926418263,15.7168689413851,4.77546364800653));
#26001=CARTESIAN_POINT('Ctrl Pts',(152.628495458125,14.9323745329016,7.35736913647443));
#26002=CARTESIAN_POINT('Ctrl Pts',(152.667726733619,13.4982359264005,9.74188465743662));
#26003=CARTESIAN_POINT('Ctrl Pts',(152.706958009113,11.5852310664511,11.6450609063546));
#26004=CARTESIAN_POINT('Ctrl Pts',(152.746189284608,9.67222620650168,13.5482371552725));
#26005=CARTESIAN_POINT('Ctrl Pts',(152.785420560102,7.28035509310412,14.9700741321463));
#26006=CARTESIAN_POINT('Ctrl Pts',(152.824651835597,4.69444293825117,15.7412587766719));
#26007=CARTESIAN_POINT('Ctrl Pts',(152.863883111091,2.10853078339819,16.5124434211975));
#26008=CARTESIAN_POINT('Ctrl Pts',(152.903114386585,-0.671422412910195,
16.632975733375));
#26009=CARTESIAN_POINT('Ctrl Pts',(152.94234566208,-3.31437842963123,16.0885026649596));
#26010=CARTESIAN_POINT('Ctrl Pts',(152.981576937574,-5.95733444635227,15.5440295965442));
#26011=CARTESIAN_POINT('Ctrl Pts',(153.020808213068,-8.46329328348596,14.3345511475358));
#26012=CARTESIAN_POINT('Ctrl Pts',(153.060039488563,-10.5338441056942,12.6040926183492));
#26013=CARTESIAN_POINT('Ctrl Pts',(153.099270764057,-12.6043949279025,10.8736340891626));
#26014=CARTESIAN_POINT('Ctrl Pts',(153.138502039552,-14.2395377351854,8.62219547979772));
#26015=CARTESIAN_POINT('Ctrl Pts',(153.177733315046,-15.2445589018574,6.11787922918138));
#26016=CARTESIAN_POINT('Ctrl Pts',(153.20810326098,-16.0225718038015,4.17922319074239));
#26017=CARTESIAN_POINT('Ctrl Pts',(153.238473206914,-16.4229711502018,2.08902494350394));
#26018=CARTESIAN_POINT('Ctrl Pts',(153.268843152848,-16.4250464537185,-0.000400491521010713));
#26019=CARTESIAN_POINT('Origin',(157.6,0.,0.));
#26020=CARTESIAN_POINT('',(154.981156847152,-16.4236977086378,-8.83777446403222E-5));
#26021=CARTESIAN_POINT('',(154.768843152848,-16.4236758302589,-4.56654442711846E-5));
#26022=CARTESIAN_POINT('',(157.6,-16.425,-2.01148236759953E-15));
#26023=CARTESIAN_POINT('Ctrl Pts',(154.981156847152,-16.4236977086378,-8.83777446403222E-5));
#26024=CARTESIAN_POINT('Ctrl Pts',(154.960085654594,-16.4234191421019,1.44993295162065));
#26025=CARTESIAN_POINT('Ctrl Pts',(154.939014462037,-16.233159747019,2.90002600296101));
#26026=CARTESIAN_POINT('Ctrl Pts',(154.917943269479,-15.8538585334443,4.29885934448325));
#26027=CARTESIAN_POINT('Ctrl Pts',(154.878711993985,-15.1476588077049,6.90326894504319));
#26028=CARTESIAN_POINT('Ctrl Pts',(154.839480718491,-13.7861525287593,9.32998863536398));
#26029=CARTESIAN_POINT('Ctrl Pts',(154.800249442996,-11.9314685472444,11.2900434174645));
#26030=CARTESIAN_POINT('Ctrl Pts',(154.761018167502,-10.0767845657294,13.250098199565));
#26031=CARTESIAN_POINT('Ctrl Pts',(154.721786892007,-7.72892288164514,14.7434880734452));
#26032=CARTESIAN_POINT('Ctrl Pts',(154.682555616513,-5.16746804203438,15.5923794238297));
#26033=CARTESIAN_POINT('Ctrl Pts',(154.643324341019,-2.60601320242361,16.4412707742142));
#26034=CARTESIAN_POINT('Ctrl Pts',(154.604093065524,0.169034792713642,16.6456636011031));
#26035=CARTESIAN_POINT('Ctrl Pts',(154.56486179003,2.82722183613503,16.1812187041457));
#26036=CARTESIAN_POINT('Ctrl Pts',(154.525630514535,5.48540887955642,15.7167738071883));
#26037=CARTESIAN_POINT('Ctrl Pts',(154.486399239041,8.02673497126193,14.5834911863846));
#26038=CARTESIAN_POINT('Ctrl Pts',(154.447167963547,10.1485777255062,12.9163227046816));
#26039=CARTESIAN_POINT('Ctrl Pts',(154.407936688052,12.2704204797506,11.2491542229785));
#26040=CARTESIAN_POINT('Ctrl Pts',(154.368705412558,13.9727798965336,9.04809988037614));
#26041=CARTESIAN_POINT('Ctrl Pts',(154.329474137063,15.0529381625909,6.5752623320541));
#26042=CARTESIAN_POINT('Ctrl Pts',(154.290242861569,16.1330964286481,4.10242478373211));
#26043=CARTESIAN_POINT('Ctrl Pts',(154.251011586075,16.5910535439795,1.35780402969045));
#26044=CARTESIAN_POINT('Ctrl Pts',(154.21178031058,16.3722757455772,-1.33176911396061));
#26045=CARTESIAN_POINT('Ctrl Pts',(154.172549035086,16.1534979471749,-4.02134225761174));
#26046=CARTESIAN_POINT('Ctrl Pts',(154.133317759591,15.2579852350389,-6.65586779087229));
#26047=CARTESIAN_POINT('Ctrl Pts',(154.094086484097,13.7923757121252,-8.92162509174716));
#26048=CARTESIAN_POINT('Ctrl Pts',(154.054855208603,12.3267661892115,-11.187382392622));
#26049=CARTESIAN_POINT('Ctrl Pts',(154.015623933108,10.2910598555201,-13.0843714611112));
#26050=CARTESIAN_POINT('Ctrl Pts',(153.976392657614,7.92766964238983,-14.3866978873974));
#26051=CARTESIAN_POINT('Ctrl Pts',(153.937161382119,5.56427942925962,-15.6890243136836));
#26052=CARTESIAN_POINT('Ctrl Pts',(153.897930106625,2.87320533669065,-16.3966880977669));
#26053=CARTESIAN_POINT('Ctrl Pts',(153.858698831131,0.174901817485615,-16.42542028127));
#26054=CARTESIAN_POINT('Ctrl Pts',(153.819467555636,-2.52340170171938,-16.454152464773));
#26055=CARTESIAN_POINT('Ctrl Pts',(153.780236280142,-5.22893464756042,-15.803953047696));
#26056=CARTESIAN_POINT('Ctrl Pts',(153.741005004647,-7.61952079973456,-14.5522481027684));
#26057=CARTESIAN_POINT('Ctrl Pts',(153.701773729153,-10.0101069519087,-13.3005431578408));
#26058=CARTESIAN_POINT('Ctrl Pts',(153.662542453659,-12.0857463104159,-11.4473326850627));
#26059=CARTESIAN_POINT('Ctrl Pts',(153.623311178164,-13.5992706992915,-9.21329791711442));
#26060=CARTESIAN_POINT('Ctrl Pts',(153.58407990267,-15.1127950881672,-6.97926314916609));
#26061=CARTESIAN_POINT('Ctrl Pts',(153.544848627175,-16.0642045074111,-4.36440408604759));
#26062=CARTESIAN_POINT('Ctrl Pts',(153.505617351681,-16.340204646147,-1.68009945662473));
#26063=CARTESIAN_POINT('Ctrl Pts',(153.497463850171,-16.3975662159535,-1.12221594218909));
#26064=CARTESIAN_POINT('Ctrl Pts',(153.489310348662,-16.4257541551807,-0.561332795744825));
#26065=CARTESIAN_POINT('Ctrl Pts',(153.481156847152,-16.4251954303659,-0.000393763598601771));
#26066=CARTESIAN_POINT('Ctrl Pts',(153.268843152848,-16.4250464537185,-0.000400491521010713));
#26067=CARTESIAN_POINT('Ctrl Pts',(153.277704482409,-16.4256519848721,-0.610052132384859));
#26068=CARTESIAN_POINT('Ctrl Pts',(153.286565811969,-16.3923460737495,-1.21963797963861));
#26069=CARTESIAN_POINT('Ctrl Pts',(153.295427141529,-16.324614256424,-1.8253744147469));
#26070=CARTESIAN_POINT('Ctrl Pts',(153.334658417024,-16.0247489182573,-4.50711791619102));
#26071=CARTESIAN_POINT('Ctrl Pts',(153.373889692518,-15.0501187158627,-7.11341102721143));
#26072=CARTESIAN_POINT('Ctrl Pts',(153.413120968012,-13.5167831026228,-9.3338950568178));
#26073=CARTESIAN_POINT('Ctrl Pts',(153.452352243507,-11.9834474893829,-11.5543790864242));
#26074=CARTESIAN_POINT('Ctrl Pts',(153.491583519001,-9.89140646529765,-13.3890540346165));
#26075=CARTESIAN_POINT('Ctrl Pts',(153.530814794496,-7.48978132489561,-14.6194458882782));
#26076=CARTESIAN_POINT('Ctrl Pts',(153.57004606999,-5.08815618449357,-15.84983774194));
#26077=CARTESIAN_POINT('Ctrl Pts',(153.609277345484,-2.37694692777465,-16.4759465010711));
#26078=CARTESIAN_POINT('Ctrl Pts',(153.648508620979,0.32099428701121,-16.4232148205748));
#26079=CARTESIAN_POINT('Ctrl Pts',(153.687739896473,3.01893550179707,-16.3704831400786));
#26080=CARTESIAN_POINT('Ctrl Pts',(153.726971171968,5.70360867464991,-15.6389110199551));
#26081=CARTESIAN_POINT('Ctrl Pts',(153.766202447462,8.05532157749775,-14.3156144352293));
#26082=CARTESIAN_POINT('Ctrl Pts',(153.805433722957,10.4070344803456,-12.9923178505035));
#26083=CARTESIAN_POINT('Ctrl Pts',(153.844664998451,12.4257871131884,-11.0772968011756));
#26084=CARTESIAN_POINT('Ctrl Pts',(153.883896273945,13.8711853998883,-8.79859295438607));
#26085=CARTESIAN_POINT('Ctrl Pts',(153.92312754944,15.3165836865881,-6.51988910759658));
#26086=CARTESIAN_POINT('Ctrl Pts',(153.962358824934,16.188627627145,-3.87750246334555));
#26087=CARTESIAN_POINT('Ctrl Pts',(154.001590100428,16.3834737916948,-1.18608974866797));
#26088=CARTESIAN_POINT('Ctrl Pts',(154.040821375923,16.5783199562446,1.50532296600961));
#26089=CARTESIAN_POINT('Ctrl Pts',(154.080052651417,16.0959683447872,4.24576175111375));
#26090=CARTESIAN_POINT('Ctrl Pts',(154.119283926912,14.9938576291657,6.70889378149298));
#26091=CARTESIAN_POINT('Ctrl Pts',(154.158515202406,13.8917469135441,9.17202581187224));
#26092=CARTESIAN_POINT('Ctrl Pts',(154.1977464779,12.1698770937584,11.3578510875266));
#26093=CARTESIAN_POINT('Ctrl Pts',(154.236977753395,10.0332892916491,13.0060804382075));
#26094=CARTESIAN_POINT('Ctrl Pts',(154.276209028889,7.89670148953989,14.6543097888884));
#26095=CARTESIAN_POINT('Ctrl Pts',(154.315440304384,5.34539570510719,15.764943214596));
#26096=CARTESIAN_POINT('Ctrl Pts',(154.354671579878,2.6831827109122,16.2057259298961));
#26097=CARTESIAN_POINT('Ctrl Pts',(154.393902855372,0.0209697167172235,
16.6465086451963));
#26098=CARTESIAN_POINT('Ctrl Pts',(154.433134130867,-2.75215048724,16.4174406500891));
#26099=CARTESIAN_POINT('Ctrl Pts',(154.472365406361,-5.30595335605791,15.5457994763339));
#26100=CARTESIAN_POINT('Ctrl Pts',(154.511596681856,-7.85975622487584,14.6741583025787));
#26101=CARTESIAN_POINT('Ctrl Pts',(154.55082795735,-10.1942417585544,13.1599439501754));
#26102=CARTESIAN_POINT('Ctrl Pts',(154.590059232844,-12.0314182487506,11.1834698237477));
#26103=CARTESIAN_POINT('Ctrl Pts',(154.629290508339,-13.8685947389469,9.20699569731996));
#26104=CARTESIAN_POINT('Ctrl Pts',(154.668521783833,-15.2084621856608,6.76826179686773));
#26105=CARTESIAN_POINT('Ctrl Pts',(154.707753059328,-15.8914685012518,4.15767377854104));
#26106=CARTESIAN_POINT('Ctrl Pts',(154.728116423834,-16.2459893877024,2.80262338253725));
#26107=CARTESIAN_POINT('Ctrl Pts',(154.748479788341,-16.4235369624548,1.40127158289091));
#26108=CARTESIAN_POINT('Ctrl Pts',(154.768843152848,-16.4236758302589,-4.56654442711846E-5));
#26109=CARTESIAN_POINT('Origin',(157.6,0.,0.));
#26110=CARTESIAN_POINT('',(156.481156847152,-16.4245975118847,0.000389008950720526));
#26111=CARTESIAN_POINT('',(156.268843152848,-16.4247375848135,0.000397937037689734));
#26112=CARTESIAN_POINT('',(157.6,-16.425,-2.01148236759953E-15));
#26113=CARTESIAN_POINT('Ctrl Pts',(156.481156847152,-16.4245975118847,0.000389008950720526));
#26114=CARTESIAN_POINT('Ctrl Pts',(156.470092236022,-16.4252950978913,0.761684348249804));
#26115=CARTESIAN_POINT('Ctrl Pts',(156.459027624891,-16.3733031429826,1.52288516962114));
#26116=CARTESIAN_POINT('Ctrl Pts',(156.447963013761,-16.2678244069857,2.27660078309594));
#26117=CARTESIAN_POINT('Ctrl Pts',(156.408731738266,-15.893833373596,4.94901507116341));
#26118=CARTESIAN_POINT('Ctrl Pts',(156.369500462772,-14.8474248389515,7.52732788803067));
#26119=CARTESIAN_POINT('Ctrl Pts',(156.330269187278,-13.2532056562426,9.70451245016734));
#26120=CARTESIAN_POINT('Ctrl Pts',(156.291037911783,-11.6589864735338,11.881697012304));
#26121=CARTESIAN_POINT('Ctrl Pts',(156.251806636289,-9.51695664276062,13.6577533197101));
#26122=CARTESIAN_POINT('Ctrl Pts',(156.212575360794,-7.08219015062719,14.8211876964187));
#26123=CARTESIAN_POINT('Ctrl Pts',(156.1733440853,-4.64742365849377,15.9846220731273));
#26124=CARTESIAN_POINT('Ctrl Pts',(156.134112809806,-1.91992050500006,16.5354345191385));
#26125=CARTESIAN_POINT('Ctrl Pts',(156.094881534311,0.775526866203273,16.4080340120903));
#26126=CARTESIAN_POINT('Ctrl Pts',(156.055650258817,3.4709742374066,16.280633505042));
#26127=CARTESIAN_POINT('Ctrl Pts',(156.016418983322,6.13436582631956,15.4750200449344));
#26128=CARTESIAN_POINT('Ctrl Pts',(155.977187707828,8.44854362656052,14.0871264866976));
#26129=CARTESIAN_POINT('Ctrl Pts',(155.937956432334,10.7627214268014,12.6992329284609));
#26130=CARTESIAN_POINT('Ctrl Pts',(155.898725156839,12.7276854383704,10.7290592720952));
#26131=CARTESIAN_POINT('Ctrl Pts',(155.859493881345,14.1094467611315,8.41121478485182));
#26132=CARTESIAN_POINT('Ctrl Pts',(155.82026260585,15.4912080838927,6.09337029760841));
#26133=CARTESIAN_POINT('Ctrl Pts',(155.781031330356,16.2897667178459,3.42785497948738));
#26134=CARTESIAN_POINT('Ctrl Pts',(155.741800054862,16.4100299002982,0.73207973160974));
#26135=CARTESIAN_POINT('Ctrl Pts',(155.702568779367,16.5302930827504,-1.96369551626784));
#26136=CARTESIAN_POINT('Ctrl Pts',(155.663337503873,15.9722608137017,-4.689730693902));
#26137=CARTESIAN_POINT('Ctrl Pts',(155.624106228379,14.8023838556628,-7.12140816494386));
#26138=CARTESIAN_POINT('Ctrl Pts',(155.584874952884,13.6325068976238,-9.5530856359857));
#26139=CARTESIAN_POINT('Ctrl Pts',(155.54564367739,11.8507852505947,-11.6904054004352));
#26140=CARTESIAN_POINT('Ctrl Pts',(155.506412401895,9.66938722202629,-13.2788543486488));
#26141=CARTESIAN_POINT('Ctrl Pts',(155.467181126401,7.48798919345788,-14.8673032968624));
#26142=CARTESIAN_POINT('Ctrl Pts',(155.427949850907,4.90691478335018,-15.9068814288401));
#26143=CARTESIAN_POINT('Ctrl Pts',(155.388718575412,2.23351962714189,-16.273795259167));
#26144=CARTESIAN_POINT('Ctrl Pts',(155.349487299918,-0.439875529066391,
-16.6407090894939));
#26145=CARTESIAN_POINT('Ctrl Pts',(155.310256024423,-3.20559143137527,-16.3349586181701));
#26146=CARTESIAN_POINT('Ctrl Pts',(155.271024748929,-5.73428524283742,-15.3929527646872));
#26147=CARTESIAN_POINT('Ctrl Pts',(155.231793473434,-8.26297905429957,-14.4509469112043));
#26148=CARTESIAN_POINT('Ctrl Pts',(155.19256219794,-10.554650774915,-12.8726856755622));
#26149=CARTESIAN_POINT('Ctrl Pts',(155.153330922446,-12.336406986676,-10.8461091973669));
#26150=CARTESIAN_POINT('Ctrl Pts',(155.114099646951,-14.1181631984369,-8.81953271917163));
#26151=CARTESIAN_POINT('Ctrl Pts',(155.074868371457,-15.3900039013434,-6.34464099842317));
#26152=CARTESIAN_POINT('Ctrl Pts',(155.035637095963,-16.0004776665301,-3.71614538264941));
#26153=CARTESIAN_POINT('Ctrl Pts',(155.017477013026,-16.2830648133123,-2.49941975290202));
#26154=CARTESIAN_POINT('Ctrl Pts',(154.999316930089,-16.4239377895627,-1.24978070197727));
#26155=CARTESIAN_POINT('Ctrl Pts',(154.981156847152,-16.4236977086378,-8.83777446403222E-5));
#26156=CARTESIAN_POINT('Ctrl Pts',(154.768843152848,-16.4236758302589,-4.56654442711846E-5));
#26157=CARTESIAN_POINT('Ctrl Pts',(154.787711063836,-16.4238044998294,-1.29845237510138));
#26158=CARTESIAN_POINT('Ctrl Pts',(154.806578974823,-16.2716248951007,-2.59682942189317));
#26159=CARTESIAN_POINT('Ctrl Pts',(154.825446885811,-15.966790672975,-3.85831802479324));
#26160=CARTESIAN_POINT('Ctrl Pts',(154.864678161305,-15.3329613446391,-6.48127967359964));
#26161=CARTESIAN_POINT('Ctrl Pts',(154.903909436799,-14.0391575034993,-8.9447608350113));
#26162=CARTESIAN_POINT('Ctrl Pts',(154.943140712294,-12.2394459599386,-10.9554089366298));
#26163=CARTESIAN_POINT('Ctrl Pts',(154.982371987788,-10.4397344163778,-12.9660570382483));
#26164=CARTESIAN_POINT('Ctrl Pts',(155.021603263283,-8.13411517039618,-14.5238720800737));
#26165=CARTESIAN_POINT('Ctrl Pts',(155.060834538777,-5.59714251831809,-15.4433486655156));
#26166=CARTESIAN_POINT('Ctrl Pts',(155.100065814272,-3.06016986623997,-16.3628252509574));
#26167=CARTESIAN_POINT('Ctrl Pts',(155.139297089766,-0.291843808065398,
-16.6439633800158));
#26168=CARTESIAN_POINT('Ctrl Pts',(155.17852836526,2.37818200058848,-16.2532849832618));
#26169=CARTESIAN_POINT('Ctrl Pts',(155.217759640755,5.04820780924235,-15.8626065865077));
#26170=CARTESIAN_POINT('Ctrl Pts',(155.256990916249,7.61993336837555,-14.8001116639413));
#26171=CARTESIAN_POINT('Ctrl Pts',(155.296222191744,9.78711630841292,-13.1923226438957));
#26172=CARTESIAN_POINT('Ctrl Pts',(155.335453467238,11.9542992484503,-11.5845336238501));
#26173=CARTESIAN_POINT('Ctrl Pts',(155.374684742732,13.7169395693918,-9.43145050632542));
#26174=CARTESIAN_POINT('Ctrl Pts',(155.413916018227,14.8651411776684,-6.98946350895643));
#26175=CARTESIAN_POINT('Ctrl Pts',(155.453147293721,16.0133427859449,-4.54747651158745));
#26176=CARTESIAN_POINT('Ctrl Pts',(155.492378569216,16.5471056815565,-1.81658563437417));
#26177=CARTESIAN_POINT('Ctrl Pts',(155.53160984471,16.4028691111549,0.878013267192959));
#26178=CARTESIAN_POINT('Ctrl Pts',(155.570841120204,16.2586325407533,3.57261216876009));
#26179=CARTESIAN_POINT('Ctrl Pts',(155.610072395699,15.4363965043385,6.23091909468103));
#26180=CARTESIAN_POINT('Ctrl Pts',(155.649303671193,14.0340732815655,8.53638152279379));
#26181=CARTESIAN_POINT('Ctrl Pts',(155.688534946687,12.6317500587925,10.8418439509066));
#26182=CARTESIAN_POINT('Ctrl Pts',(155.727766222182,10.6493396496614,12.7944618812111));
#26183=CARTESIAN_POINT('Ctrl Pts',(155.766997497676,8.32290848008079,14.1617165911215));
#26184=CARTESIAN_POINT('Ctrl Pts',(155.806228773171,5.99647731050022,15.5289713010318));
#26185=CARTESIAN_POINT('Ctrl Pts',(155.845460048665,3.32602538047026,16.3108627905479));
#26186=CARTESIAN_POINT('Ctrl Pts',(155.884691324159,0.629551445334231,16.4142830288966));
#26187=CARTESIAN_POINT('Ctrl Pts',(155.923922599654,-2.0669224898018,16.5177032672453));
#26188=CARTESIAN_POINT('Ctrl Pts',(155.963153875148,-4.78941843004388,15.9426522544265));
#26189=CARTESIAN_POINT('Ctrl Pts',(156.002385150643,-7.21374019320702,14.7576073534959));
#26190=CARTESIAN_POINT('Ctrl Pts',(156.041616426137,-9.63806195637014,13.5725624525653));
#26191=CARTESIAN_POINT('Ctrl Pts',(156.080847701631,-11.7642095424543,11.7775236635228));
#26192=CARTESIAN_POINT('Ctrl Pts',(156.120078977126,-13.3390002304198,9.5862451057704));
#26193=CARTESIAN_POINT('Ctrl Pts',(156.15931025262,-14.9137909183852,7.39496654801799));
#26194=CARTESIAN_POINT('Ctrl Pts',(156.198541528115,-15.9372247082318,4.80744822155563));
#26195=CARTESIAN_POINT('Ctrl Pts',(156.237772803609,-16.287430590904,2.13181310661377));
#26196=CARTESIAN_POINT('Ctrl Pts',(156.248129586689,-16.3798825011303,1.42546409968821));
#26197=CARTESIAN_POINT('Ctrl Pts',(156.258486369768,-16.425415598584,0.712974029600022));
#26198=CARTESIAN_POINT('Ctrl Pts',(156.268843152848,-16.4247375848135,0.000397937037689734));
#26199=CARTESIAN_POINT('Origin',(157.6,0.,0.));
#26200=CARTESIAN_POINT('',(157.981156847152,-16.4263224034013,7.32633077222405E-5));
#26201=CARTESIAN_POINT('',(157.768843152848,-16.4263481654919,2.43998567653511E-5));
#26202=CARTESIAN_POINT('',(157.6,-16.425,-2.01148236759953E-15));
#26203=CARTESIAN_POINT('Ctrl Pts',(157.981156847152,-16.4263224034013,7.32633077222405E-5));
#26204=CARTESIAN_POINT('Ctrl Pts',(157.980098817449,-16.4263409280204,0.0728484104607535));
#26205=CARTESIAN_POINT('Ctrl Pts',(157.979040787745,-16.4258671636985,0.145623315585142));
#26206=CARTESIAN_POINT('Ctrl Pts',(157.977982758042,-16.4248996084331,0.218391655079058));
#26207=CARTESIAN_POINT('Ctrl Pts',(157.938751482548,-16.389023085253,2.91660964019587));
#26208=CARTESIAN_POINT('Ctrl Pts',(157.899520207053,-15.6742364830876,5.60580058104853));
#26209=CARTESIAN_POINT('Ctrl Pts',(157.860288931559,-14.3656569490643,7.96573427148533));
#26210=CARTESIAN_POINT('Ctrl Pts',(157.821057656065,-13.057077415041,10.3256679619221));
#26211=CARTESIAN_POINT('Ctrl Pts',(157.78182638057,-11.1547049491598,12.356344401943));
#26212=CARTESIAN_POINT('Ctrl Pts',(157.742595105076,-8.88507501889968,13.8159496224704));
#26213=CARTESIAN_POINT('Ctrl Pts',(157.703363829582,-6.61544508863964,15.2755548429977));
#26214=CARTESIAN_POINT('Ctrl Pts',(157.664132554087,-3.97855769400073,16.1640888440315));
#26215=CARTESIAN_POINT('Ctrl Pts',(157.624901278593,-1.28841470861576,16.3757445510345));
#26216=CARTESIAN_POINT('Ctrl Pts',(157.585670003098,1.40172827676925,16.5874002580375));
#26217=CARTESIAN_POINT('Ctrl Pts',(157.546438727604,4.14512685290032,16.1221776710096));
#26218=CARTESIAN_POINT('Ctrl Pts',(157.50720745211,6.61509574122592,15.0354757289728));
#26219=CARTESIAN_POINT('Ctrl Pts',(157.467976176615,9.08506462955151,13.9487737869359));
#26220=CARTESIAN_POINT('Ctrl Pts',(157.428744901121,11.2816038300716,12.24059248989));
#26221=CARTESIAN_POINT('Ctrl Pts',(157.389513625626,12.9431483529905,10.1143429235217));
#26222=CARTESIAN_POINT('Ctrl Pts',(157.350282350132,14.6046928759094,7.98809335715339));
#26223=CARTESIAN_POINT('Ctrl Pts',(157.311051074638,15.7312427212271,5.44377552146273));
#26224=CARTESIAN_POINT('Ctrl Pts',(157.271819799143,16.1886477682787,2.78436806056945));
#26225=CARTESIAN_POINT('Ctrl Pts',(157.232588523649,16.6460528153303,0.124960599676174));
#26226=CARTESIAN_POINT('Ctrl Pts',(157.193357248154,16.4343130641158,-2.64953648641971));
#26227=CARTESIAN_POINT('Ctrl Pts',(157.15412597266,15.5786425904199,-5.20873469300084));
#26228=CARTESIAN_POINT('Ctrl Pts',(157.114894697166,14.7229721167239,-7.76793289958189));
#26229=CARTESIAN_POINT('Ctrl Pts',(157.075663421671,13.2233709205465,-10.1118322266482));
#26230=CARTESIAN_POINT('Ctrl Pts',(157.036432146177,11.2584122645379,-11.9613199666181));
#26231=CARTESIAN_POINT('Ctrl Pts',(156.997200870682,9.29345360852907,-13.8108077065882));
#26232=CARTESIAN_POINT('Ctrl Pts',(156.957969595188,6.86313749268894,-15.1658838594618));
#26233=CARTESIAN_POINT('Ctrl Pts',(156.918738319694,4.25686717915344,-15.8651852772402));
#26234=CARTESIAN_POINT('Ctrl Pts',(156.879507044199,1.65059686561801,-16.5644866950186));
#26235=CARTESIAN_POINT('Ctrl Pts',(156.840275768705,-1.13162764561276,-16.6080133777018));
#26236=CARTESIAN_POINT('Ctrl Pts',(156.80104449321,-3.75849766416033,-15.9905821460826));
#26237=CARTESIAN_POINT('Ctrl Pts',(156.761813217716,-6.38536768270793,-15.3731509144634));
#26238=CARTESIAN_POINT('Ctrl Pts',(156.722581942222,-8.85688320857233,-14.0947617685418));
#26239=CARTESIAN_POINT('Ctrl Pts',(156.683350666727,-10.8787349332059,-12.3076459290621));
#26240=CARTESIAN_POINT('Ctrl Pts',(156.644119391233,-12.9005866578396,-10.5205300895824));
#26241=CARTESIAN_POINT('Ctrl Pts',(156.604888115738,-14.4727745812424,-8.22468755654467));
#26242=CARTESIAN_POINT('Ctrl Pts',(156.565656840244,-15.4080817768764,-5.69350841039195));
#26243=CARTESIAN_POINT('Ctrl Pts',(156.53749017588,-16.0795991701985,-3.87621155841627));
#26244=CARTESIAN_POINT('Ctrl Pts',(156.509323511516,-16.4228216997318,-1.93760502006057));
#26245=CARTESIAN_POINT('Ctrl Pts',(156.481156847152,-16.4245975118847,0.000389008950720526));
#26246=CARTESIAN_POINT('Ctrl Pts',(156.268843152848,-16.4247375848135,0.000397937037689734));
#26247=CARTESIAN_POINT('Ctrl Pts',(156.297717645263,-16.4228472967459,-1.98624915417195));
#26248=CARTESIAN_POINT('Ctrl Pts',(156.326592137678,-16.0617660728888,-3.97356488312194));
#26249=CARTESIAN_POINT('Ctrl Pts',(156.355466630092,-15.3568301421047,-5.83033364067544));
#26250=CARTESIAN_POINT('Ctrl Pts',(156.394697905587,-14.3990458351355,-8.35309336960156));
#26251=CARTESIAN_POINT('Ctrl Pts',(156.433929181081,-12.8064992456994,-10.6348609240325));
#26252=CARTESIAN_POINT('Ctrl Pts',(156.473160456575,-10.7688316204978,-12.4039222790379));
#26253=CARTESIAN_POINT('Ctrl Pts',(156.51239173207,-8.73116399529622,-14.1729836340432));
#26254=CARTESIAN_POINT('Ctrl Pts',(156.551623007564,-6.24837533432913,-15.4293387896229));
#26255=CARTESIAN_POINT('Ctrl Pts',(156.590854283059,-3.61611735672674,-16.0233803436549));
#26256=CARTESIAN_POINT('Ctrl Pts',(156.630085558553,-0.983859379124374,
-16.6174218976868));
#26257=CARTESIAN_POINT('Ctrl Pts',(156.669316834047,1.79786791511326,-16.5491498501711));
#26258=CARTESIAN_POINT('Ctrl Pts',(156.708548109542,4.39781504445652,-15.8266940707716));
#26259=CARTESIAN_POINT('Ctrl Pts',(156.747779385036,6.99776217379977,-15.1042382913721));
#26260=CARTESIAN_POINT('Ctrl Pts',(156.787010660531,9.41592913824868,-13.7275987800887));
#26261=CARTESIAN_POINT('Ctrl Pts',(156.826241936025,11.364359402709,-11.8607064604561));
#26262=CARTESIAN_POINT('Ctrl Pts',(156.865473211519,13.3127896671693,-9.99381414082351));
#26263=CARTESIAN_POINT('Ctrl Pts',(156.904704487014,14.791483231641,-7.63666901284167));
#26264=CARTESIAN_POINT('Ctrl Pts',(156.943935762508,15.6243565247449,-5.06996110070942));
#26265=CARTESIAN_POINT('Ctrl Pts',(156.983167038003,16.4572298178488,-2.50325318857716));
#26266=CARTESIAN_POINT('Ctrl Pts',(157.022398313497,16.6442828395849,0.27301750770553));
#26267=CARTESIAN_POINT('Ctrl Pts',(157.061629588991,16.1632412222978,2.92825128103057));
#26268=CARTESIAN_POINT('Ctrl Pts',(157.100860864486,15.6821996050108,5.58348505435563));
#26269=CARTESIAN_POINT('Ctrl Pts',(157.14009213998,14.5330633487007,8.11768190472299));
#26270=CARTESIAN_POINT('Ctrl Pts',(157.179323415474,12.8526721751827,10.229068400022));
#26271=CARTESIAN_POINT('Ctrl Pts',(157.218554690969,11.1722810016648,12.3404548953211));
#26272=CARTESIAN_POINT('Ctrl Pts',(157.257785966463,8.96063491093908,14.0290310355517));
#26273=CARTESIAN_POINT('Ctrl Pts',(157.297017241958,6.48109782886473,15.093720326935));
#26274=CARTESIAN_POINT('Ctrl Pts',(157.336248517452,4.00156074679037,16.1584096183183));
#26275=CARTESIAN_POINT('Ctrl Pts',(157.375479792946,1.25413267336734,16.5992120608542));
#26276=CARTESIAN_POINT('Ctrl Pts',(157.414711068441,-1.43402127829404,16.3636366785762));
#26277=CARTESIAN_POINT('Ctrl Pts',(157.453942343935,-4.12217522995539,16.1280612962983));
#26278=CARTESIAN_POINT('Ctrl Pts',(157.49317361943,-6.75105505985506,15.2161080892066));
#26279=CARTESIAN_POINT('Ctrl Pts',(157.532404894924,-9.00761243918612,13.736372902643));
#26280=CARTESIAN_POINT('Ctrl Pts',(157.571636170419,-11.2641698185172,12.2566377160794));
#26281=CARTESIAN_POINT('Ctrl Pts',(157.610867445913,-13.1484047472796,10.2091205500439));
#26282=CARTESIAN_POINT('Ctrl Pts',(157.650098721407,-14.4359415850123,7.83764077571543));
#26283=CARTESIAN_POINT('Ctrl Pts',(157.689329996902,-15.7234784227451,5.46616100138692));
#26284=CARTESIAN_POINT('Ctrl Pts',(157.728561272396,-16.4143171694482,2.77071861876541));
#26285=CARTESIAN_POINT('Ctrl Pts',(157.76779254789,-16.4261924006351,0.0722882588242302));
#26286=CARTESIAN_POINT('Ctrl Pts',(157.768142749543,-16.4262984059977,0.0482004676566812));
#26287=CARTESIAN_POINT('Ctrl Pts',(157.768492951196,-16.4263503087819,0.0241124383949297));
#26288=CARTESIAN_POINT('Ctrl Pts',(157.768843152848,-16.4263481654919,2.43998567653511E-5));
#26289=CARTESIAN_POINT('Origin',(157.6,0.,0.));
#26290=CARTESIAN_POINT('',(159.481156847152,-16.4250281341261,-0.000400964822849792));
#26291=CARTESIAN_POINT('',(159.268843152848,-16.4248806122125,-0.000401937761208326));
#26292=CARTESIAN_POINT('',(157.6,-16.425,-2.01148236759953E-15));
#26293=CARTESIAN_POINT('Ctrl Pts',(159.481156847152,-16.4250281341261,-0.000400964822849792));
#26294=CARTESIAN_POINT('Ctrl Pts',(159.450874123381,-16.4229611439312,2.08303035180522));
#26295=CARTESIAN_POINT('Ctrl Pts',(159.420591399611,-16.0249145329238,4.16722913013917));
#26296=CARTESIAN_POINT('Ctrl Pts',(159.390308675841,-15.2512553341834,6.10116651089424));
#26297=CARTESIAN_POINT('Ctrl Pts',(159.351077400346,-14.2489796672177,8.60658282510862));
#26298=CARTESIAN_POINT('Ctrl Pts',(159.311846124852,-12.6163055679695,10.8598123049093));
#26299=CARTESIAN_POINT('Ctrl Pts',(159.272614849357,-10.5476526871368,12.5925392536077));
#26300=CARTESIAN_POINT('Ctrl Pts',(159.233383573863,-8.47899980630407,14.3252662023061));
#26301=CARTESIAN_POINT('Ctrl Pts',(159.194152298369,-5.97436814388689,15.5374906199021));
#26302=CARTESIAN_POINT('Ctrl Pts',(159.154921022874,-3.33201049458475,16.0848602146892));
#26303=CARTESIAN_POINT('Ctrl Pts',(159.11568974738,-0.689652845282527,16.6322298094763));
#26304=CARTESIAN_POINT('Ctrl Pts',(159.076458471885,2.09043079090466,16.5147445814543));
#26305=CARTESIAN_POINT('Ctrl Pts',(159.037227196391,4.67718666007232,15.7463947305075));
#26306=CARTESIAN_POINT('Ctrl Pts',(158.997995920897,7.26394252923991,14.9780448795608));
#26307=CARTESIAN_POINT('Ctrl Pts',(158.958764645402,9.65737063138799,13.5588304056892));
#26308=CARTESIAN_POINT('Ctrl Pts',(158.919533369908,11.5724603475543,11.6577520803283));
#26309=CARTESIAN_POINT('Ctrl Pts',(158.880302094413,13.4875500637206,9.75667375496737));
#26310=CARTESIAN_POINT('Ctrl Pts',(158.841070818919,14.924301393905,7.37373157811711));
#26311=CARTESIAN_POINT('Ctrl Pts',(158.801839543425,15.7116252690259,4.79268749949553));
#26312=CARTESIAN_POINT('Ctrl Pts',(158.76260826793,16.4989491441468,2.21164342087391));
#26313=CARTESIAN_POINT('Ctrl Pts',(158.723376992436,16.6368455642041,-0.567502559519045));
#26314=CARTESIAN_POINT('Ctrl Pts',(158.684145716941,16.1088937543276,-3.21380834430115));
#26315=CARTESIAN_POINT('Ctrl Pts',(158.644914441447,15.5809419444511,-5.86011412908327));
#26316=CARTESIAN_POINT('Ctrl Pts',(158.605683165953,14.3871419046409,-8.37357971825453));
#26317=CARTESIAN_POINT('Ctrl Pts',(158.566451890458,12.6696519424551,-10.4549003686864));
#26318=CARTESIAN_POINT('Ctrl Pts',(158.527220614964,10.9521619802693,-12.5362210191182));
#26319=CARTESIAN_POINT('Ctrl Pts',(158.487989339469,8.71098209570786,-14.1853967308107));
#26320=CARTESIAN_POINT('Ctrl Pts',(158.448758063975,6.21299311361428,-15.2060428327785));
#26321=CARTESIAN_POINT('Ctrl Pts',(158.409526788481,3.71500413152066,-16.2266889347464));
#26322=CARTESIAN_POINT('Ctrl Pts',(158.370295512986,0.960206051894863,-16.6188054269897));
#26323=CARTESIAN_POINT('Ctrl Pts',(158.331064237492,-1.72335838811734,-16.3356988809239));
#26324=CARTESIAN_POINT('Ctrl Pts',(158.291832961997,-4.40692282812948,-16.0525923348582));
#26325=CARTESIAN_POINT('Ctrl Pts',(158.252601686503,-7.01925362852802,-15.0942627504835));
#26326=CARTESIAN_POINT('Ctrl Pts',(158.213370411009,-9.24927312724007,-13.5748284954112));
#26327=CARTESIAN_POINT('Ctrl Pts',(158.174139135514,-11.4792926259521,-12.055394240339));
#26328=CARTESIAN_POINT('Ctrl Pts',(158.13490786002,-13.3270008229777,-9.97485531456915));
#26329=CARTESIAN_POINT('Ctrl Pts',(158.095676584525,-14.572371699393,-7.58096333699378));
#26330=CARTESIAN_POINT('Ctrl Pts',(158.057503338734,-15.7841561231085,-5.25163231968812));
#26331=CARTESIAN_POINT('Ctrl Pts',(158.019330092943,-16.4256540432978,-2.62562199965823));
#26332=CARTESIAN_POINT('Ctrl Pts',(157.981156847152,-16.4263224034013,7.32633077222405E-5));
#26333=CARTESIAN_POINT('Ctrl Pts',(157.768843152848,-16.4263481654919,2.43998567653511E-5));
#26334=CARTESIAN_POINT('Ctrl Pts',(157.80772422669,-16.4261102071114,-2.67434563319392));
#26335=CARTESIAN_POINT('Ctrl Pts',(157.846605300532,-15.7596727937856,-5.34883001203914));
#26336=CARTESIAN_POINT('Ctrl Pts',(157.885486374374,-14.5043647551611,-7.71028050230903));
#26337=CARTESIAN_POINT('Ctrl Pts',(157.924717649868,-13.2377501628293,-10.0930005662402));
#26338=CARTESIAN_POINT('Ctrl Pts',(157.963948925363,-11.371609262495,-12.1570223568418));
#26339=CARTESIAN_POINT('Ctrl Pts',(158.003180200857,-9.1281630486379,-13.6565611239626));
#26340=CARTESIAN_POINT('Ctrl Pts',(158.042411476351,-6.88471683478079,-15.1560998910834));
#26341=CARTESIAN_POINT('Ctrl Pts',(158.081642751846,-4.26396530740087,-16.0911556347235));
#26342=CARTESIAN_POINT('Ctrl Pts',(158.12087402734,-1.57798887296388,-16.3503814479005));
#26343=CARTESIAN_POINT('Ctrl Pts',(158.160105302834,1.10798756147311,-16.6096072610774));
#26344=CARTESIAN_POINT('Ctrl Pts',(158.199336578329,3.85918890296716,-16.1930031437911));
#26345=CARTESIAN_POINT('Ctrl Pts',(158.238567853823,6.34800071575338,-15.1501785232993));
#26346=CARTESIAN_POINT('Ctrl Pts',(158.277799129318,8.8368125285396,-14.1073539028075));
#26347=CARTESIAN_POINT('Ctrl Pts',(158.317030404812,11.063234812618,-12.4383087791102));
#26348=CARTESIAN_POINT('Ctrl Pts',(158.356261680306,12.7621440856132,-10.3417938827408));
#26349=CARTESIAN_POINT('Ctrl Pts',(158.395492955801,14.4610533586083,-8.24527898637131));
#26350=CARTESIAN_POINT('Ctrl Pts',(158.434724231295,15.6324496205203,-5.72129431732967));
#26351=CARTESIAN_POINT('Ctrl Pts',(158.47395550679,16.1368424169009,-3.07039723605181));
#26352=CARTESIAN_POINT('Ctrl Pts',(158.513186782284,16.6412352132814,-0.419500154773992));
#26353=CARTESIAN_POINT('Ctrl Pts',(158.552418057778,16.4786245441306,2.35830933874003));
#26354=CARTESIAN_POINT('Ctrl Pts',(158.591649333273,15.6683741694975,4.93224829663603));
#26355=CARTESIAN_POINT('Ctrl Pts',(158.630880608767,14.8581237948644,7.50618725453202));
#26356=CARTESIAN_POINT('Ctrl Pts',(158.670111884262,13.4002337147489,9.87625567680998));
#26357=CARTESIAN_POINT('Ctrl Pts',(158.709343159756,11.4683102111779,11.7602246269039));
#26358=CARTESIAN_POINT('Ctrl Pts',(158.74857443525,9.53638670760697,13.6441935769979));
#26359=CARTESIAN_POINT('Ctrl Pts',(158.787805710745,7.13042978058057,15.0420630549078));
#26360=CARTESIAN_POINT('Ctrl Pts',(158.827036986239,4.53694198781206,15.7873740620242));
#26361=CARTESIAN_POINT('Ctrl Pts',(158.866268261733,1.94345419504354,16.5326850691405));
#26362=CARTESIAN_POINT('Ctrl Pts',(158.905499537228,-0.837564463467088,
16.6254376054632));
#26363=CARTESIAN_POINT('Ctrl Pts',(158.944730812722,-3.47494889088804,16.0545866524418));
#26364=CARTESIAN_POINT('Ctrl Pts',(158.983962088217,-6.11233331830896,15.4837356994203));
#26365=CARTESIAN_POINT('Ctrl Pts',(159.023193363711,-8.60608351464021,14.2492812570547));
#26366=CARTESIAN_POINT('Ctrl Pts',(159.062424639206,-10.659242455622,12.4982227795519));
#26367=CARTESIAN_POINT('Ctrl Pts',(159.1016559147,-12.7124013966038,10.7471643020491));
#26368=CARTESIAN_POINT('Ctrl Pts',(159.140887190194,-14.3249690822362,8.47950178940902));
#26369=CARTESIAN_POINT('Ctrl Pts',(159.180118465689,-15.3049201436399,5.96526963111059));
#26370=CARTESIAN_POINT('Ctrl Pts',(159.209693361409,-16.0436662100445,4.06989016766049));
#26371=CARTESIAN_POINT('Ctrl Pts',(159.239268257128,-16.4228929943252,2.03438390607463));
#26372=CARTESIAN_POINT('Ctrl Pts',(159.268843152848,-16.4248806122125,-0.000401937761208326));
#26373=CARTESIAN_POINT('Origin',(157.6,0.,0.));
#26374=CARTESIAN_POINT('',(160.981156847152,-16.4236740929622,-4.03570622692362E-5));
#26375=CARTESIAN_POINT('',(160.768843152848,-16.4236679926984,2.89616052317413E-6));
#26376=CARTESIAN_POINT('',(157.6,-16.425,-2.01148236759953E-15));
#26377=CARTESIAN_POINT('Ctrl Pts',(160.981156847152,-16.4236740929622,-4.03570622692362E-5));
#26378=CARTESIAN_POINT('Ctrl Pts',(160.960880704809,-16.4235519097392,1.39527506482232));
#26379=CARTESIAN_POINT('Ctrl Pts',(160.940604562465,-16.2475393266592,2.79062075644783));
#26380=CARTESIAN_POINT('Ctrl Pts',(160.920328420122,-15.8960160304352,4.14025318335245));
#26381=CARTESIAN_POINT('Ctrl Pts',(160.881097144628,-15.2158715017878,6.7515882519092));
#26382=CARTESIAN_POINT('Ctrl Pts',(160.841865869133,-13.8786778735385,9.19178926895033));
#26383=CARTESIAN_POINT('Ctrl Pts',(160.802634593639,-12.0436688336838,11.1702758733465));
#26384=CARTESIAN_POINT('Ctrl Pts',(160.763403318144,-10.2086597938292,13.1487624777426));
#26385=CARTESIAN_POINT('Ctrl Pts',(160.72417204265,-7.8758353423693,14.6655346694938));
#26386=CARTESIAN_POINT('Ctrl Pts',(160.684940767156,-5.32298938514325,15.5399744551839));
#26387=CARTESIAN_POINT('Ctrl Pts',(160.645709491661,-2.77014342791723,16.4144142408739));
#26388=CARTESIAN_POINT('Ctrl Pts',(160.606478216167,0.00272403507491303,
16.6465216205029));
#26389=CARTESIAN_POINT('Ctrl Pts',(160.567246940672,2.66541855545244,16.2086571308781));
#26390=CARTESIAN_POINT('Ctrl Pts',(160.528015665178,5.32811307583003,15.7707926412532));
#26391=CARTESIAN_POINT('Ctrl Pts',(160.488784389684,7.88063465359301,14.6629562823745));
#26392=CARTESIAN_POINT('Ctrl Pts',(160.449553114189,10.0190277389006,13.0170697635549));
#26393=CARTESIAN_POINT('Ctrl Pts',(160.410321838695,12.157420824208,11.3711832447354));
#26394=CARTESIAN_POINT('Ctrl Pts',(160.3710905632,13.8816854170602,9.18724656597482));
#26395=CARTESIAN_POINT('Ctrl Pts',(160.331859287706,14.9864952248381,6.72532400245657));
#26396=CARTESIAN_POINT('Ctrl Pts',(160.292628012212,16.0913050326161,4.26340143893821));
#26397=CARTESIAN_POINT('Ctrl Pts',(160.253396736717,16.57666005532,1.52349299066212));
#26398=CARTESIAN_POINT('Ctrl Pts',(160.214165461223,16.384763973389,-1.16813166999598));
#26399=CARTESIAN_POINT('Ctrl Pts',(160.174934185728,16.1928678914581,-3.85975633065405));
#26400=CARTESIAN_POINT('Ctrl Pts',(160.135702910234,15.3237207048923,-6.50309720369402));
#26401=CARTESIAN_POINT('Ctrl Pts',(160.09647163474,13.8808208966376,-8.783383932038));
#26402=CARTESIAN_POINT('Ctrl Pts',(160.057240359245,12.4379210883829,-11.063670660382));
#26403=CARTESIAN_POINT('Ctrl Pts',(160.018009083751,10.4212686584393,-12.98090324403));
#26404=CARTESIAN_POINT('Ctrl Pts',(159.978777808256,8.07100758972996,-14.3067766652253));
#26405=CARTESIAN_POINT('Ctrl Pts',(159.939546532762,5.7207465210206,-15.6326500864207));
#26406=CARTESIAN_POINT('Ctrl Pts',(159.900315257268,3.03687681354547,-16.3671643451634));
#26407=CARTESIAN_POINT('Ctrl Pts',(159.861083981773,0.338995018316543,-16.4228531150854));
#26408=CARTESIAN_POINT('Ctrl Pts',(159.821852706279,-2.35888677691235,-16.4785418850075));
#26409=CARTESIAN_POINT('Ctrl Pts',(159.782621430785,-5.07078065989505,-15.8554051661089));
#26410=CARTESIAN_POINT('Ctrl Pts',(159.74339015529,-7.47375294674307,-14.6276463914453));
#26411=CARTESIAN_POINT('Ctrl Pts',(159.704158879796,-9.87672523359113,-13.3998876167818));
#26412=CARTESIAN_POINT('Ctrl Pts',(159.664927604301,-11.9707759243045,-11.5675067863533));
#26413=CARTESIAN_POINT('Ctrl Pts',(159.625696328807,-13.5065444122441,-9.34870472858095));
#26414=CARTESIAN_POINT('Ctrl Pts',(159.586465053313,-15.0423129001837,-7.12990267080861));
#26415=CARTESIAN_POINT('Ctrl Pts',(159.547233777818,-16.0197991853496,-4.52467938569242));
#26416=CARTESIAN_POINT('Ctrl Pts',(159.508002502324,-16.3226037105909,-1.84326616882031));
#26417=CARTESIAN_POINT('Ctrl Pts',(159.4990539506,-16.3916726338472,-1.23164280042124));
#26418=CARTESIAN_POINT('Ctrl Pts',(159.490105398876,-16.4256389301963,-0.616055390147352));
#26419=CARTESIAN_POINT('Ctrl Pts',(159.481156847152,-16.4250281341261,-0.000400964822849792));
#26420=CARTESIAN_POINT('Ctrl Pts',(159.268843152848,-16.4248806122125,-0.000401937761208326));
#26421=CARTESIAN_POINT('Ctrl Pts',(159.278499532623,-16.4255295813027,-0.664771646930069));
#26422=CARTESIAN_POINT('Ctrl Pts',(159.288155912397,-16.3859625378202,-1.32906455514114));
#26423=CARTESIAN_POINT('Ctrl Pts',(159.297812292172,-16.3055626961613,-1.98837811710903));
#26424=CARTESIAN_POINT('Ctrl Pts',(159.337043567666,-15.9789197501039,-4.66699190307352));
#26425=CARTESIAN_POINT('Ctrl Pts',(159.376274843161,-14.9782994208139,-7.26341767104574));
#26426=CARTESIAN_POINT('Ctrl Pts',(159.415506118655,-13.4228560790206,-9.46847173819219));
#26427=CARTESIAN_POINT('Ctrl Pts',(159.45473739415,-11.8674127372274,-11.6735258053386));
#26428=CARTESIAN_POINT('Ctrl Pts',(159.493968669644,-9.75714638293084,-13.4872081716593));
#26429=CARTESIAN_POINT('Ctrl Pts',(159.533199945138,-7.34334859212344,-14.6935446312183));
#26430=CARTESIAN_POINT('Ctrl Pts',(159.572431220633,-4.92955080131603,-15.8998810907773));
#26431=CARTESIAN_POINT('Ctrl Pts',(159.611662496127,-2.21222157399777,-16.4988716435747));
#26432=CARTESIAN_POINT('Ctrl Pts',(159.650893771621,0.485058162412974,-16.4191881941259));
#26433=CARTESIAN_POINT('Ctrl Pts',(159.690125047116,3.18233789882364,-16.339504744677));
#26434=CARTESIAN_POINT('Ctrl Pts',(159.72935632261,5.85956814432678,-15.5811472929821));
#26435=CARTESIAN_POINT('Ctrl Pts',(159.768587598105,8.19794297837249,-14.2344214247857));
#26436=CARTESIAN_POINT('Ctrl Pts',(159.807818873599,10.5363178124183,-12.8876955565893));
#26437=CARTESIAN_POINT('Ctrl Pts',(159.847050149093,12.5358372350066,-10.9526012718913));
#26438=CARTESIAN_POINT('Ctrl Pts',(159.886281424588,13.9583974703242,-8.65957056876912));
#26439=CARTESIAN_POINT('Ctrl Pts',(159.925512700082,15.3809577056418,-6.36653986564693));
#26440=CARTESIAN_POINT('Ctrl Pts',(159.964743975577,16.2265587536887,-3.71557274410037));
#26441=CARTESIAN_POINT('Ctrl Pts',(160.003975251071,16.3945060175047,-1.02234769870506));
#26442=CARTESIAN_POINT('Ctrl Pts',(160.043206526566,16.5624532813207,1.67087734669029));
#26443=CARTESIAN_POINT('Ctrl Pts',(160.08243780206,16.0527467609058,4.40636031593449));
#26444=CARTESIAN_POINT('Ctrl Pts',(160.121669077554,14.926082564383,6.8583585249146));
#26445=CARTESIAN_POINT('Ctrl Pts',(160.160900353049,13.7994183678601,9.3103567338947));
#26446=CARTESIAN_POINT('Ctrl Pts',(160.200131628543,12.0557964952294,11.4788701826107));
#26447=CARTESIAN_POINT('Ctrl Pts',(160.239362904037,9.90284831369518,13.1056712018496));
#26448=CARTESIAN_POINT('Ctrl Pts',(160.278594179532,7.74990013216097,14.7324722210885));
#26449=CARTESIAN_POINT('Ctrl Pts',(160.317825455026,5.18762564172333,15.8175608108503));
#26450=CARTESIAN_POINT('Ctrl Pts',(160.357056730521,2.52114177395646,16.231724077579));
#26451=CARTESIAN_POINT('Ctrl Pts',(160.396288006015,-0.145342093810331,
16.6458873443076));
#26452=CARTESIAN_POINT('Ctrl Pts',(160.435519281509,-2.91603533890632,16.3891252880031));
#26453=CARTESIAN_POINT('Ctrl Pts',(160.474750557004,-5.46100241990846,15.4920132631237));
#26454=CARTESIAN_POINT('Ctrl Pts',(160.513981832498,-8.00596950091064,14.5949012382442));
#26455=CARTESIAN_POINT('Ctrl Pts',(160.553213107993,-10.325210417819,13.0574392447898));
#26456=CARTESIAN_POINT('Ctrl Pts',(160.592444383487,-12.1425487989022,11.0627090281415));
#26457=CARTESIAN_POINT('Ctrl Pts',(160.631675658981,-13.9598871799855,9.06797881149322));
#26458=CARTESIAN_POINT('Ctrl Pts',(160.670906934476,-15.2753230252437,6.61598037165108));
#26459=CARTESIAN_POINT('Ctrl Pts',(160.71013820997,-15.9322135743927,3.99869891276921));
#26460=CARTESIAN_POINT('Ctrl Pts',(160.729706524263,-16.2598664625444,2.69321532768862));
#26461=CARTESIAN_POINT('Ctrl Pts',(160.749274838555,-16.4236764509222,1.34661012305833));
#26462=CARTESIAN_POINT('Ctrl Pts',(160.768843152848,-16.4236679926984,2.89616052317413E-6));
#26463=CARTESIAN_POINT('Origin',(157.6,0.,0.));
#26464=CARTESIAN_POINT('',(162.481156847152,-16.4247551753985,0.000398700478366487));
#26465=CARTESIAN_POINT('',(162.268843152848,-16.4249001992122,0.000402101984826423));
#26466=CARTESIAN_POINT('',(157.6,-16.425,-2.01148236759953E-15));
#26467=CARTESIAN_POINT('Ctrl Pts',(162.481156847152,-16.4247551753985,0.000398700478366487));
#26468=CARTESIAN_POINT('Ctrl Pts',(162.470887286236,-16.4254300789369,0.706971482165368));
#26469=CARTESIAN_POINT('Ctrl Pts',(162.46061772532,-16.38066296943,1.41345935288586));
#26470=CARTESIAN_POINT('Ctrl Pts',(162.450348164403,-16.2897574053744,2.11395972898341));
#26471=CARTESIAN_POINT('Ctrl Pts',(162.411116888909,-15.9424844054321,4.78997708386633));
#26472=CARTESIAN_POINT('Ctrl Pts',(162.371885613415,-14.9218873213385,7.37861560534905));
#26473=CARTESIAN_POINT('Ctrl Pts',(162.33265433792,-13.3494993657526,9.57161891980958));
#26474=CARTESIAN_POINT('Ctrl Pts',(162.293423062426,-11.7771114101666,11.7646222342701));
#26475=CARTESIAN_POINT('Ctrl Pts',(162.254191786932,-9.65293258308827,13.5619903417085));
#26476=CARTESIAN_POINT('Ctrl Pts',(162.214960511437,-7.22991116477318,14.749691746323));
#26477=CARTESIAN_POINT('Ctrl Pts',(162.175729235943,-4.80688974645808,15.9373931509376));
#26478=CARTESIAN_POINT('Ctrl Pts',(162.136497960448,-2.08502573690623,16.5154278527283));
#26479=CARTESIAN_POINT('Ctrl Pts',(162.097266684954,0.611559932333494,16.4149631894586));
#26480=CARTESIAN_POINT('Ctrl Pts',(162.058035409459,3.30814560157322,16.314498526189));
#26481=CARTESIAN_POINT('Ctrl Pts',(162.018804133965,5.97945293050085,15.5355344978588));
#26482=CARTESIAN_POINT('Ctrl Pts',(161.979572858471,8.30738130243708,14.1708305316958));
#26483=CARTESIAN_POINT('Ctrl Pts',(161.940341582976,10.6353096743733,12.8061265655328));
#26484=CARTESIAN_POINT('Ctrl Pts',(161.901110307482,12.6198590893181,10.8556826615369));
#26485=CARTESIAN_POINT('Ctrl Pts',(161.861879031988,14.0247084074806,8.55175865815035));
#26486=CARTESIAN_POINT('Ctrl Pts',(161.822647756493,15.429557725643,6.24783465476382));
#26487=CARTESIAN_POINT('Ctrl Pts',(161.783416480999,16.254706947023,3.5904305519868));
#26488=CARTESIAN_POINT('Ctrl Pts',(161.744185205504,16.4018968884372,0.895991363348477));
#26489=CARTESIAN_POINT('Ctrl Pts',(161.70495393001,16.5490868298513,-1.79844782528973));
#26490=CARTESIAN_POINT('Ctrl Pts',(161.665722654515,16.0183174912997,-4.52992209978915));
#26491=CARTESIAN_POINT('Ctrl Pts',(161.626491379021,14.872793151855,-6.97316613341791));
#26492=CARTESIAN_POINT('Ctrl Pts',(161.587260103527,13.7272688124102,-9.41641016704681));
#26493=CARTESIAN_POINT('Ctrl Pts',(161.548028828032,11.9669894720722,-11.571423959805));
#26494=CARTESIAN_POINT('Ctrl Pts',(161.508797552538,9.80157007765527,-13.1815873882825));
#26495=CARTESIAN_POINT('Ctrl Pts',(161.469566277044,7.63615068323841,-14.7917508167599));
#26496=CARTESIAN_POINT('Ctrl Pts',(161.430335001549,5.0655912347426,-15.8570638809565));
#26497=CARTESIAN_POINT('Ctrl Pts',(161.391103726055,2.3959952407036,-16.2506685668203));
#26498=CARTESIAN_POINT('Ctrl Pts',(161.35187245056,-0.273600753335407,-16.644273252684));
#26499=CARTESIAN_POINT('Ctrl Pts',(161.312641175066,-3.04223329291763,-16.3661695602148));
#26500=CARTESIAN_POINT('Ctrl Pts',(161.273409899572,-5.58021222646632,-15.4494742166104));
#26501=CARTESIAN_POINT('Ctrl Pts',(161.234178624077,-8.11819116001507,-14.532778873006));
#26502=CARTESIAN_POINT('Ctrl Pts',(161.194947348583,-10.4255164875303,-12.9774918782664));
#26503=CARTESIAN_POINT('Ctrl Pts',(161.155716073088,-12.2274307516426,-10.9688175878669));
#26504=CARTESIAN_POINT('Ctrl Pts',(161.116484797594,-14.0293450157549,-8.96014329746748));
#26505=CARTESIAN_POINT('Ctrl Pts',(161.0772535221,-15.3258482164643,-6.49808171140809));
#26506=CARTESIAN_POINT('Ctrl Pts',(161.038022246605,-15.9625521022962,-3.87581635834224));
#26507=CARTESIAN_POINT('Ctrl Pts',(161.019067113454,-16.2701843875503,-2.60883259861186));
#26508=CARTESIAN_POINT('Ctrl Pts',(161.000111980303,-16.4237883158366,-1.30444970484835));
#26509=CARTESIAN_POINT('Ctrl Pts',(160.981156847152,-16.4236740929622,-4.03570622692362E-5));
#26510=CARTESIAN_POINT('Ctrl Pts',(160.768843152848,-16.4236679926984,2.89616052317413E-6));
#26511=CARTESIAN_POINT('Ctrl Pts',(160.78850611405,-16.4236594935644,-1.35311752394874));
#26512=CARTESIAN_POINT('Ctrl Pts',(160.808169075252,-16.2582440199641,-2.70623998593522));
#26513=CARTESIAN_POINT('Ctrl Pts',(160.827832036453,-15.9274463816101,-4.01764534721292));
#26514=CARTESIAN_POINT('Ctrl Pts',(160.867063311948,-15.2674433866387,-6.63414367039156));
#26515=CARTESIAN_POINT('Ctrl Pts',(160.906294587442,-13.9490921436561,-9.0845758388273));
#26516=CARTESIAN_POINT('Ctrl Pts',(160.945525862937,-12.12938257997,-11.0771431607507));
#26517=CARTESIAN_POINT('Ctrl Pts',(160.984757138431,-10.3096730162838,-13.0697104826741));
#26518=CARTESIAN_POINT('Ctrl Pts',(161.023988413925,-7.98860513189412,-14.6044129580852));
#26519=CARTESIAN_POINT('Ctrl Pts',(161.06321968942,-5.44257285473611,-15.4984974463957));
#26520=CARTESIAN_POINT('Ctrl Pts',(161.102450964914,-2.89654057757807,-16.3925819347062));
#26521=CARTESIAN_POINT('Ctrl Pts',(161.141682240409,-0.125543907651698,
-16.6460484359161));
#26522=CARTESIAN_POINT('Ctrl Pts',(161.180913515903,2.54044548163889,-16.2287140319209));
#26523=CARTESIAN_POINT('Ctrl Pts',(161.220144791397,5.20643487092948,-15.8113796279257));
#26524=CARTESIAN_POINT('Ctrl Pts',(161.259376066892,7.76741697958431,-14.7232443187254));
#26525=CARTESIAN_POINT('Ctrl Pts',(161.298607342386,9.91842877350012,-13.093883802755));
#26526=CARTESIAN_POINT('Ctrl Pts',(161.33783861788,12.0694405674159,-11.4645232867847));
#26527=CARTESIAN_POINT('Ctrl Pts',(161.377069893375,13.8104820465927,-9.29393756404428));
#26528=CARTESIAN_POINT('Ctrl Pts',(161.416301168869,14.9342291183729,-6.84060107117715));
#26529=CARTESIAN_POINT('Ctrl Pts',(161.455532444364,16.057976190153,-4.38726457831001));
#26530=CARTESIAN_POINT('Ctrl Pts',(161.494763719858,16.5644288545364,-1.65117731531621));
#26531=CARTESIAN_POINT('Ctrl Pts',(161.533994995353,16.3932784742086,1.04184607408865));
#26532=CARTESIAN_POINT('Ctrl Pts',(161.573226270847,16.2221280938808,3.73486946349348));
#26533=CARTESIAN_POINT('Ctrl Pts',(161.612457546341,15.3733746688418,6.3848289793093));
#26534=CARTESIAN_POINT('Ctrl Pts',(161.651688821836,13.9480881826851,8.6761661131565));
#26535=CARTESIAN_POINT('Ctrl Pts',(161.69092009733,12.5228016965284,10.9675032470038));
#26536=CARTESIAN_POINT('Ctrl Pts',(161.730151372824,10.5209821492541,12.9002179988825));
#26537=CARTESIAN_POINT('Ctrl Pts',(161.769382648319,8.18100721667673,14.244161726677));
#26538=CARTESIAN_POINT('Ctrl Pts',(161.808613923813,5.84103228409951,15.5881054544714));
#26539=CARTESIAN_POINT('Ctrl Pts',(161.847845199308,3.16290196621933,16.3432781581817));
#26540=CARTESIAN_POINT('Ctrl Pts',(161.887076474802,0.465529364656197,16.4197534934507));
#26541=CARTESIAN_POINT('Ctrl Pts',(161.926307750296,-2.23184323690693,16.4962288287198));
#26542=CARTESIAN_POINT('Ctrl Pts',(161.965539025791,-4.94845812215303,15.8940067955476));
#26543=CARTESIAN_POINT('Ctrl Pts',(162.004770301285,-7.36081942787581,14.6848002957225));
#26544=CARTESIAN_POINT('Ctrl Pts',(162.04400157678,-9.77318073359862,13.4755937958975));
#26545=CARTESIAN_POINT('Ctrl Pts',(162.083232852274,-11.8812884597981,11.6594028294195));
#26546=CARTESIAN_POINT('Ctrl Pts',(162.122464127769,-13.4341080809988,9.4525003275898));
#26547=CARTESIAN_POINT('Ctrl Pts',(162.161695403263,-14.9869277021995,7.24559782576006));
#26548=CARTESIAN_POINT('Ctrl Pts',(162.200926678757,-15.9844592184014,4.6479837885785));
#26549=CARTESIAN_POINT('Ctrl Pts',(162.240157954252,-16.3079160762864,1.96898339857192));
#26550=CARTESIAN_POINT('Ctrl Pts',(162.249719687117,-16.386751343038,1.31603786588246));
#26551=CARTESIAN_POINT('Ctrl Pts',(162.259281419983,-16.4255445549274,0.658257739925561));
#26552=CARTESIAN_POINT('Ctrl Pts',(162.268843152848,-16.4249001992122,0.000402101984826423));
#26553=CARTESIAN_POINT('Origin',(157.6,0.,0.));
#26554=CARTESIAN_POINT('',(163.981156847152,-16.426349720506,1.83455734200678E-5));
#26555=CARTESIAN_POINT('',(163.768843152848,-16.4263461654774,-3.0980125475399E-5));
#26556=CARTESIAN_POINT('',(157.6,-16.425,-2.01148236759953E-15));
#26557=CARTESIAN_POINT('Ctrl Pts',(163.981156847152,-16.426349720506,1.83455734200678E-5));
#26558=CARTESIAN_POINT('Ctrl Pts',(163.980893867663,-16.4263509381512,0.0181069480969145));
#26559=CARTESIAN_POINT('Ctrl Pts',(163.980630888174,-16.4263216708674,0.0361955466634846));
#26560=CARTESIAN_POINT('Ctrl Pts',(163.980367908685,-16.4262618946208,0.054284044404482));
#26561=CARTESIAN_POINT('Ctrl Pts',(163.94113663319,-16.4173444752216,2.75272581608827));
#26562=CARTESIAN_POINT('Ctrl Pts',(163.901905357696,-15.7294602457597,5.44892374822015));
#26563=CARTESIAN_POINT('Ctrl Pts',(163.862674082202,-14.444523408231,7.82181331292719));
#26564=CARTESIAN_POINT('Ctrl Pts',(163.823442806707,-13.1595865707024,10.1947028776342));
#26565=CARTESIAN_POINT('Ctrl Pts',(163.784211531213,-11.2775971251071,12.2442840749163));
#26566=CARTESIAN_POINT('Ctrl Pts',(163.744980255719,-9.02266302473022,13.7264917114902));
#26567=CARTESIAN_POINT('Ctrl Pts',(163.705748980224,-6.76772892435329,15.2086993480642));
#26568=CARTESIAN_POINT('Ctrl Pts',(163.66651770473,-4.13985016919475,16.1235334239298));
#26569=CARTESIAN_POINT('Ctrl Pts',(163.627286429235,-1.45195602286144,16.3620550561079));
#26570=CARTESIAN_POINT('Ctrl Pts',(163.588055153741,1.23593812347187,16.6005766882859));
#26571=CARTESIAN_POINT('Ctrl Pts',(163.548823878247,3.98384766097998,16.1627858767762));
#26572=CARTESIAN_POINT('Ctrl Pts',(163.509592602752,6.46455021341737,15.1008149624023));
#26573=CARTESIAN_POINT('Ctrl Pts',(163.470361327258,8.94525276585476,14.0388440480284));
#26574=CARTESIAN_POINT('Ctrl Pts',(163.431130051763,11.1587483332215,12.3526930307903));
#26575=CARTESIAN_POINT('Ctrl Pts',(163.391898776269,12.8414527190008,10.2431496238017));
#26576=CARTESIAN_POINT('Ctrl Pts',(163.352667500774,14.5241571047801,8.13360621681312));
#26577=CARTESIAN_POINT('Ctrl Pts',(163.31343622528,15.676070308972,5.60067042007414));
#26578=CARTESIAN_POINT('Ctrl Pts',(163.274204949786,16.1600219460145,2.94596549675071));
#26579=CARTESIAN_POINT('Ctrl Pts',(163.234973674291,16.643973583057,0.291260573427248));
#26580=CARTESIAN_POINT('Ctrl Pts',(163.195742398797,16.45996365295,-2.48521347648057));
#26581=CARTESIAN_POINT('Ctrl Pts',(163.156511123302,15.6299041423788,-5.05283272941568));
#26582=CARTESIAN_POINT('Ctrl Pts',(163.117279847808,14.7998446318076,-7.62045198235076));
#26583=CARTESIAN_POINT('Ctrl Pts',(163.078048572314,13.3237355407723,-9.97921643831304));
#26584=CARTESIAN_POINT('Ctrl Pts',(163.038817296819,11.3773526842037,-11.8482432432018));
#26585=CARTESIAN_POINT('Ctrl Pts',(162.999586021325,9.43096982763521,-13.7172700480906));
#26586=CARTESIAN_POINT('Ctrl Pts',(162.960354745831,7.01431320553354,-15.0965592019059));
#26587=CARTESIAN_POINT('Ctrl Pts',(162.921123470336,4.41515949874548,-15.8218642601142));
#26588=CARTESIAN_POINT('Ctrl Pts',(162.881892194842,1.81600579195742,-16.5471693183225));
#26589=CARTESIAN_POINT('Ctrl Pts',(162.842660919347,-0.965644999517052,
-16.6184902809239));
#26590=CARTESIAN_POINT('Ctrl Pts',(162.803429643853,-3.59855250319817,-16.0273342120322));
#26591=CARTESIAN_POINT('Ctrl Pts',(162.764198368359,-6.23146000687928,-15.4361781431406));
#26592=CARTESIAN_POINT('Ctrl Pts',(162.724967092864,-8.71562422276706,-14.182545042756));
#26593=CARTESIAN_POINT('Ctrl Pts',(162.68573581737,-10.7552296304183,-12.4157181692461));
#26594=CARTESIAN_POINT('Ctrl Pts',(162.646504541875,-12.7948350380696,-10.6488912957361));
#26595=CARTESIAN_POINT('Ctrl Pts',(162.607273266381,-14.3898816374843,-8.36887064910085));
#26596=CARTESIAN_POINT('Ctrl Pts',(162.568041990887,-15.3504304792961,-5.84716223164164));
#26597=CARTESIAN_POINT('Ctrl Pts',(162.539080276308,-16.0595366973441,-3.98556077933925));
#26598=CARTESIAN_POINT('Ctrl Pts',(162.51011856173,-16.4228518453724,-1.99224338023886));
#26599=CARTESIAN_POINT('Ctrl Pts',(162.481156847152,-16.4247551753985,0.000398700478366487));
#26600=CARTESIAN_POINT('Ctrl Pts',(162.268843152848,-16.4249001992122,0.000402101984826423));
#26601=CARTESIAN_POINT('Ctrl Pts',(162.298512695477,-16.4229007980964,-2.04088854774718));
#26602=CARTESIAN_POINT('Ctrl Pts',(162.328182238106,-16.041185646821,-4.08290624763289));
#26603=CARTESIAN_POINT('Ctrl Pts',(162.357851780735,-15.2978144185396,-5.98346859195882));
#26604=CARTESIAN_POINT('Ctrl Pts',(162.397083056229,-14.3148737033398,-8.49653344965138));
#26605=CARTESIAN_POINT('Ctrl Pts',(162.436314331724,-12.699610073372,-10.7622764222049));
#26606=CARTESIAN_POINT('Ctrl Pts',(162.475545607218,-10.6443699319163,-12.5108916999377));
#26607=CARTESIAN_POINT('Ctrl Pts',(162.514776882712,-8.58912979046056,-14.2595069776706));
#26608=CARTESIAN_POINT('Ctrl Pts',(162.554008158207,-6.09391313751689,-15.4909945605828));
#26609=CARTESIAN_POINT('Ctrl Pts',(162.593239433701,-3.45585162373997,-16.0587082895774));
#26610=CARTESIAN_POINT('Ctrl Pts',(162.632470709196,-0.817790109963057,
-16.6264220185721));
#26611=CARTESIAN_POINT('Ctrl Pts',(162.67170198469,1.96311626464708,-16.5303618936492));
#26612=CARTESIAN_POINT('Ctrl Pts',(162.710933260184,4.55571577409399,-15.7819668026727));
#26613=CARTESIAN_POINT('Ctrl Pts',(162.750164535679,7.1483152835409,-15.0335717116962));
#26614=CARTESIAN_POINT('Ctrl Pts',(162.789395811173,9.55260792782455,-13.6328416546661));
#26615=CARTESIAN_POINT('Ctrl Pts',(162.828627086668,11.4822893328306,-11.7465762693808));
#26616=CARTESIAN_POINT('Ctrl Pts',(162.867858362162,13.4119707378367,-9.86031088409554));
#26617=CARTESIAN_POINT('Ctrl Pts',(162.907089637656,14.8670409035652,-7.4885101705551));
#26618=CARTESIAN_POINT('Ctrl Pts',(162.946320913151,15.6742293448598,-4.91360934745356));
#26619=CARTESIAN_POINT('Ctrl Pts',(162.985552188645,16.4814177861543,-2.33870852435206));
#26620=CARTESIAN_POINT('Ctrl Pts',(163.02478346414,16.6407245030151,0.439292408310395));
#26621=CARTESIAN_POINT('Ctrl Pts',(163.064014739634,16.1331791715844,3.08958770604198));
#26622=CARTESIAN_POINT('Ctrl Pts',(163.103246015128,15.6256338401538,5.73988300377354));
#26623=CARTESIAN_POINT('Ctrl Pts',(163.142477290623,14.4512364604316,8.26247266657433));
#26624=CARTESIAN_POINT('Ctrl Pts',(163.181708566117,12.7498348616949,10.3569654519852));
#26625=CARTESIAN_POINT('Ctrl Pts',(163.220939841612,11.0484332629582,12.4514582373962));
#26626=CARTESIAN_POINT('Ctrl Pts',(163.260171117106,8.82002744520687,14.1178541454175));
#26627=CARTESIAN_POINT('Ctrl Pts',(163.2994023926,6.32997709056114,15.157717915582));
#26628=CARTESIAN_POINT('Ctrl Pts',(163.338633668095,3.83992673591541,16.1975816857465));
#26629=CARTESIAN_POINT('Ctrl Pts',(163.377864943589,1.08823184437532,16.6109133180543));
#26630=CARTESIAN_POINT('Ctrl Pts',(163.417096219084,-1.59743437520489,16.348493074124));
#26631=CARTESIAN_POINT('Ctrl Pts',(163.456327494578,-4.2831005947851,16.0860728301938));
#26632=CARTESIAN_POINT('Ctrl Pts',(163.495558770072,-6.90273814240541,15.1479007100255));
#26633=CARTESIAN_POINT('Ctrl Pts',(163.534790045567,-9.14439926671966,13.6456947208487));
#26634=CARTESIAN_POINT('Ctrl Pts',(163.574021321061,-11.3860603910339,12.1434887316718));
#26635=CARTESIAN_POINT('Ctrl Pts',(163.613252596556,-13.249745092042,10.0772488734865));
#26636=CARTESIAN_POINT('Ctrl Pts',(163.65248387205,-14.5135248569151,7.69302402388132));
#26637=CARTESIAN_POINT('Ctrl Pts',(163.691270298983,-15.7629744578162,5.33583421154308));
#26638=CARTESIAN_POINT('Ctrl Pts',(163.730056725915,-16.4260467902704,2.66782986936085));
#26639=CARTESIAN_POINT('Ctrl Pts',(163.768843152848,-16.4263461654774,-3.0980125475399E-5));
#26640=CARTESIAN_POINT('Origin',(157.6,0.,0.));
#26641=CARTESIAN_POINT('',(165.275,-16.425,-2.01148236759953E-15));
#26642=CARTESIAN_POINT('',(165.268843152848,-16.4247445391107,-0.000389063610209933));
#26643=CARTESIAN_POINT('',(157.6,-16.425,-2.01148236759953E-15));
#26644=CARTESIAN_POINT('',(165.275,-10.6720568218313,12.4855047231421));
#26645=CARTESIAN_POINT('Origin',(165.275,0.,0.));
#26646=CARTESIAN_POINT('Ctrl Pts',(165.275,-10.6720568218312,12.4855047231422));
#26647=CARTESIAN_POINT('Ctrl Pts',(165.235768724506,-8.6202940722137,14.2392607093338));
#26648=CARTESIAN_POINT('Ctrl Pts',(165.196537449011,-6.12897562101673,15.4767795574399));
#26649=CARTESIAN_POINT('Ctrl Pts',(165.157306173517,-3.49257059628647,16.0506648722972));
#26650=CARTESIAN_POINT('Ctrl Pts',(165.118074898022,-0.856165571556061,
16.6245501871546));
#26651=CARTESIAN_POINT('Ctrl Pts',(165.078843622528,1.92532602670759,16.5348019687632));
#26652=CARTESIAN_POINT('Ctrl Pts',(165.039612347034,4.51972495057751,15.7923235953478));
#26653=CARTESIAN_POINT('Ctrl Pts',(165.000381071539,7.11412387444743,15.0498452219324));
#26654=CARTESIAN_POINT('Ctrl Pts',(164.961149796045,9.52143012392356,13.654636693493));
#26655=CARTESIAN_POINT('Ctrl Pts',(164.92191852055,11.4553706815436,11.7727924865797));
#26656=CARTESIAN_POINT('Ctrl Pts',(164.882687245056,13.3893112391636,9.89094827966651));
#26657=CARTESIAN_POINT('Ctrl Pts',(164.843455969562,14.8498861049275,7.52246839427947));
#26658=CARTESIAN_POINT('Ctrl Pts',(164.804224694067,15.6629797279521,4.94941629810398));
#26659=CARTESIAN_POINT('Ctrl Pts',(164.764993418573,16.4760733509766,2.37636420192853));
#26660=CARTESIAN_POINT('Ctrl Pts',(164.725762143078,16.6416857312619,-0.401260105035436));
#26661=CARTESIAN_POINT('Ctrl Pts',(164.686530867584,16.1401878137618,-3.052707085354));
#26662=CARTESIAN_POINT('Ctrl Pts',(164.64729959209,15.6386898962617,-5.70415406567245));
#26663=CARTESIAN_POINT('Ctrl Pts',(164.608068316595,14.4700816809762,-8.22942371934558));
#26664=CARTESIAN_POINT('Ctrl Pts',(164.568837041101,12.773476700623,-10.3278001313319));
#26665=CARTESIAN_POINT('Ctrl Pts',(164.529605765607,11.0768717202696,-12.4261765433184));
#26666=CARTESIAN_POINT('Ctrl Pts',(164.490374490112,8.85226997484841,-14.0976597136181));
#26667=CARTESIAN_POINT('Ctrl Pts',(164.451143214618,6.36460005341017,-15.1432112869903));
#26668=CARTESIAN_POINT('Ctrl Pts',(164.411911939123,3.87693013197185,-16.1887628603625));
#26669=CARTESIAN_POINT('Ctrl Pts',(164.372680663629,1.1261920345165,-16.6083828368073));
#26670=CARTESIAN_POINT('Ctrl Pts',(164.333449388134,-1.56006564138621,-16.3521013432403));
#26671=CARTESIAN_POINT('Ctrl Pts',(164.29421811264,-4.24632331728882,-16.0958198496733));
#26672=CARTESIAN_POINT('Ctrl Pts',(164.254986837146,-6.86810057163888,-15.1636368860945));
#26673=CARTESIAN_POINT('Ctrl Pts',(164.215755561651,-9.11318964993117,-13.6665579088443));
#26674=CARTESIAN_POINT('Ctrl Pts',(164.176524286157,-11.3582787282235,-12.169478931594));
#26675=CARTESIAN_POINT('Ctrl Pts',(164.137293010662,-13.2266796304581,-10.1075039406724));
#26676=CARTESIAN_POINT('Ctrl Pts',(164.098061735168,-14.4959047769073,-7.72617363959368));
#26677=CARTESIAN_POINT('Ctrl Pts',(164.059093439163,-15.7566219109044,-5.36080613905552));
#26678=CARTESIAN_POINT('Ctrl Pts',(164.020125143157,-16.4261692898643,-2.68035045503792));
#26679=CARTESIAN_POINT('Ctrl Pts',(163.981156847152,-16.426349720506,1.83455734200678E-5));
#26680=CARTESIAN_POINT('Ctrl Pts',(163.768843152848,-16.4263461654774,-3.0980125475399E-5));
#26681=CARTESIAN_POINT('Ctrl Pts',(163.76928800141,-16.4263495990659,-0.0306291598356519));
#26682=CARTESIAN_POINT('Ctrl Pts',(163.769732849971,-16.426265850095,-0.0612273206704939));
#26683=CARTESIAN_POINT('Ctrl Pts',(163.770177698533,-16.4260948033082,-0.0918249934937266));
#26684=CARTESIAN_POINT('Ctrl Pts',(163.809408974028,-16.4110101560904,-2.79023932023853));
#26685=CARTESIAN_POINT('Ctrl Pts',(163.848640249522,-15.7169660329169,-5.48485813270309));
#26686=CARTESIAN_POINT('Ctrl Pts',(163.887871525016,-14.4266095401332,-7.85480487595506));
#26687=CARTESIAN_POINT('Ctrl Pts',(163.927102800511,-13.1362530473495,-10.224751619207));
#26688=CARTESIAN_POINT('Ctrl Pts',(163.966334076005,-11.2495841849556,-12.2700262932464));
#26689=CARTESIAN_POINT('Ctrl Pts',(164.0055653515,-8.99126846022917,-13.7470765539275));
#26690=CARTESIAN_POINT('Ctrl Pts',(164.044796626994,-6.73295273550269,-15.2241268146085));
#26691=CARTESIAN_POINT('Ctrl Pts',(164.084027902488,-4.10299014844364,-16.1329526619312));
#26692=CARTESIAN_POINT('Ctrl Pts',(164.123259177983,-1.41455789588256,-16.3653306787166));
#26693=CARTESIAN_POINT('Ctrl Pts',(164.162490453477,1.27387435667852,-16.5977086955021));
#26694=CARTESIAN_POINT('Ctrl Pts',(164.201721728972,4.02077627474165,-16.1536388817503));
#26695=CARTESIAN_POINT('Ctrl Pts',(164.240953004466,6.49904526210118,-15.0860012513868));
#26696=CARTESIAN_POINT('Ctrl Pts',(164.28018427996,8.97731424946063,-14.0183636210233));
#26697=CARTESIAN_POINT('Ctrl Pts',(164.319415555455,11.1869503061165,-12.3271581740481));
#26698=CARTESIAN_POINT('Ctrl Pts',(164.358646830949,12.8648291450421,-10.2137745900656));
#26699=CARTESIAN_POINT('Ctrl Pts',(164.397878106443,14.5427079839677,-8.10039100608284));
#26700=CARTESIAN_POINT('Ctrl Pts',(164.437109381938,15.688829605163,-5.5648292850926));
#26701=CARTESIAN_POINT('Ctrl Pts',(164.476340657432,16.1667126905997,-2.90902521091257));
#26702=CARTESIAN_POINT('Ctrl Pts',(164.515571932927,16.6445957760363,-0.253221136732651));
#26703=CARTESIAN_POINT('Ctrl Pts',(164.554803208421,16.4542403257145,2.52282529063697));
#26704=CARTESIAN_POINT('Ctrl Pts',(164.594034483915,15.6183151529188,5.08854070546535));
#26705=CARTESIAN_POINT('Ctrl Pts',(164.63326575941,14.782389980123,7.65425612029377));
#26706=CARTESIAN_POINT('Ctrl Pts',(164.672497034904,13.3008950848533,10.0096405225808));
#26707=CARTESIAN_POINT('Ctrl Pts',(164.711728310399,11.3502451796235,11.8742143043212));
#26708=CARTESIAN_POINT('Ctrl Pts',(164.750959585893,9.39959527439374,13.7387880860616));
#26709=CARTESIAN_POINT('Ctrl Pts',(164.790190861387,6.97979035920383,15.1125512472554));
#26710=CARTESIAN_POINT('Ctrl Pts',(164.829422136882,4.37898702814889,15.8319138469491));
#26711=CARTESIAN_POINT('Ctrl Pts',(164.868653412376,1.77818369709394,16.5512764466429));
#26712=CARTESIAN_POINT('Ctrl Pts',(164.907884687871,-1.00361804982606,16.6162384848367));
#26713=CARTESIAN_POINT('Ctrl Pts',(164.947115963365,-3.63517014472577,16.0190673975602));
#26714=CARTESIAN_POINT('Ctrl Pts',(164.986347238859,-6.26672223962549,15.4218963102837));
#26715=CARTESIAN_POINT('Ctrl Pts',(165.025578514354,-8.74802468250493,14.1625920975368));
#26716=CARTESIAN_POINT('Ctrl Pts',(165.064809789848,-10.7835816465719,12.3911068786316));
#26717=CARTESIAN_POINT('Ctrl Pts',(165.104041065343,-12.8191386106389,10.6196216597264));
#26718=CARTESIAN_POINT('Ctrl Pts',(165.143272340837,-14.4089500958934,8.33595543466287));
#26719=CARTESIAN_POINT('Ctrl Pts',(165.182503616331,-15.3637438128742,5.81206157253249));
#26720=CARTESIAN_POINT('Ctrl Pts',(165.211283461837,-16.0641751732649,3.96054707270523));
#26721=CARTESIAN_POINT('Ctrl Pts',(165.240063307342,-16.4228648636352,1.97975147559551));
#26722=CARTESIAN_POINT('Ctrl Pts',(165.268843152848,-16.4247445391107,-0.000389063610209933));
#26723=CARTESIAN_POINT('Origin',(147.227129595899,0.,0.));
#26724=CARTESIAN_POINT('',(164.477129595899,-15.5672291282746,1.73860745367607E-5));
#26725=CARTESIAN_POINT('',(164.772870404101,-15.5657079000652,-0.000368715050692581));
#26726=CARTESIAN_POINT('',(147.227129595899,-15.56595,-7.64522432085395E-13));
#26727=CARTESIAN_POINT('',(165.275,15.2541446685787,3.10078767190799));
#26728=CARTESIAN_POINT('Ctrl Pts',(164.477129595899,-15.5672291282746,1.73860745367725E-5));
#26729=CARTESIAN_POINT('Ctrl Pts',(164.516097891905,-15.5670581344026,-2.54016445452667));
#26730=CARTESIAN_POINT('Ctrl Pts',(164.594297463404,-14.293717715194,-7.63783591380272));
#26731=CARTESIAN_POINT('Ctrl Pts',(164.711728310399,-8.99354421585697,-13.4871293872258));
#26732=CARTESIAN_POINT('Ctrl Pts',(164.829422136882,-1.53958007844154,-16.1374149400877));
#26733=CARTESIAN_POINT('Ctrl Pts',(164.947115963365,6.2810321020304,-14.9443951095233));
#26734=CARTESIAN_POINT('Ctrl Pts',(165.064809789848,12.6057881822385,-10.1922081771534));
#26735=CARTESIAN_POINT('Ctrl Pts',(165.174104468727,15.6911477082268,-3.52499098687683));
#26736=CARTESIAN_POINT('Ctrl Pts',(165.24416787211,15.652577916973,1.13042150275773));
#26737=CARTESIAN_POINT('Ctrl Pts',(165.275,15.2541446685787,3.100787671908));
#26738=CARTESIAN_POINT('',(165.275,7.90291568084493,-13.4105452217259));
#26739=CARTESIAN_POINT('Origin',(165.275,0.,0.));
#26740=CARTESIAN_POINT('Ctrl Pts',(164.772870404101,-15.5657079000652,-0.000368715050694315));
#26741=CARTESIAN_POINT('Ctrl Pts',(164.78332183409,-15.5663548048828,-0.681849359511778));
#26742=CARTESIAN_POINT('Ctrl Pts',(164.833004539573,-15.3574419571854,-3.92099794181115));
#26743=CARTESIAN_POINT('Ctrl Pts',(164.92191852055,-13.1524493936104,-9.4760867792538));
#26744=CARTESIAN_POINT('Ctrl Pts',(165.039612347034,-7.10203868245562,-14.5722070548038));
#26745=CARTESIAN_POINT('Ctrl Pts',(165.157306173517,0.641239642833148,-16.1982319284135));
#26746=CARTESIAN_POINT('Ctrl Pts',(165.235768724506,5.69913956220702,-14.7092438620197));
#26747=CARTESIAN_POINT('Ctrl Pts',(165.275,7.90291568084474,-13.410545221726));
#26748=CARTESIAN_POINT('Origin',(147.227129595899,0.,0.));
#26749=CARTESIAN_POINT('',(162.977129595899,-15.5657179800606,0.000377847897364862));
#26750=CARTESIAN_POINT('',(163.272870404101,-15.5672257591788,-2.9359822512065E-5));
#26751=CARTESIAN_POINT('',(147.227129595899,-15.56595,-7.64522432085395E-13));
#26752=CARTESIAN_POINT('Ctrl Pts',(162.977129595899,-15.5657179800606,0.000377847897364836));
#26753=CARTESIAN_POINT('Ctrl Pts',(163.006091310478,-15.5639141968021,-1.88804632235174));
#26754=CARTESIAN_POINT('Ctrl Pts',(163.07428430055,-14.7531973033115,-6.33601965434617));
#26755=CARTESIAN_POINT('Ctrl Pts',(163.181708566117,-10.6140241611372,-12.2527121369471));
#26756=CARTESIAN_POINT('Ctrl Pts',(163.2994023926,-3.55130708784071,-15.8169112527338));
#26757=CARTESIAN_POINT('Ctrl Pts',(163.417096219084,4.35719284595873,-15.6141389170616));
#26758=CARTESIAN_POINT('Ctrl Pts',(163.534790045567,11.2279793567904,-11.692687592161));
#26759=CARTESIAN_POINT('Ctrl Pts',(163.65248387205,15.4246990473113,-4.9864940609672));
#26760=CARTESIAN_POINT('Ctrl Pts',(163.770177698533,15.9478569233932,2.90728790015858));
#26761=CARTESIAN_POINT('Ctrl Pts',(163.887871525016,12.672857226445,10.108667254542));
#26762=CARTESIAN_POINT('Ctrl Pts',(164.005565351499,6.37967707542191,14.902556282264));
#26763=CARTESIAN_POINT('Ctrl Pts',(164.123259177983,-1.43289323788845,16.1472375393268));
#26764=CARTESIAN_POINT('Ctrl Pts',(164.240953004466,-8.90420452717788,13.5462765378252));
#26765=CARTESIAN_POINT('Ctrl Pts',(164.358646830949,-14.2548809857467,7.71912065876858));
#26766=CARTESIAN_POINT('Ctrl Pts',(164.437372361427,-15.5630648054341,2.59162629500307));
#26767=CARTESIAN_POINT('Ctrl Pts',(164.47686661641,-15.5672302822353,0.0171599299072187));
#26768=CARTESIAN_POINT('Ctrl Pts',(164.477129595899,-15.5672291282746,1.73860745367725E-5));
#26769=CARTESIAN_POINT('Ctrl Pts',(163.272870404101,-15.5672257591788,-2.93598225131189E-5));
#26770=CARTESIAN_POINT('Ctrl Pts',(163.273315252662,-15.567229013186,-0.0290272128185329));
#26771=CARTESIAN_POINT('Ctrl Pts',(163.312991376719,-15.5601500968341,-2.61534939581951));
#26772=CARTESIAN_POINT('Ctrl Pts',(163.391898776269,-14.2372025145188,-7.75167909617249));
#26773=CARTESIAN_POINT('Ctrl Pts',(163.509592602752,-8.87322202528032,-13.5665911166955));
#26774=CARTESIAN_POINT('Ctrl Pts',(163.627286429235,-1.39598620207817,-16.1504701483178));
#26775=CARTESIAN_POINT('Ctrl Pts',(163.744980255718,6.413719352529,-14.8879370857845));
#26776=CARTESIAN_POINT('Ctrl Pts',(163.862674082202,12.6959265445113,-10.0796778296488));
#26777=CARTESIAN_POINT('Ctrl Pts',(163.980367908685,15.9544602156426,-2.87083272081841));
#26778=CARTESIAN_POINT('Ctrl Pts',(164.098061735168,15.4132614171153,5.0217334684266));
#26779=CARTESIAN_POINT('Ctrl Pts',(164.215755561651,11.2012293687092,11.7183171829071));
#26780=CARTESIAN_POINT('Ctrl Pts',(164.333449388134,4.32149195873656,15.6240575808949));
#26781=CARTESIAN_POINT('Ctrl Pts',(164.451143214618,-3.58743715586971,15.8087508847164));
#26782=CARTESIAN_POINT('Ctrl Pts',(164.568837041101,-10.6420179340868,12.2284282526787));
#26783=CARTESIAN_POINT('Ctrl Pts',(164.676079437595,-14.7606212533428,6.31230839705082));
#26784=CARTESIAN_POINT('Ctrl Pts',(164.744090558595,-15.563926534192,1.87620776143336));
#26785=CARTESIAN_POINT('Ctrl Pts',(164.772870404101,-15.5657079000652,-0.000368715050694315));
#26786=CARTESIAN_POINT('Origin',(147.227129595899,0.,0.));
#26787=CARTESIAN_POINT('',(161.477129595899,-15.5646934397166,-3.82463327799083E-5));
#26788=CARTESIAN_POINT('',(161.772870404101,-15.5658554189301,0.000381071499603314));
#26789=CARTESIAN_POINT('',(147.227129595899,-15.56595,-7.64522432085395E-13));
#26790=CARTESIAN_POINT('Ctrl Pts',(161.477129595899,-15.5646934397166,-3.82463327805449E-5));
#26791=CARTESIAN_POINT('Ctrl Pts',(161.49608472905,-15.5648016885781,-1.23622519836749));
#26792=CARTESIAN_POINT('Ctrl Pts',(161.554271137696,-15.1179460024313,-5.03086065784982));
#26793=CARTESIAN_POINT('Ctrl Pts',(161.651688821836,-12.0668967458695,-10.8248079212624));
#26794=CARTESIAN_POINT('Ctrl Pts',(161.769382648319,-5.50694958937003,-15.2466379844161));
#26795=CARTESIAN_POINT('Ctrl Pts',(161.887076474802,2.3645382059743,-16.0373134495834));
#26796=CARTESIAN_POINT('Ctrl Pts',(162.004770301285,9.67288521004985,-13.0085262547648));
#26797=CARTESIAN_POINT('Ctrl Pts',(162.122464127768,14.67752816854,-6.88161539679513));
#26798=CARTESIAN_POINT('Ctrl Pts',(162.240157954252,16.1865562937323,0.884227887797634));
#26799=CARTESIAN_POINT('Ctrl Pts',(162.357851780735,13.840577933451,8.43948257156437));
#26800=CARTESIAN_POINT('Ctrl Pts',(162.475545607218,8.19831364750381,13.9847816194923));
#26801=CARTESIAN_POINT('Ctrl Pts',(162.593239433701,0.603530758605001,16.1994510472156));
#26802=CARTESIAN_POINT('Ctrl Pts',(162.710933260184,-7.13498962120933,14.5560429620394));
#26803=CARTESIAN_POINT('Ctrl Pts',(162.828627086668,-13.1742337149738,9.44595308222564));
#26804=CARTESIAN_POINT('Ctrl Pts',(162.917359198573,-15.361859159625,3.89726831243747));
#26805=CARTESIAN_POINT('Ctrl Pts',(162.966860034983,-15.5663575852194,0.669995905194144));
#26806=CARTESIAN_POINT('Ctrl Pts',(162.977129595899,-15.5657179800606,0.000377847897364836));
#26807=CARTESIAN_POINT('Ctrl Pts',(161.772870404101,-15.5658554189301,0.000381071499603106));
#26808=CARTESIAN_POINT('Ctrl Pts',(161.80253994673,-15.5639605892315,-1.93414728096267));
#26809=CARTESIAN_POINT('Ctrl Pts',(161.871440764853,-14.7238756891141,-6.42825297656992));
#26810=CARTESIAN_POINT('Ctrl Pts',(161.979572858471,-10.5046199403779,-12.3466361338107));
#26811=CARTESIAN_POINT('Ctrl Pts',(162.097266684954,-3.41047972870878,-15.8478734198804));
#26812=CARTESIAN_POINT('Ctrl Pts',(162.214960511437,4.49590375656297,-15.5747652734798));
#26813=CARTESIAN_POINT('Ctrl Pts',(162.33265433792,11.3315382928711,-11.5923554047623));
#26814=CARTESIAN_POINT('Ctrl Pts',(162.450348164404,15.4684423013133,-4.84909854322174));
#26815=CARTESIAN_POINT('Ctrl Pts',(162.568041990887,15.9213665733349,3.04902449198908));
#26816=CARTESIAN_POINT('Ctrl Pts',(162.68573581737,12.5824422093376,10.2209887954907));
#26817=CARTESIAN_POINT('Ctrl Pts',(162.803429643853,6.24687078672089,14.9587121533836));
#26818=CARTESIAN_POINT('Ctrl Pts',(162.921123470336,-1.57646165108159,16.1338536185746));
#26819=CARTESIAN_POINT('Ctrl Pts',(163.038817296819,-9.02434239708718,13.466540319226));
#26820=CARTESIAN_POINT('Ctrl Pts',(163.156066274741,-14.3029494091455,7.61422624586815));
#26821=CARTESIAN_POINT('Ctrl Pts',(163.234083977168,-15.5669420417053,2.52829871263177));
#26822=CARTESIAN_POINT('Ctrl Pts',(163.272870404101,-15.5672257591788,-2.93598225131189E-5));
#26823=CARTESIAN_POINT('Origin',(147.227129595899,0.,0.));
#26824=CARTESIAN_POINT('',(159.977129595899,-15.5659766626728,-0.000379993813608694));
#26825=CARTESIAN_POINT('',(160.272870404101,-15.564687658505,2.74468699046349E-6));
#26826=CARTESIAN_POINT('',(147.227129595899,-15.56595,-7.64522432085395E-13));
#26827=CARTESIAN_POINT('Ctrl Pts',(159.977129595899,-15.5659766626728,-0.000379993813609536));
#26828=CARTESIAN_POINT('Ctrl Pts',(159.986078147623,-15.5665555132718,-0.583834849331341));
#26829=CARTESIAN_POINT('Ctrl Pts',(160.034257974841,-15.3932425959096,-3.72486762104057));
#26830=CARTESIAN_POINT('Ctrl Pts',(160.121669077554,-13.3292169161666,-9.22596553264098));
#26831=CARTESIAN_POINT('Ctrl Pts',(160.239362904037,-7.37563000308724,-14.4355999413));
#26832=CARTESIAN_POINT('Ctrl Pts',(160.357056730521,0.334544350851575,-16.2072373859648));
#26833=CARTESIAN_POINT('Ctrl Pts',(160.474750557004,7.96504328657251,-14.1189429154851));
#26834=CARTESIAN_POINT('Ctrl Pts',(160.592444383487,13.6985795225324,-8.66806683595355));
#26835=CARTESIAN_POINT('Ctrl Pts',(160.71013820997,16.1696483168198,-1.15279526285827));
#26836=CARTESIAN_POINT('Ctrl Pts',(160.827832036453,14.7897374463801,6.6370271865379));
#26837=CARTESIAN_POINT('Ctrl Pts',(160.945525862937,9.88748786846115,12.8461685828396));
#26838=CARTESIAN_POINT('Ctrl Pts',(161.06321968942,2.63042426053809,15.9958535820154));
#26839=CARTESIAN_POINT('Ctrl Pts',(161.180913515903,-5.25310382814925,15.3359500448582));
#26840=CARTESIAN_POINT('Ctrl Pts',(161.298607342386,-11.8855474391451,11.0236212598008));
#26841=CARTESIAN_POINT('Ctrl Pts',(161.397346035718,-15.0750246160597,5.20324843830764));
#26842=CARTESIAN_POINT('Ctrl Pts',(161.456853453556,-15.5645776468435,1.32230026759633));
#26843=CARTESIAN_POINT('Ctrl Pts',(161.477129595899,-15.5646934397166,-3.82463327805449E-5));
#26844=CARTESIAN_POINT('Ctrl Pts',(160.272870404101,-15.564687658505,2.74468699018593E-6));
#26845=CARTESIAN_POINT('Ctrl Pts',(160.292533365303,-15.5646796038872,-1.28234762386084));
#26846=CARTESIAN_POINT('Ctrl Pts',(160.351427601999,-15.095142128267,-5.12323198115841));
#26847=CARTESIAN_POINT('Ctrl Pts',(160.449553114189,-11.9701358491835,-10.9317112871024));
#26848=CARTESIAN_POINT('Ctrl Pts',(160.567246940672,-5.37111728571021,-15.2950175879472));
#26849=CARTESIAN_POINT('Ctrl Pts',(160.684940767156,2.50709195889985,-16.0156471558938));
#26850=CARTESIAN_POINT('Ctrl Pts',(160.802634593639,9.78820966743234,-12.9219741300954));
#26851=CARTESIAN_POINT('Ctrl Pts',(160.920328420122,14.7381575419149,-6.75079078198745));
#26852=CARTESIAN_POINT('Ctrl Pts',(161.038022246605,16.1780510307112,1.02816767123628));
#26853=CARTESIAN_POINT('Ctrl Pts',(161.155716073088,13.7649636560103,8.56225668040771));
#26854=CARTESIAN_POINT('Ctrl Pts',(161.273409899572,8.07359872781038,14.0571500488103));
#26855=CARTESIAN_POINT('Ctrl Pts',(161.391103726055,0.459417427060223,16.2041784592796));
#26856=CARTESIAN_POINT('Ctrl Pts',(161.508797552538,-7.2641791890122,14.4920034716527));
#26857=CARTESIAN_POINT('Ctrl Pts',(161.626491379021,-13.2577316019136,9.32839839865786));
#26858=CARTESIAN_POINT('Ctrl Pts',(161.714515662875,-15.3788599629686,3.80489090455934));
#26859=CARTESIAN_POINT('Ctrl Pts',(161.763308671235,-15.5664660739587,0.623829958404114));
#26860=CARTESIAN_POINT('Ctrl Pts',(161.772870404101,-15.5658554189301,0.000381071499603106));
#26861=CARTESIAN_POINT('Origin',(147.227129595899,0.,0.));
#26862=CARTESIAN_POINT('',(158.477129595899,-15.5672032398919,6.94315363263075E-5));
#26863=CARTESIAN_POINT('',(158.772870404101,-15.5658368563573,-0.000380915866178277));
#26864=CARTESIAN_POINT('',(147.227129595899,-15.56595,-7.64522432085395E-13));
#26865=CARTESIAN_POINT('Ctrl Pts',(158.477129595899,-15.5672032398919,6.94315363258292E-5));
#26866=CARTESIAN_POINT('Ctrl Pts',(158.51530284169,-15.5665698359374,-2.48829837233368));
#26867=CARTESIAN_POINT('Ctrl Pts',(158.592707362976,-14.3338262659127,-7.5346083212108));
#26868=CARTESIAN_POINT('Ctrl Pts',(158.709343159756,-9.12783936934241,-13.3966044972293));
#26869=CARTESIAN_POINT('Ctrl Pts',(158.827036986239,-1.70073240633521,-16.1212274002243));
#26870=CARTESIAN_POINT('Ctrl Pts',(158.944730812722,6.13142269276078,-15.0064026125651));
#26871=CARTESIAN_POINT('Ctrl Pts',(159.062424639206,12.503312012229,-10.3176379240867));
#26872=CARTESIAN_POINT('Ctrl Pts',(159.180118465689,15.8973999993859,-3.17161423682451));
#26873=CARTESIAN_POINT('Ctrl Pts',(159.297812292172,15.5053472542187,4.7297642788828));
#26874=CARTESIAN_POINT('Ctrl Pts',(159.415506118655,11.4205254518286,11.5046973889728));
#26875=CARTESIAN_POINT('Ctrl Pts',(159.533199945138,4.61577985061722,15.5396602272488));
#26876=CARTESIAN_POINT('Ctrl Pts',(159.650893771622,-3.28826451042518,15.8736819962219));
#26877=CARTESIAN_POINT('Ctrl Pts',(159.768587598105,-10.4091724968367,12.4272117362987));
#26878=CARTESIAN_POINT('Ctrl Pts',(159.877332872864,-14.698090296236,6.5081394447137));
#26879=CARTESIAN_POINT('Ctrl Pts',(159.946846872129,-15.5640177788966,1.97408501093939));
#26880=CARTESIAN_POINT('Ctrl Pts',(159.977129595899,-15.5659766626728,-0.000379993813609536));
#26881=CARTESIAN_POINT('Ctrl Pts',(158.772870404101,-15.5658368563573,-0.000380915866179943));
#26882=CARTESIAN_POINT('Ctrl Pts',(158.782526783875,-15.5664518834751,-0.630003179149869));
#26883=CARTESIAN_POINT('Ctrl Pts',(158.831414439144,-15.376611447023,-3.81724297589167));
#26884=CARTESIAN_POINT('Ctrl Pts',(158.919533369908,-13.2466273275316,-9.34416012052252));
#26885=CARTESIAN_POINT('Ctrl Pts',(159.037227196391,-7.24693772795856,-14.5006330027196));
#26886=CARTESIAN_POINT('Ctrl Pts',(159.154921022874,0.478689831123546,-16.2036205817727));
#26887=CARTESIAN_POINT('Ctrl Pts',(159.272614849357,8.0903121397976,-14.0475376273962));
#26888=CARTESIAN_POINT('Ctrl Pts',(159.390308675841,13.7751375929553,-8.54587901901382));
#26889=CARTESIAN_POINT('Ctrl Pts',(159.508002502324,16.1792624575846,-1.00892529013043));
#26890=CARTESIAN_POINT('Ctrl Pts',(159.625696328807,14.7301179440772,6.76831509801693));
#26891=CARTESIAN_POINT('Ctrl Pts',(159.74339015529,9.77283376357005,12.9336067723623));
#26892=CARTESIAN_POINT('Ctrl Pts',(159.861083981773,2.48804168970207,16.0186176826459));
#26893=CARTESIAN_POINT('Ctrl Pts',(159.978777808256,-5.3893048890199,15.2886185355531));
#26894=CARTESIAN_POINT('Ctrl Pts',(160.09647163474,-11.9831292087549,10.9174666602997));
#26895=CARTESIAN_POINT('Ctrl Pts',(160.194502500021,-15.0982173014888,5.11088082725593));
#26896=CARTESIAN_POINT('Ctrl Pts',(160.253302089808,-15.5646956743521,1.27618056895072));
#26897=CARTESIAN_POINT('Ctrl Pts',(160.272870404101,-15.564687658505,2.74468699018593E-6));
#26898=CARTESIAN_POINT('Origin',(147.227129595899,0.,0.));
#26899=CARTESIAN_POINT('',(156.977129595899,-15.5655685625645,0.000368663249558582));
#26900=CARTESIAN_POINT('',(157.272870404101,-15.5672276545898,2.31237102392076E-5));
#26901=CARTESIAN_POINT('',(147.227129595899,-15.56595,-7.64522432085395E-13));
#26902=CARTESIAN_POINT('Ctrl Pts',(156.977129595899,-15.5655685625645,0.000368663249558365));
#26903=CARTESIAN_POINT('Ctrl Pts',(157.005296260263,-15.5638856278198,-1.83626562325807));
#26904=CARTESIAN_POINT('Ctrl Pts',(157.072694200122,-14.7855673246138,-6.23240172064292));
#26905=CARTESIAN_POINT('Ctrl Pts',(157.179323415475,-10.7359079622712,-12.1460587777823));
#26906=CARTESIAN_POINT('Ctrl Pts',(157.297017241958,-3.70915232759935,-15.780641704898));
#26907=CARTESIAN_POINT('Ctrl Pts',(157.414711068441,4.20097874648159,-15.6568911722382));
#26908=CARTESIAN_POINT('Ctrl Pts',(157.532404894924,11.1106005078261,-11.8042797308094));
#26909=CARTESIAN_POINT('Ctrl Pts',(157.650098721407,15.3741105059335,-5.14034918648998));
#26910=CARTESIAN_POINT('Ctrl Pts',(157.76779254789,15.976106922448,2.74781207694638));
#26911=CARTESIAN_POINT('Ctrl Pts',(157.885486374374,12.7732176868821,9.98155165949782));
#26912=CARTESIAN_POINT('Ctrl Pts',(158.003180200857,6.52824611275682,14.8380748852059));
#26913=CARTESIAN_POINT('Ctrl Pts',(158.12087402734,-1.27149910480069,16.1607473105111));
#26914=CARTESIAN_POINT('Ctrl Pts',(158.238567853823,-8.76842281997508,13.6345599436814));
#26915=CARTESIAN_POINT('Ctrl Pts',(158.356261680306,-14.1770501597529,7.86115210230364));
#26916=CARTESIAN_POINT('Ctrl Pts',(158.435782260998,-15.5501236141346,2.69533522288462));
#26917=CARTESIAN_POINT('Ctrl Pts',(158.476071566196,-15.5672207956481,0.069038338801308));
#26918=CARTESIAN_POINT('Ctrl Pts',(158.477129595899,-15.5672032398919,6.94315363258292E-5));
#26919=CARTESIAN_POINT('Ctrl Pts',(157.272870404101,-15.5672276545898,2.31237102390775E-5));
#26920=CARTESIAN_POINT('Ctrl Pts',(157.311751477943,-15.5670021417586,-2.53447369309111));
#26921=CARTESIAN_POINT('Ctrl Pts',(157.389863827279,-14.2981498398272,-7.6265132345712));
#26922=CARTESIAN_POINT('Ctrl Pts',(157.507207452109,-9.00831934563013,-13.4772640576497));
#26923=CARTESIAN_POINT('Ctrl Pts',(157.624901278593,-1.55727144834802,-16.135717199698));
#26924=CARTESIAN_POINT('Ctrl Pts',(157.742595105076,6.26465777934683,-14.9512717459131));
#26925=CARTESIAN_POINT('Ctrl Pts',(157.860288931559,12.5945898255295,-10.2060164138188));
#26926=CARTESIAN_POINT('Ctrl Pts',(157.977982758042,15.9249817238141,-3.03008597380632));
#26927=CARTESIAN_POINT('Ctrl Pts',(158.095676584526,15.4626639986145,4.86749278154799));
#26928=CARTESIAN_POINT('Ctrl Pts',(158.213370411009,11.3177427031671,11.6058245729193));
#26929=CARTESIAN_POINT('Ctrl Pts',(158.331064237492,4.47737645143262,15.5801015408959));
#26930=CARTESIAN_POINT('Ctrl Pts',(158.448758063975,-3.42932626773513,15.8438058957402));
#26931=CARTESIAN_POINT('Ctrl Pts',(158.566451890458,-10.5192972026361,12.3341335437509));
#26932=CARTESIAN_POINT('Ctrl Pts',(158.674489337167,-14.7278239251552,6.41592101404979));
#26933=CARTESIAN_POINT('Ctrl Pts',(158.743295508381,-15.5639531936083,1.92798284095932));
#26934=CARTESIAN_POINT('Ctrl Pts',(158.772870404101,-15.5658368563573,-0.000380915866179943));
#26935=CARTESIAN_POINT('Origin',(147.227129595899,0.,0.));
#26936=CARTESIAN_POINT('',(155.477129595899,-15.56471582026,-8.37554675685322E-5));
#26937=CARTESIAN_POINT('',(155.772870404101,-15.5657013094872,0.000377124385127214));
#26938=CARTESIAN_POINT('',(147.227129595899,-15.56595,-7.64522432085395E-13));
#26939=CARTESIAN_POINT('Ctrl Pts',(155.477129595899,-15.56471582026,-8.37554675685304E-5));
#26940=CARTESIAN_POINT('Ctrl Pts',(155.495289678836,-15.5649433446237,-1.18441545923554));
#26941=CARTESIAN_POINT('Ctrl Pts',(155.552681037267,-15.1430267377089,-4.92710253995072));
#26942=CARTESIAN_POINT('Ctrl Pts',(155.649303671193,-12.1744422313121,-10.703710569898));
#26943=CARTESIAN_POINT('Ctrl Pts',(155.766997497676,-5.65899978025936,-15.1908586029469));
#26944=CARTESIAN_POINT('Ctrl Pts',(155.884691324159,2.20419573563924,-16.0601365114588));
#26945=CARTESIAN_POINT('Ctrl Pts',(156.002385150643,9.54243778386128,-13.104516196672));
#26946=CARTESIAN_POINT('Ctrl Pts',(156.120078977126,14.6080432763861,-7.02791115787139));
#26947=CARTESIAN_POINT('Ctrl Pts',(156.237772803609,16.1945825272352,0.72246825277614));
#26948=CARTESIAN_POINT('Ctrl Pts',(156.355466630092,13.9242037567905,8.30078389955334));
#26949=CARTESIAN_POINT('Ctrl Pts',(156.473160456575,8.3376226506933,13.9021765253628));
#26950=CARTESIAN_POINT('Ctrl Pts',(156.590854283059,0.765344969699789,16.1926128430546));
#26951=CARTESIAN_POINT('Ctrl Pts',(156.708548109542,-6.9892080370811,14.626600241413));
#26952=CARTESIAN_POINT('Ctrl Pts',(156.826241936025,-13.0792042460899,9.5771018526883));
#26953=CARTESIAN_POINT('Ctrl Pts',(156.915769098144,-15.3422530299605,4.00103142563335));
#26954=CARTESIAN_POINT('Ctrl Pts',(156.966064984769,-15.5662296638674,0.72184721343301));
#26955=CARTESIAN_POINT('Ctrl Pts',(156.977129595899,-15.5655685625645,0.000368663249558365));
#26956=CARTESIAN_POINT('Ctrl Pts',(155.772870404101,-15.5657013094872,0.000377124385127978));
#26957=CARTESIAN_POINT('Ctrl Pts',(155.801744896515,-15.563909886075,-1.88236560251977));
#26958=CARTESIAN_POINT('Ctrl Pts',(155.869850664425,-14.7567776476042,-6.3246530627241));
#26959=CARTESIAN_POINT('Ctrl Pts',(155.977187707828,-10.6274475707617,-12.2410711150283));
#26960=CARTESIAN_POINT('Ctrl Pts',(156.094881534311,-3.56864133200721,-15.8130092947535));
#26961=CARTESIAN_POINT('Ctrl Pts',(156.212575360794,4.34007610648377,-15.6189053170316));
#26962=CARTESIAN_POINT('Ctrl Pts',(156.330269187278,11.215156665436,-11.7049871799245));
#26963=CARTESIAN_POINT('Ctrl Pts',(156.447963013761,15.4192242617626,-5.00339755345713));
#26964=CARTESIAN_POINT('Ctrl Pts',(156.565656840244,15.9510339391494,2.88980625381255));
#26965=CARTESIAN_POINT('Ctrl Pts',(156.683350666727,12.6839293713117,10.0947709045845));
#26966=CARTESIAN_POINT('Ctrl Pts',(156.80104449321,6.39600745972602,14.8955547895202));
#26967=CARTESIAN_POINT('Ctrl Pts',(156.918738319694,-1.41519400502264,16.1487984023771));
#26968=CARTESIAN_POINT('Ctrl Pts',(157.036432146177,-8.88935144579475,13.5560279870475));
#26969=CARTESIAN_POINT('Ctrl Pts',(157.15412597266,-14.246412028328,7.7347403467461));
#26970=CARTESIAN_POINT('Ctrl Pts',(157.232938725301,-15.5616701988428,2.60300355025934));
#26971=CARTESIAN_POINT('Ctrl Pts',(157.272520202448,-15.5672296857829,0.0228513248357287));
#26972=CARTESIAN_POINT('Ctrl Pts',(157.272870404101,-15.5672276545898,2.31237102390775E-5));
#26973=CARTESIAN_POINT('Origin',(147.227129595899,0.,0.));
#26974=CARTESIAN_POINT('',(153.977129595899,-15.56613520909,-0.000373169223084742));
#26975=CARTESIAN_POINT('',(154.272870404101,-15.5646950861503,-4.32770794628334E-5));
#26976=CARTESIAN_POINT('',(147.227129595899,-15.56595,-7.64522432085395E-13));
#26977=CARTESIAN_POINT('Ctrl Pts',(153.977129595899,-15.56613520909,-0.000373169223085931));
#26978=CARTESIAN_POINT('Ctrl Pts',(153.985283097409,-15.5666647118316,-0.531974321578409));
#26979=CARTESIAN_POINT('Ctrl Pts',(154.032667874413,-15.4114159073324,-3.62111245429205));
#26980=CARTESIAN_POINT('Ctrl Pts',(154.119283926912,-13.4207257992801,-9.09233647794895));
#26981=CARTESIAN_POINT('Ctrl Pts',(154.236977753395,-7.51948406913288,-14.3611915571709));
#26982=CARTESIAN_POINT('Ctrl Pts',(154.354671579878,0.172605530559356,-16.2097708478104));
#26983=CARTESIAN_POINT('Ctrl Pts',(154.472365406361,7.82358722393355,-14.1978148514905));
#26984=CARTESIAN_POINT('Ctrl Pts',(154.590059232844,13.6112955353353,-8.80449302671448));
#26985=CARTESIAN_POINT('Ctrl Pts',(154.707753059327,16.1573240470198,-1.31428430991864));
#26986=CARTESIAN_POINT('Ctrl Pts',(154.825446885811,14.8553080544366,6.48893567663383));
#26987=CARTESIAN_POINT('Ctrl Pts',(154.943140712294,10.0153369925782,12.7467442326578));
#26988=CARTESIAN_POINT('Ctrl Pts',(155.060834538777,2.79010322505614,15.968775394539));
#26989=CARTESIAN_POINT('Ctrl Pts',(155.17852836526,-5.09962432561176,15.3876669883817));
#26990=CARTESIAN_POINT('Ctrl Pts',(155.296222191744,-11.7748202308851,11.1418163751715));
#26991=CARTESIAN_POINT('Ctrl Pts',(155.39575593529,-15.0484368117828,5.30699215271008));
#26992=CARTESIAN_POINT('Ctrl Pts',(155.456058403342,-15.5644518231355,1.37409947204133));
#26993=CARTESIAN_POINT('Ctrl Pts',(155.477129595899,-15.56471582026,-8.37554675685304E-5));
#26994=CARTESIAN_POINT('Ctrl Pts',(154.272870404101,-15.5646950861503,-4.32770794628334E-5));
#26995=CARTESIAN_POINT('Ctrl Pts',(154.291738315088,-15.5648170261259,-1.23054153718203));
#26996=CARTESIAN_POINT('Ctrl Pts',(154.34983750157,-15.1207250389303,-5.01947793156282));
#26997=CARTESIAN_POINT('Ctrl Pts',(154.447167963547,-12.0787542064295,-10.8115753122814));
#26998=CARTESIAN_POINT('Ctrl Pts',(154.56486179003,-5.52365760332652,-15.2405928557154));
#26999=CARTESIAN_POINT('Ctrl Pts',(154.682555616513,2.34695883598703,-16.039895515079));
#27000=CARTESIAN_POINT('Ctrl Pts',(154.800249442996,9.65862120442349,-13.0191205671478));
#27001=CARTESIAN_POINT('Ctrl Pts',(154.917943269479,14.6699766571649,-6.8976988040002));
#27002=CARTESIAN_POINT('Ctrl Pts',(155.035637095963,16.1875157521321,0.86648582616573));
#27003=CARTESIAN_POINT('Ctrl Pts',(155.153330922446,13.8498198560533,8.4243073227026));
#27004=CARTESIAN_POINT('Ctrl Pts',(155.271024748929,8.21363696874461,13.9757873358942));
#27005=CARTESIAN_POINT('Ctrl Pts',(155.388718575412,0.621286060936392,16.1987798164848));
#27006=CARTESIAN_POINT('Ctrl Pts',(155.506412401895,-7.11903095842639,14.563854645163));
#27007=CARTESIAN_POINT('Ctrl Pts',(155.624106228379,-13.1638724228295,9.4603872409082));
#27008=CARTESIAN_POINT('Ctrl Pts',(155.712925562447,-15.3597346541413,3.90865167943404));
#27009=CARTESIAN_POINT('Ctrl Pts',(155.762513621021,-15.5663438622087,0.675684511174927));
#27010=CARTESIAN_POINT('Ctrl Pts',(155.772870404101,-15.5657013094872,0.000377124385127978));
#27011=CARTESIAN_POINT('Origin',(147.227129595899,0.,0.));
#27012=CARTESIAN_POINT('',(152.477129595899,-15.5671496799154,0.000119929893292461));
#27013=CARTESIAN_POINT('',(152.772870404101,-15.5659940241253,-0.000379545266269155));
#27014=CARTESIAN_POINT('',(147.227129595899,-15.56595,-7.64522432085395E-13));
#27015=CARTESIAN_POINT('Ctrl Pts',(152.477129595899,-15.5671496799154,0.000119929893292372));
#27016=CARTESIAN_POINT('Ctrl Pts',(152.514507791476,-15.566130228717,-2.43644601235259));
#27017=CARTESIAN_POINT('Ctrl Pts',(152.591117262548,-14.3733013902904,-7.43133785604296));
#27018=CARTESIAN_POINT('Ctrl Pts',(152.706958009113,-9.26122566274478,-13.3047421182903));
#27019=CARTESIAN_POINT('Ctrl Pts',(152.824651835596,-1.8617103463467,-16.1034312552471));
#27020=CARTESIAN_POINT('Ctrl Pts',(152.94234566208,5.98119177380371,-15.0669110494933));
#27021=CARTESIAN_POINT('Ctrl Pts',(153.060039488563,12.3996072607107,-10.44204019278));
#27022=CARTESIAN_POINT('Ctrl Pts',(153.177733315046,15.86491984296,-3.3302825682171));
#27023=CARTESIAN_POINT('Ctrl Pts',(153.295427141529,15.551827199527,4.5746184937969));
#27024=CARTESIAN_POINT('Ctrl Pts',(153.413120968012,11.5348957884658,11.3900238260024));
#27025=CARTESIAN_POINT('Ctrl Pts',(153.530814794496,4.77080202447272,15.4927696571985));
#27026=CARTESIAN_POINT('Ctrl Pts',(153.648508620979,-3.12951073579735,15.9057419242933));
#27027=CARTESIAN_POINT('Ctrl Pts',(153.766202447462,-10.2844960796655,12.5305867378607));
#27028=CARTESIAN_POINT('Ctrl Pts',(153.875742772435,-14.6641232704987,6.61169964040524));
#27029=CARTESIAN_POINT('Ctrl Pts',(153.946051821915,-15.5641169637375,2.02587045667698));
#27030=CARTESIAN_POINT('Ctrl Pts',(153.977129595899,-15.56613520909,-0.000373169223085931));
#27031=CARTESIAN_POINT('Ctrl Pts',(152.772870404101,-15.5659940241253,-0.000379545266269155));
#27032=CARTESIAN_POINT('Ctrl Pts',(152.781731733661,-15.5665678851702,-0.578145570173576));
#27033=CARTESIAN_POINT('Ctrl Pts',(152.829824338716,-15.3952625119623,-3.71348484017464));
#27034=CARTESIAN_POINT('Ctrl Pts',(152.917148219265,-13.3393211827226,-9.21135029713916));
#27035=CARTESIAN_POINT('Ctrl Pts',(153.034842045748,-7.39144794457472,-14.4275071025847));
#27036=CARTESIAN_POINT('Ctrl Pts',(153.152535872232,0.316779951246796,-16.2075943426206));
#27037=CARTESIAN_POINT('Ctrl Pts',(153.270229698715,7.94956321608139,-14.1276646543581));
#27038=CARTESIAN_POINT('Ctrl Pts',(153.387923525198,13.689070530273,-8.68307617896328));
#27039=CARTESIAN_POINT('Ctrl Pts',(153.505617351681,16.1683750739281,-1.17051756981636));
#27040=CARTESIAN_POINT('Ctrl Pts',(153.623311178164,14.7970031896607,6.62081267803603));
#27041=CARTESIAN_POINT('Ctrl Pts',(153.741005004647,9.90156218120505,12.8353235364053));
#27042=CARTESIAN_POINT('Ctrl Pts',(153.858698831131,2.64795519030276,15.9929608647873));
#27043=CARTESIAN_POINT('Ctrl Pts',(153.976392657614,-5.23629146518378,15.3416985892734));
#27044=CARTESIAN_POINT('Ctrl Pts',(154.094086484097,-11.8734576922091,11.0366419867544));
#27045=CARTESIAN_POINT('Ctrl Pts',(154.192912399593,-15.0721355684421,5.21463012093322));
#27046=CARTESIAN_POINT('Ctrl Pts',(154.252507039594,-15.5645634813227,1.32798315955527));
#27047=CARTESIAN_POINT('Ctrl Pts',(154.272870404101,-15.5646950861503,-4.32770794628334E-5));
#27048=CARTESIAN_POINT('Origin',(147.227129595899,0.,0.));
#27049=CARTESIAN_POINT('',(150.977129595899,-15.5654260231298,0.00035522955525607));
#27050=CARTESIAN_POINT('',(151.272870404101,-15.5671986622434,7.50751021387497E-5));
#27051=CARTESIAN_POINT('',(147.227129595899,-15.56595,-7.64522432085395E-13));
#27052=CARTESIAN_POINT('Ctrl Pts',(150.977129595899,-15.5654260231298,0.000355229555255854));
#27053=CARTESIAN_POINT('Ctrl Pts',(151.004501210049,-15.563880046197,-1.78448425824574));
#27054=CARTESIAN_POINT('Ctrl Pts',(151.071104099693,-14.8173427789448,-6.12876694614427));
#27055=CARTESIAN_POINT('Ctrl Pts',(151.176938264832,-10.8567200010544,-12.0381919340435));
#27056=CARTESIAN_POINT('Ctrl Pts',(151.294632091315,-3.86662739613892,-15.7427975140589));
#27057=CARTESIAN_POINT('Ctrl Pts',(151.412325917798,4.04434534995169,-15.6980803397344));
#27058=CARTESIAN_POINT('Ctrl Pts',(151.530019744281,10.9921126129483,-11.9146937268782));
#27059=CARTESIAN_POINT('Ctrl Pts',(151.647713570765,15.3219873755107,-5.293691155264));
#27060=CARTESIAN_POINT('Ctrl Pts',(151.765407397248,16.0027622209035,2.58806194553672));
#27061=CARTESIAN_POINT('Ctrl Pts',(151.883101223731,12.8723031774915,9.8534397471975));
#27062=CARTESIAN_POINT('Ctrl Pts',(152.000795050214,6.67616348792316,14.772112390107));
#27063=CARTESIAN_POINT('Ctrl Pts',(152.118488876698,-1.1099779917617,16.1726439575597));
#27064=CARTESIAN_POINT('Ctrl Pts',(152.23618270318,-8.63176600122648,13.7214824003989));
#27065=CARTESIAN_POINT('Ctrl Pts',(152.353876529664,-14.0978039594459,8.00239883654923));
#27066=CARTESIAN_POINT('Ctrl Pts',(152.43419216057,-15.5366625291471,2.79904944997984));
#27067=CARTESIAN_POINT('Ctrl Pts',(152.475276515982,-15.5672002207324,0.120916328577713));
#27068=CARTESIAN_POINT('Ctrl Pts',(152.477129595899,-15.5671496799154,0.000119929893292372));
#27069=CARTESIAN_POINT('Ctrl Pts',(151.272870404101,-15.5671986622434,7.50751021387757E-5));
#27070=CARTESIAN_POINT('Ctrl Pts',(151.310956427728,-15.5665192742014,-2.48260917620549));
#27071=CARTESIAN_POINT('Ctrl Pts',(151.38827372685,-14.3381877797512,-7.52328095819091));
#27072=CARTESIAN_POINT('Ctrl Pts',(151.504822301467,-9.14251744982534,-13.3865917383038));
#27073=CARTESIAN_POINT('Ctrl Pts',(151.62251612795,-1.71840131299559,-16.1193536145945));
#27074=CARTESIAN_POINT('Ctrl Pts',(151.740209954433,6.11497100889316,-15.0131140483778));
#27075=CARTESIAN_POINT('Ctrl Pts',(151.857903780916,12.491995698527,-10.3313361861333));
#27076=CARTESIAN_POINT('Ctrl Pts',(151.9755976074,15.8939141615272,-3.18903692982364));
#27077=CARTESIAN_POINT('Ctrl Pts',(152.093291433883,15.510522082331,4.71276655929273));
#27078=CARTESIAN_POINT('Ctrl Pts',(152.210985260366,11.4331285039078,11.4921728375615));
#27079=CARTESIAN_POINT('Ctrl Pts',(152.328679086849,4.63280957101442,15.5345917033455));
#27080=CARTESIAN_POINT('Ctrl Pts',(152.446372913332,-3.2708639369447,15.8772766247591));
#27081=CARTESIAN_POINT('Ctrl Pts',(152.564066739816,-10.3955452083385,12.4386134168428));
#27082=CARTESIAN_POINT('Ctrl Pts',(152.672899236738,-14.6943933737833,6.51950183076509));
#27083=CARTESIAN_POINT('Ctrl Pts',(152.742500458167,-15.5640272618256,1.97976607728038));
#27084=CARTESIAN_POINT('Ctrl Pts',(152.772870404101,-15.5659940241253,-0.000379545266269155));
#27085=CARTESIAN_POINT('Origin',(110.25,0.,0.));
#27086=CARTESIAN_POINT('',(110.,4.5,-5.51091059616309E-16));
#27087=CARTESIAN_POINT('Origin',(110.,0.,0.));
#27088=CARTESIAN_POINT('',(110.5,4.,4.89858719658941E-16));
#27089=CARTESIAN_POINT('',(110.25,4.25,-5.20474889637625E-16));
#27090=CARTESIAN_POINT('',(110.5,-4.,-4.89858719658941E-16));
#27091=CARTESIAN_POINT('Origin',(110.5,0.,0.));
#27092=CARTESIAN_POINT('Origin',(110.5,0.,0.));
#27093=CARTESIAN_POINT('Origin',(138.,0.,0.));
#27094=CARTESIAN_POINT('',(165.5,4.,-4.89858719658941E-16));
#27095=CARTESIAN_POINT('',(165.5,-4.,-4.89858719658941E-16));
#27096=CARTESIAN_POINT('Origin',(165.5,0.,0.));
#27097=CARTESIAN_POINT('Origin',(165.5,0.,0.));
#27098=CARTESIAN_POINT('',(138.,-4.,-4.89858719658941E-16));
#27099=CARTESIAN_POINT('Origin',(110.,18.,0.));
#27100=CARTESIAN_POINT('',(110.,-18.,-2.20436423846524E-15));
#27101=CARTESIAN_POINT('Origin',(110.,0.,0.));
#27102=CARTESIAN_POINT('Origin',(165.75,0.,0.));
#27103=CARTESIAN_POINT('',(166.,4.5,5.51091059616309E-16));
#27104=CARTESIAN_POINT('',(165.75,4.25,-5.20474889637625E-16));
#27105=CARTESIAN_POINT('Origin',(166.,0.,0.));
#27106=CARTESIAN_POINT('Origin',(166.,4.,0.));
#27107=CARTESIAN_POINT('',(166.,-15.7,-1.92269547466135E-15));
#27108=CARTESIAN_POINT('Origin',(166.,0.,0.));
#27109=CARTESIAN_POINT('Origin',(149.823223304703,0.,-7.76228700170039E-16));
#27110=CARTESIAN_POINT('',(150.,24.5,-3.00038465791102E-15));
#27111=CARTESIAN_POINT('Origin',(150.,0.,0.));
#27112=CARTESIAN_POINT('',(149.646446609407,25.3535533905933,3.10491480068016E-15));
#27113=CARTESIAN_POINT('',(149.823223304703,24.9267766952966,3.05264972929559E-15));
#27114=CARTESIAN_POINT('',(149.646446609407,-25.3535533905933,-3.10491480068016E-15));
#27115=CARTESIAN_POINT('Origin',(149.646446609407,0.,-1.55245740034008E-15));
#27116=CARTESIAN_POINT('Origin',(149.646446609407,0.,-1.55245740034008E-15));
#27117=CARTESIAN_POINT('Origin',(149.5,0.,0.));
#27118=CARTESIAN_POINT('',(149.,-26.,0.));
#27119=CARTESIAN_POINT('',(149.5,-25.5,-3.12284933782575E-15));
#27120=CARTESIAN_POINT('Origin',(149.,0.,0.));
#27121=CARTESIAN_POINT('Origin',(150.,16.5,0.));
#27122=CARTESIAN_POINT('',(150.,9.03673727728063,-12.6742328676692));
#27123=CARTESIAN_POINT('Ctrl Pts',(150.,7.06578282810886,14.8277078846935));
#27124=CARTESIAN_POINT('Ctrl Pts',(150.,7.3876419804473,14.6646824144564));
#27125=CARTESIAN_POINT('Ctrl Pts',(150.,7.70374682458374,14.491245032939));
#27126=CARTESIAN_POINT('Ctrl Pts',(150.,8.01354498609211,14.3075878423168));
#27127=CARTESIAN_POINT('Ctrl Pts',(150.,8.20003860763413,14.1970291016367));
#27128=CARTESIAN_POINT('Ctrl Pts',(150.,8.38424640275821,14.0827659317836));
#27129=CARTESIAN_POINT('Ctrl Pts',(150.,8.5660435295279,13.9648322169156));
#27130=CARTESIAN_POINT('Ctrl Pts',(150.,8.86854267759597,13.7685978269121));
#27131=CARTESIAN_POINT('Ctrl Pts',(150.,9.16436931521678,13.562202911389));
#27132=CARTESIAN_POINT('Ctrl Pts',(150.,9.4531259487604,13.3461003396371));
#27133=CARTESIAN_POINT('Ctrl Pts',(150.,9.68471359963282,13.1727824617919));
#27134=CARTESIAN_POINT('Ctrl Pts',(150.,9.91175309910759,12.9932193970716));
#27135=CARTESIAN_POINT('Ctrl Pts',(150.,10.1340225547111,12.8076273523271));
#27136=CARTESIAN_POINT('Ctrl Pts',(150.,10.2312654415376,12.7264308327514));
#27137=CARTESIAN_POINT('Ctrl Pts',(150.,10.3275951052629,12.6440801438521));
#27138=CARTESIAN_POINT('Ctrl Pts',(150.,10.4229919550846,12.5605925759226));
#27139=CARTESIAN_POINT('Ctrl Pts',(150.,10.4640372264647,12.5246713700449));
#27140=CARTESIAN_POINT('Ctrl Pts',(150.,10.5049098053371,12.4885396969055));
#27141=CARTESIAN_POINT('Ctrl Pts',(150.,10.5456080940746,12.4521989078195));
#27142=CARTESIAN_POINT('Ctrl Pts',(150.,10.5768828741308,12.4242726676509));
#27143=CARTESIAN_POINT('Ctrl Pts',(150.,10.6080543978282,12.3962231908927));
#27144=CARTESIAN_POINT('Ctrl Pts',(150.,10.6391119118545,12.3680603239059));
#27145=CARTESIAN_POINT('Ctrl Pts',(150.,10.9051224416353,12.1268427183698));
#27146=CARTESIAN_POINT('Ctrl Pts',(150.,11.1629640541356,11.8771392131954));
#27147=CARTESIAN_POINT('Ctrl Pts',(150.,11.4122648034249,11.6194163080923));
#27148=CARTESIAN_POINT('Ctrl Pts',(150.,11.663316550501,11.3598832510432));
#27149=CARTESIAN_POINT('Ctrl Pts',(150.,11.9057074706405,11.0922173370697));
#27150=CARTESIAN_POINT('Ctrl Pts',(150.,12.139020104929,10.8168575422661));
#27151=CARTESIAN_POINT('Ctrl Pts',(150.,12.3696205173147,10.5446987608535));
#27152=CARTESIAN_POINT('Ctrl Pts',(150.,12.5913527847256,10.2650234491502));
#27153=CARTESIAN_POINT('Ctrl Pts',(150.,12.8037719291964,9.97822590843219));
#27154=CARTESIAN_POINT('Ctrl Pts',(150.,12.9118552877259,9.83229724698291));
#27155=CARTESIAN_POINT('Ctrl Pts',(150.,13.0175267866837,9.68452421806683));
#27156=CARTESIAN_POINT('Ctrl Pts',(150.,13.1207231838825,9.53495638439154));
#27157=CARTESIAN_POINT('Ctrl Pts',(150.,13.1753746187829,9.45574725551507));
#27158=CARTESIAN_POINT('Ctrl Pts',(150.,13.2293318270461,9.37603472741769));
#27159=CARTESIAN_POINT('Ctrl Pts',(150.,13.2825850354999,9.29582600723517));
#27160=CARTESIAN_POINT('Ctrl Pts',(150.,13.3133564873096,9.24947877597002));
#27161=CARTESIAN_POINT('Ctrl Pts',(150.,13.3438963544375,9.20296040961011));
#27162=CARTESIAN_POINT('Ctrl Pts',(150.,13.3741837495123,9.15630179064984));
#27163=CARTESIAN_POINT('Ctrl Pts',(150.,13.5688092517606,8.85647550559098));
#27164=CARTESIAN_POINT('Ctrl Pts',(150.,13.7531325481106,8.55068502662042));
#27165=CARTESIAN_POINT('Ctrl Pts',(150.,13.9267868768619,8.23937315101738));
#27166=CARTESIAN_POINT('Ctrl Pts',(150.,13.9442701936976,8.20803063168576));
#27167=CARTESIAN_POINT('Ctrl Pts',(150.,13.9616453336674,8.17663211865198));
#27168=CARTESIAN_POINT('Ctrl Pts',(150.,13.978911899393,8.14517804578991));
#27169=CARTESIAN_POINT('Ctrl Pts',(150.,14.149665119914,7.83412115555321));
#27170=CARTESIAN_POINT('Ctrl Pts',(150.,14.3098038877351,7.5176329213665));
#27171=CARTESIAN_POINT('Ctrl Pts',(150.,14.4592458812746,7.19630664194355));
#27172=CARTESIAN_POINT('Ctrl Pts',(150.,14.6095351561267,6.8731585603258));
#27173=CARTESIAN_POINT('Ctrl Pts',(150.,14.7490061923864,6.5451168640693));
#27174=CARTESIAN_POINT('Ctrl Pts',(150.,14.8775272777826,6.21276242824458));
#27175=CARTESIAN_POINT('Ctrl Pts',(150.,15.0060195745878,5.88048243947166));
#27176=CARTESIAN_POINT('Ctrl Pts',(150.,15.1235669606131,5.54389106936735));
#27177=CARTESIAN_POINT('Ctrl Pts',(150.,15.2299877412795,5.20355481059925));
#27178=CARTESIAN_POINT('Ctrl Pts',(150.,15.3357635135699,4.86528130438908));
#27179=CARTESIAN_POINT('Ctrl Pts',(150.,15.4305472375715,4.52330760271481));
#27180=CARTESIAN_POINT('Ctrl Pts',(150.,15.5141094203472,4.17818464278366));
#27181=CARTESIAN_POINT('Ctrl Pts',(150.,15.5500452320262,4.02976494762718));
#27182=CARTESIAN_POINT('Ctrl Pts',(150.,15.5839050579811,3.88076280523603));
#27183=CARTESIAN_POINT('Ctrl Pts',(150.,15.6156676469,3.73122212516282));
#27184=CARTESIAN_POINT('Ctrl Pts',(150.,15.6317105670279,3.65569083920871));
#27185=CARTESIAN_POINT('Ctrl Pts',(150.,15.6472184227117,3.58002216691571));
#27186=CARTESIAN_POINT('Ctrl Pts',(150.,15.6621882966678,3.50422178644977));
#27187=CARTESIAN_POINT('Ctrl Pts',(150.,15.6710144670918,3.45953022270224));
#27188=CARTESIAN_POINT('Ctrl Pts',(150.,15.6796543727474,3.41478865442006));
#27189=CARTESIAN_POINT('Ctrl Pts',(150.,15.6881022820279,3.37002604753674));
#27190=CARTESIAN_POINT('Ctrl Pts',(150.,15.7539079983008,3.02134386944905));
#27191=CARTESIAN_POINT('Ctrl Pts',(150.,15.8081300769565,2.67108305809694));
#27192=CARTESIAN_POINT('Ctrl Pts',(150.,15.850673220764,2.31981577884298));
#27193=CARTESIAN_POINT('Ctrl Pts',(150.,15.8931832860664,1.96882161989506));
#27194=CARTESIAN_POINT('Ctrl Pts',(150.,15.9240326794299,1.61682198581937));
#27195=CARTESIAN_POINT('Ctrl Pts',(150.,15.9430758712819,1.26437592001532));
#27196=CARTESIAN_POINT('Ctrl Pts',(150.,15.955887932133,1.02725388307379));
#27197=CARTESIAN_POINT('Ctrl Pts',(150.,15.9633549233283,0.789929536529496));
#27198=CARTESIAN_POINT('Ctrl Pts',(150.,15.9654192721832,0.552572077685281));
#27199=CARTESIAN_POINT('Ctrl Pts',(150.,15.9684942852131,0.199009123944068));
#27200=CARTESIAN_POINT('Ctrl Pts',(150.,15.959583998504,-0.154627786657829));
#27201=CARTESIAN_POINT('Ctrl Pts',(150.,15.9388380541415,-0.507759999674467));
#27202=CARTESIAN_POINT('Ctrl Pts',(150.,15.9181162996423,-0.860480458961035));
#27203=CARTESIAN_POINT('Ctrl Pts',(150.,15.8855863159675,-1.21269796963108));
#27204=CARTESIAN_POINT('Ctrl Pts',(150.,15.8413465220212,-1.56382488170133));
#27205=CARTESIAN_POINT('Ctrl Pts',(150.,15.8116151333713,-1.7998000017681));
#27206=CARTESIAN_POINT('Ctrl Pts',(150.,15.7765939397513,-2.03528231493771));
#27207=CARTESIAN_POINT('Ctrl Pts',(150.,15.7363004455236,-2.27008868110735));
#27208=CARTESIAN_POINT('Ctrl Pts',(150.,15.718672041799,-2.37281646630657));
#27209=CARTESIAN_POINT('Ctrl Pts',(150.,15.700034360781,-2.47541481223874));
#27210=CARTESIAN_POINT('Ctrl Pts',(150.,15.6803882863496,-2.577868081932));
#27211=CARTESIAN_POINT('Ctrl Pts',(150.,15.6725708481322,-2.6186356209535));
#27212=CARTESIAN_POINT('Ctrl Pts',(150.,15.6645937418988,-2.65938018708575));
#27213=CARTESIAN_POINT('Ctrl Pts',(150.,15.6564570079706,-2.70010078606003));
#27214=CARTESIAN_POINT('Ctrl Pts',(150.,15.6496235725067,-2.7342989775701));
#27215=CARTESIAN_POINT('Ctrl Pts',(150.,15.6426774366298,-2.76848066450812));
#27216=CARTESIAN_POINT('Ctrl Pts',(150.,15.6356218052556,-2.80263028884055));
#27217=CARTESIAN_POINT('Ctrl Pts',(150.,15.5646458610471,-3.14615756553515));
#27218=CARTESIAN_POINT('Ctrl Pts',(150.,15.4825212883806,-3.4868094060629));
#27219=CARTESIAN_POINT('Ctrl Pts',(150.,15.3894544689962,-3.82403800229257));
#27220=CARTESIAN_POINT('Ctrl Pts',(150.,15.2958691082522,-4.16314553857796));
#27221=CARTESIAN_POINT('Ctrl Pts',(150.,15.1912191037315,-4.49879215189183));
#27222=CARTESIAN_POINT('Ctrl Pts',(150.,15.075662546082,-4.83041256132867));
#27223=CARTESIAN_POINT('Ctrl Pts',(150.,14.9604081100008,-5.1611659522229));
#27224=CARTESIAN_POINT('Ctrl Pts',(150.,14.8343038948605,-5.48791471934051));
#27225=CARTESIAN_POINT('Ctrl Pts',(150.,14.6974578001503,-5.81008135591099));
#27226=CARTESIAN_POINT('Ctrl Pts',(150.,14.5620425815663,-6.12887938667728));
#27227=CARTESIAN_POINT('Ctrl Pts',(150.,14.4161087215575,-6.44319110561363));
#27228=CARTESIAN_POINT('Ctrl Pts',(150.,14.2597158771019,-6.75243283543992));
#27229=CARTESIAN_POINT('Ctrl Pts',(150.,14.2213695562824,-6.82825652560918));
#27230=CARTESIAN_POINT('Ctrl Pts',(150.,14.1823942444334,-6.90377527744399));
#27231=CARTESIAN_POINT('Ctrl Pts',(150.,14.142790426037,-6.97898021017884));
#27232=CARTESIAN_POINT('Ctrl Pts',(150.,13.9929250135453,-7.26356434176228));
#27233=CARTESIAN_POINT('Ctrl Pts',(150.,13.8340617188498,-7.54365669711128));
#27234=CARTESIAN_POINT('Ctrl Pts',(150.,13.6664743986313,-7.81889776725218));
#27235=CARTESIAN_POINT('Ctrl Pts',(150.,13.5931549460357,-7.93931573543883));
#27236=CARTESIAN_POINT('Ctrl Pts',(150.,13.5181653204488,-8.05880480754739));
#27237=CARTESIAN_POINT('Ctrl Pts',(150.,13.4415269527696,-8.1773332441067));
#27238=CARTESIAN_POINT('Ctrl Pts',(150.,13.4114222136612,-8.22389305178011));
#27239=CARTESIAN_POINT('Ctrl Pts',(150.,13.3810630576661,-8.27030461804413));
#27240=CARTESIAN_POINT('Ctrl Pts',(150.,13.3504507482978,-8.31656597356602));
#27241=CARTESIAN_POINT('Ctrl Pts',(150.,13.3224450834883,-8.3588881649692));
#27242=CARTESIAN_POINT('Ctrl Pts',(150.,13.2942238181009,-8.40109005482901));
#27243=CARTESIAN_POINT('Ctrl Pts',(150.,13.2658080686662,-8.44314055564525));
#27244=CARTESIAN_POINT('Ctrl Pts',(150.,13.071711669246,-8.73037038292888));
#27245=CARTESIAN_POINT('Ctrl Pts',(150.,12.8684114271802,-9.01074622663321));
#27246=CARTESIAN_POINT('Ctrl Pts',(150.,12.656361724003,-9.28390086392591));
#27247=CARTESIAN_POINT('Ctrl Pts',(150.,12.4426766270286,-9.55916215542676));
#27248=CARTESIAN_POINT('Ctrl Pts',(150.,12.2201062317378,-9.82709087463049));
#27249=CARTESIAN_POINT('Ctrl Pts',(150.,11.9890703934198,-10.0872836008548));
#27250=CARTESIAN_POINT('Ctrl Pts',(150.,11.7579191485341,-10.3476062980382));
#27251=CARTESIAN_POINT('Ctrl Pts',(150.,11.5182935940267,-10.6001856936534));
#27252=CARTESIAN_POINT('Ctrl Pts',(150.,11.2705750738404,-10.8445837082846));
#27253=CARTESIAN_POINT('Ctrl Pts',(150.,11.0242453255649,-11.0876115665887));
#27254=CARTESIAN_POINT('Ctrl Pts',(150.,10.7699126752476,-11.3225498984125));
#27255=CARTESIAN_POINT('Ctrl Pts',(150.,10.5079196621001,-11.5489283694475));
#27256=CARTESIAN_POINT('Ctrl Pts',(150.,10.2501511146187,-11.7716566359715));
#27257=CARTESIAN_POINT('Ctrl Pts',(150.,9.98496681714273,-11.9860991380323));
#27258=CARTESIAN_POINT('Ctrl Pts',(150.,9.71266793165041,-12.1917647788381));
#27259=CARTESIAN_POINT('Ctrl Pts',(150.,9.4919811642635,-12.3584481104644));
#27260=CARTESIAN_POINT('Ctrl Pts',(150.,9.26662069281188,-12.5193657157872));
#27261=CARTESIAN_POINT('Ctrl Pts',(150.,9.03673727728059,-12.6742328676692));
#27262=CARTESIAN_POINT('',(150.,-9.03673727728022,-12.6742328676695));
#27263=CARTESIAN_POINT('Origin',(150.,0.,0.));
#27264=CARTESIAN_POINT('Ctrl Pts',(150.,-9.03713009573235,-12.6741506013612));
#27265=CARTESIAN_POINT('Ctrl Pts',(150.,-9.32675130828298,-12.4794591630376));
#27266=CARTESIAN_POINT('Ctrl Pts',(150.,-9.60948430272415,-12.2752594880836));
#27267=CARTESIAN_POINT('Ctrl Pts',(150.,-9.88481429489231,-12.0618497574774));
#27268=CARTESIAN_POINT('Ctrl Pts',(150.,-10.0428450895277,-11.9393592541907));
#27269=CARTESIAN_POINT('Ctrl Pts',(150.,-10.1984366956213,-11.8138336902965));
#27270=CARTESIAN_POINT('Ctrl Pts',(150.,-10.3514882980122,-11.685322512026));
#27271=CARTESIAN_POINT('Ctrl Pts',(150.,-10.6171411156183,-11.4622646931721));
#27272=CARTESIAN_POINT('Ctrl Pts',(150.,-10.8751436575605,-11.2302144699766));
#27273=CARTESIAN_POINT('Ctrl Pts',(150.,-11.1251971708097,-10.989681345775));
#27274=CARTESIAN_POINT('Ctrl Pts',(150.,-11.3264658616713,-10.7960756395891));
#27275=CARTESIAN_POINT('Ctrl Pts',(150.,-11.5225841327858,-10.596973184495));
#27276=CARTESIAN_POINT('Ctrl Pts',(150.,-11.7133796840543,-10.3926215396668));
#27277=CARTESIAN_POINT('Ctrl Pts',(150.,-11.7968527377343,-10.3032176950545));
#27278=CARTESIAN_POINT('Ctrl Pts',(150.,-11.8793067872374,-10.212808930071));
#27279=CARTESIAN_POINT('Ctrl Pts',(150.,-11.9607264194818,-10.1214151270844));
#27280=CARTESIAN_POINT('Ctrl Pts',(150.,-11.9958094399868,-10.08203432204));
#27281=CARTESIAN_POINT('Ctrl Pts',(150.,-12.0307003950494,-10.0424706214301));
#27282=CARTESIAN_POINT('Ctrl Pts',(150.,-12.0653980152307,-10.0027255888958));
#27283=CARTESIAN_POINT('Ctrl Pts',(150.,-12.0915722427461,-9.97274383456447));
#27284=CARTESIAN_POINT('Ctrl Pts',(150.,-12.1176335868785,-9.94266214609465));
#27285=CARTESIAN_POINT('Ctrl Pts',(150.,-12.1435764176906,-9.91248733704835));
#27286=CARTESIAN_POINT('Ctrl Pts',(150.,-12.370855862704,-9.64813245985379));
#27287=CARTESIAN_POINT('Ctrl Pts',(150.,-12.5891632401871,-9.37649512848077));
#27288=CARTESIAN_POINT('Ctrl Pts',(150.,-12.798217773339,-9.09810414031864));
#27289=CARTESIAN_POINT('Ctrl Pts',(150.,-13.0086584353209,-8.81786729036698));
#27290=CARTESIAN_POINT('Ctrl Pts',(150.,-13.2097235351087,-8.53078649584846));
#27291=CARTESIAN_POINT('Ctrl Pts',(150.,-13.4010903795913,-8.23736297463736));
#27292=CARTESIAN_POINT('Ctrl Pts',(150.,-13.5919691678086,-7.94468779198147));
#27293=CARTESIAN_POINT('Ctrl Pts',(150.,-13.7731994468326,-7.64570171222069));
#27294=CARTESIAN_POINT('Ctrl Pts',(150.,-13.9444195937118,-7.3408712172528));
#27295=CARTESIAN_POINT('Ctrl Pts',(150.,-14.0293152641616,-7.18972785173465));
#27296=CARTESIAN_POINT('Ctrl Pts',(150.,-14.1117493216321,-7.03714723294329));
#27297=CARTESIAN_POINT('Ctrl Pts',(150.,-14.1916734971045,-6.88318395033817));
#27298=CARTESIAN_POINT('Ctrl Pts',(150.,-14.231107214406,-6.80722014432851));
#27299=CARTESIAN_POINT('Ctrl Pts',(150.,-14.2699298996688,-6.73091973174407));
#27300=CARTESIAN_POINT('Ctrl Pts',(150.,-14.3081354892757,-6.65428915565419));
#27301=CARTESIAN_POINT('Ctrl Pts',(150.,-14.3309894228917,-6.60845004894412));
#27302=CARTESIAN_POINT('Ctrl Pts',(150.,-14.3536246467107,-6.56248835872825));
#27303=CARTESIAN_POINT('Ctrl Pts',(150.,-14.3760267541699,-6.51643268441378));
#27304=CARTESIAN_POINT('Ctrl Pts',(150.,-14.5303274258899,-6.19921157045388));
#27305=CARTESIAN_POINT('Ctrl Pts',(150.,-14.6736828241265,-5.8773171309456));
#27306=CARTESIAN_POINT('Ctrl Pts',(150.,-14.8058059081092,-5.55126966129319));
#27307=CARTESIAN_POINT('Ctrl Pts',(150.,-14.8174163159938,-5.5226180131611));
#27308=CARTESIAN_POINT('Ctrl Pts',(150.,-14.8289399613271,-5.49393427291357));
#27309=CARTESIAN_POINT('Ctrl Pts',(150.,-14.8403766345866,-5.46521878133834));
#27310=CARTESIAN_POINT('Ctrl Pts',(150.,-14.969217594009,-5.14172160686549));
#27311=CARTESIAN_POINT('Ctrl Pts',(150.,-15.087024399383,-4.81419707145875));
#27312=CARTESIAN_POINT('Ctrl Pts',(150.,-15.1938238425128,-4.48324472088699));
#27313=CARTESIAN_POINT('Ctrl Pts',(150.,-15.3015591096403,-4.14939241931651));
#27314=CARTESIAN_POINT('Ctrl Pts',(150.,-15.3980934196097,-3.81205143901055));
#27315=CARTESIAN_POINT('Ctrl Pts',(150.,-15.4834062862694,-3.47181341026954));
#27316=CARTESIAN_POINT('Ctrl Pts',(150.,-15.5690125587188,-3.13040524375862));
#27317=CARTESIAN_POINT('Ctrl Pts',(150.,-15.6433201934172,-2.78607950118257));
#27318=CARTESIAN_POINT('Ctrl Pts',(150.,-15.706258362334,-2.43941835600141));
#27319=CARTESIAN_POINT('Ctrl Pts',(150.,-15.7690404765126,-2.09361675464159));
#27320=CARTESIAN_POINT('Ctrl Pts',(150.,-15.8205095189187,-1.74549073870081));
#27321=CARTESIAN_POINT('Ctrl Pts',(150.,-15.860543920808,-1.39561128848453));
#27322=CARTESIAN_POINT('Ctrl Pts',(150.,-15.8778029773184,-1.24477628363531));
#27323=CARTESIAN_POINT('Ctrl Pts',(150.,-15.8929362272837,-1.09361536384623));
#27324=CARTESIAN_POINT('Ctrl Pts',(150.,-15.9059309180032,-0.942174294848833));
#27325=CARTESIAN_POINT('Ctrl Pts',(150.,-15.9127116225689,-0.863151471594134));
#27326=CARTESIAN_POINT('Ctrl Pts',(150.,-15.9189100072436,-0.784052370778021));
#27327=CARTESIAN_POINT('Ctrl Pts',(150.,-15.9245240604719,-0.704883513438272));
#27328=CARTESIAN_POINT('Ctrl Pts',(150.,-15.9273357657567,-0.665233106590456));
#27329=CARTESIAN_POINT('Ctrl Pts',(150.,-15.930000944285,-0.625563840008872));
#27330=CARTESIAN_POINT('Ctrl Pts',(150.,-15.9325181502449,-0.58589706136608));
#27331=CARTESIAN_POINT('Ctrl Pts',(150.,-15.9549841971573,-0.231871318522656));
#27332=CARTESIAN_POINT('Ctrl Pts',(150.,-15.9656952733194,0.122328988982216));
#27333=CARTESIAN_POINT('Ctrl Pts',(150.,-15.964663028844,0.476104466719937));
#27334=CARTESIAN_POINT('Ctrl Pts',(150.,-15.963626438801,0.831369276938752));
#27335=CARTESIAN_POINT('Ctrl Pts',(150.,-15.9507475567728,1.18620625026855));
#27336=CARTESIAN_POINT('Ctrl Pts',(150.,-15.9259875244419,1.54002188838368));
#27337=CARTESIAN_POINT('Ctrl Pts',(150.,-15.9096853081207,1.77297712015682));
#27338=CARTESIAN_POINT('Ctrl Pts',(150.,-15.8882315518575,2.0054898613174));
#27339=CARTESIAN_POINT('Ctrl Pts',(150.,-15.8616028955927,2.23739204259502));
#27340=CARTESIAN_POINT('Ctrl Pts',(150.,-15.8212798853536,2.58855486272253));
#27341=CARTESIAN_POINT('Ctrl Pts',(150.,-15.7690932560903,2.93831808304219));
#27342=CARTESIAN_POINT('Ctrl Pts',(150.,-15.7052969768754,3.28614647273987));
#27343=CARTESIAN_POINT('Ctrl Pts',(150.,-15.6413364804764,3.63487020303523));
#27344=CARTESIAN_POINT('Ctrl Pts',(150.,-15.5657063273605,3.98164968446553));
#27345=CARTESIAN_POINT('Ctrl Pts',(150.,-15.4786108162115,4.32593597572798));
#27346=CARTESIAN_POINT('Ctrl Pts',(150.,-15.4190869863304,4.56123212774712));
#27347=CARTESIAN_POINT('Ctrl Pts',(150.,-15.3542068592886,4.79536356426335));
#27348=CARTESIAN_POINT('Ctrl Pts',(150.,-15.2840224182957,5.02815045121079));
#27349=CARTESIAN_POINT('Ctrl Pts',(150.,-15.2533167253613,5.1299947142503));
#27350=CARTESIAN_POINT('Ctrl Pts',(150.,-15.2215956180984,5.23158156413266));
#27351=CARTESIAN_POINT('Ctrl Pts',(150.,-15.188862825923,5.33289564289095));
#27352=CARTESIAN_POINT('Ctrl Pts',(150.,-15.1755305235451,5.37416159801956));
#27353=CARTESIAN_POINT('Ctrl Pts',(150.,-15.1620303791686,5.41538229834444));
#27354=CARTESIAN_POINT('Ctrl Pts',(150.,-15.1483626271037,5.45655669628066));
#27355=CARTESIAN_POINT('Ctrl Pts',(150.,-15.1375744047441,5.48905644886255));
#27356=CARTESIAN_POINT('Ctrl Pts',(150.,-15.1266818175398,5.52152708261994));
#27357=CARTESIAN_POINT('Ctrl Pts',(150.,-15.1156895277528,5.55395494244973));
#27358=CARTESIAN_POINT('Ctrl Pts',(150.,-15.0017362463883,5.89012339386607));
#27359=CARTESIAN_POINT('Ctrl Pts',(150.,-14.8769534065169,6.22205632476711));
#27360=CARTESIAN_POINT('Ctrl Pts',(150.,-14.7416520189261,6.54923687148926));
#27361=CARTESIAN_POINT('Ctrl Pts',(150.,-14.6048919693399,6.87994469784704));
#27362=CARTESIAN_POINT('Ctrl Pts',(150.,-14.4573852372237,7.20579767618766));
#27363=CARTESIAN_POINT('Ctrl Pts',(150.,-14.2994004327061,7.52625523447028));
#27364=CARTESIAN_POINT('Ctrl Pts',(150.,-14.1413143169204,7.84691829328636));
#27365=CARTESIAN_POINT('Ctrl Pts',(150.,-13.9727364884057,8.162179567917));
#27366=CARTESIAN_POINT('Ctrl Pts',(150.,-13.7938862061515,8.47148227089501));
#27367=CARTESIAN_POINT('Ctrl Pts',(150.,-13.6162151688029,8.77874559416266));
#27368=CARTESIAN_POINT('Ctrl Pts',(150.,-13.4284064523002,9.08012918547539));
#27369=CARTESIAN_POINT('Ctrl Pts',(150.,-13.2306291725494,9.37506419100143));
#27370=CARTESIAN_POINT('Ctrl Pts',(150.,-13.1804286520628,9.44992562506406));
#27371=CARTESIAN_POINT('Ctrl Pts',(150.,-13.129585671806,9.52437146170184));
#27372=CARTESIAN_POINT('Ctrl Pts',(150.,-13.0781025512757,9.59839209806963));
#27373=CARTESIAN_POINT('Ctrl Pts',(150.,-12.8868363481183,9.8733879788073));
#27374=CARTESIAN_POINT('Ctrl Pts',(150.,-12.6867371439721,10.1425172733571));
#27375=CARTESIAN_POINT('Ctrl Pts',(150.,-12.4781574315827,10.4054645622175));
#27376=CARTESIAN_POINT('Ctrl Pts',(150.,-12.3869038074123,10.520504001094));
#27377=CARTESIAN_POINT('Ctrl Pts',(150.,-12.2940265755823,10.6343598142344));
#27378=CARTESIAN_POINT('Ctrl Pts',(150.,-12.1995535549077,10.747003852065));
#27379=CARTESIAN_POINT('Ctrl Pts',(150.,-12.1572188161594,10.7974812886818));
#27380=CARTESIAN_POINT('Ctrl Pts',(150.,-12.1145636193238,10.8477153777883));
#27381=CARTESIAN_POINT('Ctrl Pts',(150.,-12.07159040601,10.8977035118573));
#27382=CARTESIAN_POINT('Ctrl Pts',(150.,-12.047631773304,10.9255731369437));
#27383=CARTESIAN_POINT('Ctrl Pts',(150.,-12.0235735549359,10.9533671050331));
#27384=CARTESIAN_POINT('Ctrl Pts',(150.,-11.9994275296361,10.9810720667265));
#27385=CARTESIAN_POINT('Ctrl Pts',(150.,-11.7657438596099,11.2491988928222));
#27386=CARTESIAN_POINT('Ctrl Pts',(150.,-11.5235990501437,11.5092729716365));
#27387=CARTESIAN_POINT('Ctrl Pts',(150.,-11.2735221781638,11.7610044607555));
#27388=CARTESIAN_POINT('Ctrl Pts',(150.,-11.0208038684604,12.0153948644967));
#27389=CARTESIAN_POINT('Ctrl Pts',(150.,-10.7599847006905,12.2612659227395));
#27390=CARTESIAN_POINT('Ctrl Pts',(150.,-10.4915645756216,12.4982917824595));
#27391=CARTESIAN_POINT('Ctrl Pts',(150.,-10.2214665929276,12.7367992585298));
#27392=CARTESIAN_POINT('Ctrl Pts',(150.,-9.94367193934656,12.9663510283537));
#27393=CARTESIAN_POINT('Ctrl Pts',(150.,-9.65864912466268,13.1865819124749));
#27394=CARTESIAN_POINT('Ctrl Pts',(150.,-9.37433281843848,13.4062668929887));
#27395=CARTESIAN_POINT('Ctrl Pts',(150.,-9.08282369807402,13.6166775145209));
#27396=CARTESIAN_POINT('Ctrl Pts',(150.,-8.78455265000496,13.8174125168282));
#27397=CARTESIAN_POINT('Ctrl Pts',(150.,-8.49002264483304,14.0156298149888));
#27398=CARTESIAN_POINT('Ctrl Pts',(150.,-8.1888988077542,14.2044129755868));
#27399=CARTESIAN_POINT('Ctrl Pts',(150.,-7.88156947113482,14.3833329330089));
#27400=CARTESIAN_POINT('Ctrl Pts',(150.,-7.61411854288894,14.5390366130436));
#27401=CARTESIAN_POINT('Ctrl Pts',(150.,-7.34196749469852,14.6872701843133));
#27402=CARTESIAN_POINT('Ctrl Pts',(150.,-7.06535955977555,14.8277213114857));
#27403=CARTESIAN_POINT('Origin',(124.,-2.95337249083895E-16,37.1267766952966));
#27404=CARTESIAN_POINT('',(114.353553390593,-9.86076131526265E-31,37.5535533905933));
#27405=CARTESIAN_POINT('Origin',(124.,-5.9067449816779E-16,37.5535533905933));
#27406=CARTESIAN_POINT('',(114.215409426056,6.00395323027717E-16,37.2200443578465));
#27407=CARTESIAN_POINT('',(114.176776695297,-1.79367239590926E-15,37.1267766952966));
#27408=CARTESIAN_POINT('',(114.458327956987,-2.99274032010616,36.6999999999997));
#27409=CARTESIAN_POINT('Ctrl Pts',(114.458327956987,-2.99274032010619,36.6999999999997));
#27410=CARTESIAN_POINT('Ctrl Pts',(114.404771619819,-2.64468250602247,36.8281053294846));
#27411=CARTESIAN_POINT('Ctrl Pts',(114.355518882547,-2.27707927894242,36.9352309965706));
#27412=CARTESIAN_POINT('Ctrl Pts',(114.24985583958,-1.26419506839176,37.1564542606582));
#27413=CARTESIAN_POINT('Ctrl Pts',(114.215409426056,-0.605353187125128,
37.2200443578465));
#27414=CARTESIAN_POINT('Ctrl Pts',(114.215409426056,2.63677968348475E-15,
37.2200443578465));
#27415=CARTESIAN_POINT('',(114.458327956987,2.99274032010617,36.6999999999997));
#27416=CARTESIAN_POINT('Origin',(124.,0.,36.7));
#27417=CARTESIAN_POINT('Ctrl Pts',(114.215409426056,3.05311331771918E-15,
37.2200443578465));
#27418=CARTESIAN_POINT('Ctrl Pts',(114.215409426056,0.605353187125133,37.2200443578465));
#27419=CARTESIAN_POINT('Ctrl Pts',(114.24985583958,1.26419506839177,37.1564542606582));
#27420=CARTESIAN_POINT('Ctrl Pts',(114.355518882547,2.27707927894242,36.9352309965706));
#27421=CARTESIAN_POINT('Ctrl Pts',(114.404771619819,2.64468250602248,36.8281053294846));
#27422=CARTESIAN_POINT('Ctrl Pts',(114.458327956987,2.99274032010619,36.6999999999997));
#27423=CARTESIAN_POINT('Origin',(124.,0.,37.6));
#27424=CARTESIAN_POINT('',(114.446446609407,-2.33994571605468E-15,37.6464466094067));
#27425=CARTESIAN_POINT('Origin',(124.,-5.8498642901367E-16,37.6464466094067));
#27426=CARTESIAN_POINT('',(114.4,-1.17566092718146E-15,37.6));
#27427=CARTESIAN_POINT('Origin',(124.,-2.92493214506835E-16,37.8232233047034));
#27428=CARTESIAN_POINT('',(115.3,1.0654427152582E-15,38.));
#27429=CARTESIAN_POINT('',(114.873223304703,5.32721357629098E-16,37.8232233047034));
#27430=CARTESIAN_POINT('Origin',(124.,0.,38.));
#27431=CARTESIAN_POINT('Origin',(124.,0.,38.));
#27432=CARTESIAN_POINT('',(119.59,-5.40069238423981E-16,38.));
#27433=CARTESIAN_POINT('Origin',(124.,0.,38.));
#27434=CARTESIAN_POINT('Origin',(165.275,2.00740175623163E-15,0.));
#27435=CARTESIAN_POINT('Ctrl Pts',(165.275,15.2541446685788,3.10078767190756));
#27436=CARTESIAN_POINT('Ctrl Pts',(165.275,15.1940847495464,3.44455795624862));
#27437=CARTESIAN_POINT('Ctrl Pts',(165.275,15.1225369332471,3.78590288866285));
#27438=CARTESIAN_POINT('Ctrl Pts',(165.275,15.039564239907,4.12423090934285));
#27439=CARTESIAN_POINT('Ctrl Pts',(165.275,14.9919405116494,4.31842060079662));
#27440=CARTESIAN_POINT('Ctrl Pts',(165.275,14.9405520100828,4.51161645307205));
#27441=CARTESIAN_POINT('Ctrl Pts',(165.275,14.8854029013542,4.7037062553512));
#27442=CARTESIAN_POINT('Ctrl Pts',(165.275,14.7896801790758,5.03711796806907));
#27443=CARTESIAN_POINT('Ctrl Pts',(165.275,14.6826308389638,5.3671983468427));
#27444=CARTESIAN_POINT('Ctrl Pts',(165.275,14.5645988217881,5.69346723342415));
#27445=CARTESIAN_POINT('Ctrl Pts',(165.275,14.4695945590912,5.95608186759131));
#27446=CARTESIAN_POINT('Ctrl Pts',(165.275,14.3674739018206,6.21622708849436));
#27447=CARTESIAN_POINT('Ctrl Pts',(165.275,14.2583929258337,6.47364480071921));
#27448=CARTESIAN_POINT('Ctrl Pts',(165.275,14.2106699988393,6.58626504981758));
#27449=CARTESIAN_POINT('Ctrl Pts',(165.275,14.1616145650519,6.69836313022639));
#27450=CARTESIAN_POINT('Ctrl Pts',(165.275,14.1112385188583,6.80991687450263));
#27451=CARTESIAN_POINT('Ctrl Pts',(165.275,14.0895319144857,6.85798442200299));
#27452=CARTESIAN_POINT('Ctrl Pts',(165.275,14.0675801066771,6.90595089933359));
#27453=CARTESIAN_POINT('Ctrl Pts',(165.275,14.045384007563,6.95381451081383));
#27454=CARTESIAN_POINT('Ctrl Pts',(165.275,14.0286403330267,6.98992052785015));
#27455=CARTESIAN_POINT('Ctrl Pts',(165.275,14.0117594503612,7.02596406769214));
#27456=CARTESIAN_POINT('Ctrl Pts',(165.275,13.9947452941642,7.06193721580921));
#27457=CARTESIAN_POINT('Ctrl Pts',(165.275,13.8456879753542,7.37709013584798));
#27458=CARTESIAN_POINT('Ctrl Pts',(165.275,13.6863285350277,7.68700870539031));
#27459=CARTESIAN_POINT('Ctrl Pts',(165.275,13.517035851541,7.99122134069323));
#27460=CARTESIAN_POINT('Ctrl Pts',(165.275,13.3466206778106,8.29745104907986));
#27461=CARTESIAN_POINT('Ctrl Pts',(165.275,13.1661398649656,8.59789943816228));
#27462=CARTESIAN_POINT('Ctrl Pts',(165.275,12.9759200473297,8.89206784933303));
#27463=CARTESIAN_POINT('Ctrl Pts',(165.275,12.7861853604144,9.18548602251582));
#27464=CARTESIAN_POINT('Ctrl Pts',(165.275,12.5867609800285,9.47265671684954));
#27465=CARTESIAN_POINT('Ctrl Pts',(165.275,12.3779259734097,9.75305983794163));
#27466=CARTESIAN_POINT('Ctrl Pts',(165.275,12.2743798164744,9.89209144021882));
#27467=CARTESIAN_POINT('Ctrl Pts',(165.275,12.1685194351303,10.0294588305789));
#27468=CARTESIAN_POINT('Ctrl Pts',(165.275,12.0603750665682,10.1650957095289));
#27469=CARTESIAN_POINT('Ctrl Pts',(165.275,12.0070178110528,10.2320174707235));
#27470=CARTESIAN_POINT('Ctrl Pts',(165.275,11.9531045209606,10.298517936528));
#27471=CARTESIAN_POINT('Ctrl Pts',(165.275,11.8986386160355,10.3645889469169));
#27472=CARTESIAN_POINT('Ctrl Pts',(165.275,11.8660580378524,10.4041115018543));
#27473=CARTESIAN_POINT('Ctrl Pts',(165.275,11.8332765167504,10.4434841146213));
#27474=CARTESIAN_POINT('Ctrl Pts',(165.275,11.8003143199149,10.4826819917362));
#27475=CARTESIAN_POINT('Ctrl Pts',(165.275,11.573278149431,10.7526681202608));
#27476=CARTESIAN_POINT('Ctrl Pts',(165.275,11.3375208402646,11.0145560562498));
#27477=CARTESIAN_POINT('Ctrl Pts',(165.275,11.0934009560395,11.2678719516012));
#27478=CARTESIAN_POINT('Ctrl Pts',(165.275,11.0719487514733,11.2901322620393));
#27479=CARTESIAN_POINT('Ctrl Pts',(165.275,11.0504319397965,11.3123263639781));
#27480=CARTESIAN_POINT('Ctrl Pts',(165.275,11.0288507471137,11.3344539273987));
#27481=CARTESIAN_POINT('Ctrl Pts',(165.275,10.7857257125245,11.5837341549126));
#27482=CARTESIAN_POINT('Ctrl Pts',(165.275,10.5344335063808,11.8245722558248));
#27483=CARTESIAN_POINT('Ctrl Pts',(165.275,10.2755327379732,12.0567488486662));
#27484=CARTESIAN_POINT('Ctrl Pts',(165.275,10.0143633671011,12.2909598749857));
#27485=CARTESIAN_POINT('Ctrl Pts',(165.275,9.74545109022612,12.5163572909644));
#27486=CARTESIAN_POINT('Ctrl Pts',(165.275,9.46932805581463,12.7326817440873));
#27487=CARTESIAN_POINT('Ctrl Pts',(165.275,9.19225538581756,12.9497501749778));
#27488=CARTESIAN_POINT('Ctrl Pts',(165.275,8.90792180753051,13.1576834716916));
#27489=CARTESIAN_POINT('Ctrl Pts',(165.275,8.61683035427967,13.3561801385625));
#27490=CARTESIAN_POINT('Ctrl Pts',(165.275,8.32646065840726,13.5541846355936));
#27491=CARTESIAN_POINT('Ctrl Pts',(165.275,8.02936606305868,13.7427995519239));
#27492=CARTESIAN_POINT('Ctrl Pts',(165.275,7.72601873800543,13.9216815905986));
#27493=CARTESIAN_POINT('Ctrl Pts',(165.275,7.59524399649598,13.9987986456584));
#27494=CARTESIAN_POINT('Ctrl Pts',(165.275,7.46330687339461,14.0741062414512));
#27495=CARTESIAN_POINT('Ctrl Pts',(165.275,7.33024399076646,14.1475741132254));
#27496=CARTESIAN_POINT('Ctrl Pts',(165.275,7.26081100839877,14.1859100739737));
#27497=CARTESIAN_POINT('Ctrl Pts',(165.275,7.19107149212728,14.2237450839022));
#27498=CARTESIAN_POINT('Ctrl Pts',(165.275,7.1210305810407,14.2610746530209));
#27499=CARTESIAN_POINT('Ctrl Pts',(165.275,7.08595176066735,14.279770544171));
#27500=CARTESIAN_POINT('Ctrl Pts',(165.275,7.05079611328678,14.2983402474553));
#27501=CARTESIAN_POINT('Ctrl Pts',(165.275,7.01558255289532,14.3167737591828));
#27502=CARTESIAN_POINT('Ctrl Pts',(165.275,6.70130170909565,14.481292755714));
#27503=CARTESIAN_POINT('Ctrl Pts',(165.275,6.38208021460805,14.6351440545872));
#27504=CARTESIAN_POINT('Ctrl Pts',(165.275,6.05847038177945,14.7780945032695));
#27505=CARTESIAN_POINT('Ctrl Pts',(165.275,5.73349820723714,14.9216467487436));
#27506=CARTESIAN_POINT('Ctrl Pts',(165.275,5.40410018618065,15.0542065060152));
#27507=CARTESIAN_POINT('Ctrl Pts',(165.275,5.07080270097262,15.1754968789651));
#27508=CARTESIAN_POINT('Ctrl Pts',(165.275,4.85135680028192,15.2553554927211));
#27509=CARTESIAN_POINT('Ctrl Pts',(165.275,4.63021981440457,15.330327964054));
#27510=CARTESIAN_POINT('Ctrl Pts',(165.275,4.40753578078987,15.4003245926304));
#27511=CARTESIAN_POINT('Ctrl Pts',(165.275,4.07033172827201,15.5063184819786));
#27512=CARTESIAN_POINT('Ctrl Pts',(165.275,3.72958090391352,15.6009051485531));
#27513=CARTESIAN_POINT('Ctrl Pts',(165.275,3.38587556434815,15.6840989062321));
#27514=CARTESIAN_POINT('Ctrl Pts',(165.275,3.04128550267235,15.7675068105896));
#27515=CARTESIAN_POINT('Ctrl Pts',(165.275,2.69372512292066,15.8394631567612));
#27516=CARTESIAN_POINT('Ctrl Pts',(165.275,2.34377900408581,15.8999313059081));
#27517=CARTESIAN_POINT('Ctrl Pts',(165.275,2.10461474598403,15.9412571536633));
#27518=CARTESIAN_POINT('Ctrl Pts',(165.275,1.86433590591982,15.9772160482172));
#27519=CARTESIAN_POINT('Ctrl Pts',(165.275,1.62312791409366,16.0077823333527));
#27520=CARTESIAN_POINT('Ctrl Pts',(165.275,1.51759941766972,16.0211550830995));
#27521=CARTESIAN_POINT('Ctrl Pts',(165.275,1.41189307363926,16.0334955063498));
#27522=CARTESIAN_POINT('Ctrl Pts',(165.275,1.30602442910336,16.0448007634354));
#27523=CARTESIAN_POINT('Ctrl Pts',(165.275,1.26290336082618,16.0494054768027));
#27524=CARTESIAN_POINT('Ctrl Pts',(165.275,1.2197553673707,16.0538384520432));
#27525=CARTESIAN_POINT('Ctrl Pts',(165.275,1.17658150105774,16.0580994771177));
#27526=CARTESIAN_POINT('Ctrl Pts',(165.275,1.1425035349691,16.0614627864618));
#27527=CARTESIAN_POINT('Ctrl Pts',(165.275,1.10840972125022,16.0647189100905));
#27528=CARTESIAN_POINT('Ctrl Pts',(165.275,1.07431443076556,16.0678665531613));
#27529=CARTESIAN_POINT('Ctrl Pts',(165.275,0.720860279791881,16.100497086391));
#27530=CARTESIAN_POINT('Ctrl Pts',(165.275,0.366870691155206,16.1215115836875));
#27531=CARTESIAN_POINT('Ctrl Pts',(165.275,0.0129443432266137,16.1309839397288));
#27532=CARTESIAN_POINT('Ctrl Pts',(165.275,-0.344797620542512,16.1405584155246));
#27533=CARTESIAN_POINT('Ctrl Pts',(165.275,-0.702475529007602,16.1383406631138));
#27534=CARTESIAN_POINT('Ctrl Pts',(165.275,-1.0594862910395,16.1243561991652));
#27535=CARTESIAN_POINT('Ctrl Pts',(165.275,-1.41672598806189,16.110362767607));
#27536=CARTESIAN_POINT('Ctrl Pts',(165.275,-1.77329827277413,16.0845875753289));
#27537=CARTESIAN_POINT('Ctrl Pts',(165.275,-2.12860531346392,16.0470044590823));
#27538=CARTESIAN_POINT('Ctrl Pts',(165.275,-2.48156963561219,16.0096691472787));
#27539=CARTESIAN_POINT('Ctrl Pts',(165.275,-2.83328591971421,15.9606811019099));
#27540=CARTESIAN_POINT('Ctrl Pts',(165.275,-3.18316570596867,15.899963443923));
#27541=CARTESIAN_POINT('Ctrl Pts',(165.275,-3.27197342713428,15.8845518738576));
#27542=CARTESIAN_POINT('Ctrl Pts',(165.275,-3.36066279296193,15.8683843486503));
#27543=CARTESIAN_POINT('Ctrl Pts',(165.275,-3.44922408738302,15.8514590814298));
#27544=CARTESIAN_POINT('Ctrl Pts',(165.275,-3.77824029779051,15.7885796111442));
#27545=CARTESIAN_POINT('Ctrl Pts',(165.275,-4.10548981858235,15.7152446356181));
#27546=CARTESIAN_POINT('Ctrl Pts',(165.275,-4.43054112840097,15.6316478807662));
#27547=CARTESIAN_POINT('Ctrl Pts',(165.275,-4.57275107644662,15.5950743005185));
#27548=CARTESIAN_POINT('Ctrl Pts',(165.275,-4.71454010907513,15.5565360566608));
#27549=CARTESIAN_POINT('Ctrl Pts',(165.275,-4.85587119547362,15.5160471135189));
#27550=CARTESIAN_POINT('Ctrl Pts',(165.275,-4.919203717467,15.4979034273181));
#27551=CARTESIAN_POINT('Ctrl Pts',(165.275,-4.98244427245377,15.4793680096898));
#27552=CARTESIAN_POINT('Ctrl Pts',(165.275,-5.0455894852499,15.4604420305817));
#27553=CARTESIAN_POINT('Ctrl Pts',(165.275,-5.08079450446641,15.4498903287394));
#27554=CARTESIAN_POINT('Ctrl Pts',(165.275,-5.11597091270945,15.4392168784065));
#27555=CARTESIAN_POINT('Ctrl Pts',(165.275,-5.15110172385917,15.428427010299));
#27556=CARTESIAN_POINT('Ctrl Pts',(165.275,-5.49109545342158,15.3240033611059));
#27557=CARTESIAN_POINT('Ctrl Pts',(165.275,-5.82717408722056,15.2085747292738));
#27558=CARTESIAN_POINT('Ctrl Pts',(165.275,-6.15885764664904,15.0825065615621));
#27559=CARTESIAN_POINT('Ctrl Pts',(165.275,-6.49404462112913,14.9551067959954));
#27560=CARTESIAN_POINT('Ctrl Pts',(165.275,-6.8247437019426,14.8168413986741));
#27561=CARTESIAN_POINT('Ctrl Pts',(165.275,-7.15045388014768,14.6680345158102));
#27562=CARTESIAN_POINT('Ctrl Pts',(165.275,-7.4782000433185,14.5182974545343));
#27563=CARTESIAN_POINT('Ctrl Pts',(165.275,-7.80089527981772,14.3578865204932));
#27564=CARTESIAN_POINT('Ctrl Pts',(165.275,-8.11801542201978,14.1870811873578));
#27565=CARTESIAN_POINT('Ctrl Pts',(165.275,-8.43434950295579,14.0166992377875));
#27566=CARTESIAN_POINT('Ctrl Pts',(165.275,-8.74513661663318,13.8359741036879));
#27567=CARTESIAN_POINT('Ctrl Pts',(165.275,-9.0498349367311,13.6451362127275));
#27568=CARTESIAN_POINT('Ctrl Pts',(165.275,-9.35071161395233,13.4566918835904));
#27569=CARTESIAN_POINT('Ctrl Pts',(165.275,-9.64565173079618,13.2583865792843));
#27570=CARTESIAN_POINT('Ctrl Pts',(165.275,-9.93410536768225,13.0504005429416));
#27571=CARTESIAN_POINT('Ctrl Pts',(165.275,-10.1851298454741,12.8694023529914));
#27572=CARTESIAN_POINT('Ctrl Pts',(165.275,-10.4312417515381,12.6810720241504));
#27573=CARTESIAN_POINT('Ctrl Pts',(165.275,-10.6720568218315,12.4855047231419));
#27574=CARTESIAN_POINT('',(165.275,-16.4196180283464,-0.4237456136972));
#27575=CARTESIAN_POINT('Origin',(165.275,0.,0.));
#27576=CARTESIAN_POINT('Ctrl Pts',(165.275,-16.4196979759281,-0.423941685646876));
#27577=CARTESIAN_POINT('Ctrl Pts',(165.275,-16.4016787090332,-0.7842830862408));
#27578=CARTESIAN_POINT('Ctrl Pts',(165.275,-16.3718071999858,-1.14360257033157));
#27579=CARTESIAN_POINT('Ctrl Pts',(165.275,-16.3300342719941,-1.50131738370712));
#27580=CARTESIAN_POINT('Ctrl Pts',(165.275,-16.3048876264591,-1.71665607426646));
#27581=CARTESIAN_POINT('Ctrl Pts',(165.275,-16.2754270872509,-1.93141328547431));
#27582=CARTESIAN_POINT('Ctrl Pts',(165.275,-16.2416328313117,-2.14546118660578));
#27583=CARTESIAN_POINT('Ctrl Pts',(165.275,-16.1854012842414,-2.50162362584976));
#27584=CARTESIAN_POINT('Ctrl Pts',(165.275,-16.1171736810049,-2.8558230812008));
#27585=CARTESIAN_POINT('Ctrl Pts',(165.275,-16.0372020629593,-3.20751222574865));
#27586=CARTESIAN_POINT('Ctrl Pts',(165.275,-15.9730634874233,-3.48957280316338));
#27587=CARTESIAN_POINT('Ctrl Pts',(165.275,-15.9013697500682,-3.77001858374566));
#27588=CARTESIAN_POINT('Ctrl Pts',(165.275,-15.8222281138278,-4.04855891945055));
#27589=CARTESIAN_POINT('Ctrl Pts',(165.275,-15.7876036479726,-4.17042031632144));
#27590=CARTESIAN_POINT('Ctrl Pts',(165.275,-15.7515533546878,-4.29191688532063));
#27591=CARTESIAN_POINT('Ctrl Pts',(165.275,-15.7140850611406,-4.4130236967691));
#27592=CARTESIAN_POINT('Ctrl Pts',(165.275,-15.697964022471,-4.46513088942947));
#27593=CARTESIAN_POINT('Ctrl Pts',(165.275,-15.6815804720113,-4.51716592437791));
#27594=CARTESIAN_POINT('Ctrl Pts',(165.275,-15.6649349944356,-4.56912679247947));
#27595=CARTESIAN_POINT('Ctrl Pts',(165.275,-15.6521437038709,-4.60905635045434));
#27596=CARTESIAN_POINT('Ctrl Pts',(165.275,-15.6391978329378,-4.64894170388832));
#27597=CARTESIAN_POINT('Ctrl Pts',(165.275,-15.6261020029682,-4.68876902426644));
#27598=CARTESIAN_POINT('Ctrl Pts',(165.275,-15.5139349861521,-5.02989377351528));
#27599=CARTESIAN_POINT('Ctrl Pts',(165.275,-15.390693116279,-5.36700737179514));
#27600=CARTESIAN_POINT('Ctrl Pts',(165.275,-15.2566512779005,-5.6995802871865));
#27601=CARTESIAN_POINT('Ctrl Pts',(165.275,-15.1216679786648,-6.03448907312229));
#27602=CARTESIAN_POINT('Ctrl Pts',(165.275,-14.9757322691986,-6.36479373098975));
#27603=CARTESIAN_POINT('Ctrl Pts',(165.275,-14.8190753781778,-6.6899343455592));
#27604=CARTESIAN_POINT('Ctrl Pts',(165.275,-14.6642395982279,-7.01129525296781));
#27605=CARTESIAN_POINT('Ctrl Pts',(165.275,-14.4989301264842,-7.32761195534377));
#27606=CARTESIAN_POINT('Ctrl Pts',(165.275,-14.3233261861414,-7.6383175684349));
#27607=CARTESIAN_POINT('Ctrl Pts',(165.275,-14.2339751831176,-7.79641116314956));
#27608=CARTESIAN_POINT('Ctrl Pts',(165.275,-14.1419582748423,-7.95305158643488));
#27609=CARTESIAN_POINT('Ctrl Pts',(165.275,-14.0472950161733,-8.10816090472558));
#27610=CARTESIAN_POINT('Ctrl Pts',(165.275,-13.99716261779,-8.19030472955101));
#27611=CARTESIAN_POINT('Ctrl Pts',(165.275,-13.9462879739077,-8.27201909773014));
#27612=CARTESIAN_POINT('Ctrl Pts',(165.275,-13.8946736934634,-8.3532921496216));
#27613=CARTESIAN_POINT('Ctrl Pts',(165.275,-13.8648492679751,-8.40025438680618));
#27614=CARTESIAN_POINT('Ctrl Pts',(165.275,-13.8347743088155,-8.44707466778208));
#27615=CARTESIAN_POINT('Ctrl Pts',(165.275,-13.8044685328867,-8.4937213499452));
#27616=CARTESIAN_POINT('Ctrl Pts',(165.275,-13.6097249156417,-8.79347093029817));
#27617=CARTESIAN_POINT('Ctrl Pts',(165.275,-13.4053424511432,-9.08623483394262));
#27618=CARTESIAN_POINT('Ctrl Pts',(165.275,-13.1915764793124,-9.37149790563643));
#27619=CARTESIAN_POINT('Ctrl Pts',(165.275,-13.1700547684607,-9.40021786182532));
#27620=CARTESIAN_POINT('Ctrl Pts',(165.275,-13.1484379053149,-9.42886176822469));
#27621=CARTESIAN_POINT('Ctrl Pts',(165.275,-13.1267261246103,-9.45742908533937));
#27622=CARTESIAN_POINT('Ctrl Pts',(165.275,-12.9120131061372,-9.73993815130696));
#27623=CARTESIAN_POINT('Ctrl Pts',(165.275,-12.6880210207321,-10.0149595594262));
#27624=CARTESIAN_POINT('Ctrl Pts',(165.275,-12.4552583907319,-10.2821767885852));
#27625=CARTESIAN_POINT('Ctrl Pts',(165.275,-12.2211760823525,-10.55090904101));
#27626=CARTESIAN_POINT('Ctrl Pts',(165.275,-11.9782230602433,-10.8117487534477));
#27627=CARTESIAN_POINT('Ctrl Pts',(165.275,-11.7268764081748,-11.0643393372962));
#27628=CARTESIAN_POINT('Ctrl Pts',(165.275,-11.4755860591534,-11.31687333945));
#27629=CARTESIAN_POINT('Ctrl Pts',(165.275,-11.2159053710805,-11.5611622650247));
#27630=CARTESIAN_POINT('Ctrl Pts',(165.275,-10.9482779591041,-11.7968097141648));
#27631=CARTESIAN_POINT('Ctrl Pts',(165.275,-10.6822726193024,-12.0310289195855));
#27632=CARTESIAN_POINT('Ctrl Pts',(165.275,-10.4084161143014,-12.256711394371));
#27633=CARTESIAN_POINT('Ctrl Pts',(165.275,-10.1271184072732,-12.4734233996839));
#27634=CARTESIAN_POINT('Ctrl Pts',(165.275,-10.006146678876,-12.5666201275353));
#27635=CARTESIAN_POINT('Ctrl Pts',(165.275,-9.88379847902285,-12.658157250573));
#27636=CARTESIAN_POINT('Ctrl Pts',(165.275,-9.76010527741534,-12.7479974951101));
#27637=CARTESIAN_POINT('Ctrl Pts',(165.275,-9.69762926093608,-12.7933747715105));
#27638=CARTESIAN_POINT('Ctrl Pts',(165.275,-9.63481010553126,-12.8383191222954));
#27639=CARTESIAN_POINT('Ctrl Pts',(165.275,-9.57165181189903,-12.8828255728729));
#27640=CARTESIAN_POINT('Ctrl Pts',(165.275,-9.53441395349683,-12.909066384796));
#27641=CARTESIAN_POINT('Ctrl Pts',(165.275,-9.49705465291021,-12.9351573739713));
#27642=CARTESIAN_POINT('Ctrl Pts',(165.275,-9.4595980405967,-12.9610815227979));
#27643=CARTESIAN_POINT('Ctrl Pts',(165.275,-9.16782661633503,-13.1630198551436));
#27644=CARTESIAN_POINT('Ctrl Pts',(165.275,-8.86990154943769,-13.355018095262));
#27645=CARTESIAN_POINT('Ctrl Pts',(165.275,-8.56630677828613,-13.5367564639103));
#27646=CARTESIAN_POINT('Ctrl Pts',(165.275,-8.26294806373811,-13.7183535239917));
#27647=CARTESIAN_POINT('Ctrl Pts',(165.275,-7.95392798018689,-13.8897069930093));
#27648=CARTESIAN_POINT('Ctrl Pts',(165.275,-7.6396980471573,-14.0504565393865));
#27649=CARTESIAN_POINT('Ctrl Pts',(165.275,-7.42828741870809,-14.158607161114));
#27650=CARTESIAN_POINT('Ctrl Pts',(165.275,-7.21451793583355,-14.2619571046843));
#27651=CARTESIAN_POINT('Ctrl Pts',(165.275,-6.99852075110882,-14.3603849559975));
#27652=CARTESIAN_POINT('Ctrl Pts',(165.275,-6.6767756444455,-14.5070011239802));
#27653=CARTESIAN_POINT('Ctrl Pts',(165.275,-6.3500881152452,-14.6426982553463));
#27654=CARTESIAN_POINT('Ctrl Pts',(165.275,-6.01904765523771,-14.7673776954759));
#27655=CARTESIAN_POINT('Ctrl Pts',(165.275,-5.68839318247852,-14.8919117616109));
#27656=CARTESIAN_POINT('Ctrl Pts',(165.275,-5.35339533712104,-15.0054539045506));
#27657=CARTESIAN_POINT('Ctrl Pts',(165.275,-5.01463099442199,-15.1078550161438));
#27658=CARTESIAN_POINT('Ctrl Pts',(165.275,-4.78696415456429,-15.176673762794));
#27659=CARTESIAN_POINT('Ctrl Pts',(165.275,-4.55759595885986,-15.2404595893394));
#27660=CARTESIAN_POINT('Ctrl Pts',(165.275,-4.32670083368095,-15.2991539971731));
#27661=CARTESIAN_POINT('Ctrl Pts',(165.275,-4.22568421641518,-15.3248328006003));
#27662=CARTESIAN_POINT('Ctrl Pts',(165.275,-4.1243753377578,-15.3495369356427));
#27663=CARTESIAN_POINT('Ctrl Pts',(165.275,-4.02278884229152,-15.373260849648));
#27664=CARTESIAN_POINT('Ctrl Pts',(165.275,-3.98236618547463,-15.3827009197064));
#27665=CARTESIAN_POINT('Ctrl Pts',(165.275,-3.94189957256296,-15.3919857817139));
#27666=CARTESIAN_POINT('Ctrl Pts',(165.275,-3.90138992826692,-15.4011150681005));
#27667=CARTESIAN_POINT('Ctrl Pts',(165.275,-3.86736893591951,-15.4087820666065));
#27668=CARTESIAN_POINT('Ctrl Pts',(165.275,-3.83331718190531,-15.4163393952635));
#27669=CARTESIAN_POINT('Ctrl Pts',(165.275,-3.79925018272408,-15.4237836538925));
#27670=CARTESIAN_POINT('Ctrl Pts',(165.275,-3.45655389291593,-15.4986690231305));
#27671=CARTESIAN_POINT('Ctrl Pts',(165.275,-3.11194988903074,-15.5622000687083));
#27672=CARTESIAN_POINT('Ctrl Pts',(165.275,-2.76602256136856,-15.6143425165745));
#27673=CARTESIAN_POINT('Ctrl Pts',(165.275,-2.41816781747772,-15.6667754884675));
#27674=CARTESIAN_POINT('Ctrl Pts',(165.275,-2.06897438754626,-15.7076927214654));
#27675=CARTESIAN_POINT('Ctrl Pts',(165.275,-1.71902298233414,-15.7370087185928));
#27676=CARTESIAN_POINT('Ctrl Pts',(165.275,-1.36998651456403,-15.7662480699259));
#27677=CARTESIAN_POINT('Ctrl Pts',(165.275,-1.02019544917748,-15.7839468280107));
#27678=CARTESIAN_POINT('Ctrl Pts',(165.275,-0.670221251270087,-15.7899686712479));
#27679=CARTESIAN_POINT('Ctrl Pts',(165.275,-0.32390640711229,-15.7959275496874));
#27680=CARTESIAN_POINT('Ctrl Pts',(165.275,0.0225883051757998,-15.7904524237367));
#27681=CARTESIAN_POINT('Ctrl Pts',(165.275,0.368705405399811,-15.7733603902667));
#27682=CARTESIAN_POINT('Ctrl Pts',(165.275,0.453570607697479,-15.7691695575191));
#27683=CARTESIAN_POINT('Ctrl Pts',(165.275,0.538413068762913,-15.7642800840483));
#27684=CARTESIAN_POINT('Ctrl Pts',(165.275,0.623224478572632,-15.7586888003296));
#27685=CARTESIAN_POINT('Ctrl Pts',(165.275,0.944160774763383,-15.7375307286545));
#27686=CARTESIAN_POINT('Ctrl Pts',(165.275,1.26465339880877,-15.7063257144656));
#27687=CARTESIAN_POINT('Ctrl Pts',(165.275,1.58426253506222,-15.6651777123449));
#27688=CARTESIAN_POINT('Ctrl Pts',(165.275,1.7240915321731,-15.647175461417));
#27689=CARTESIAN_POINT('Ctrl Pts',(165.275,1.86375126122269,-15.6272696157382));
#27690=CARTESIAN_POINT('Ctrl Pts',(165.275,2.00320401000376,-15.6054668437631));
#27691=CARTESIAN_POINT('Ctrl Pts',(165.275,2.05798321167464,-15.5969023769208));
#27692=CARTESIAN_POINT('Ctrl Pts',(165.275,2.11273046877317,-15.5880451935127));
#27693=CARTESIAN_POINT('Ctrl Pts',(165.275,2.16744346830565,-15.5788956468138));
#27694=CARTESIAN_POINT('Ctrl Pts',(165.275,2.21749764255649,-15.5705251862524));
#27695=CARTESIAN_POINT('Ctrl Pts',(165.275,2.26752960855478,-15.5619088337655));
#27696=CARTESIAN_POINT('Ctrl Pts',(165.275,2.31750237759088,-15.5530532358352));
#27697=CARTESIAN_POINT('Ctrl Pts',(165.275,2.65884602114199,-15.4925642511012));
#27698=CARTESIAN_POINT('Ctrl Pts',(165.275,2.99767177970771,-15.4208793715129));
#27699=CARTESIAN_POINT('Ctrl Pts',(165.275,3.3334593644421,-15.3382643317085));
#27700=CARTESIAN_POINT('Ctrl Pts',(165.275,3.67183663894271,-15.2550121411194));
#27701=CARTESIAN_POINT('Ctrl Pts',(165.275,4.00712925195428,-15.1606604008729));
#27702=CARTESIAN_POINT('Ctrl Pts',(165.275,4.3387978893757,-15.0554285812879));
#27703=CARTESIAN_POINT('Ctrl Pts',(165.275,4.67063218389584,-14.9501442020215));
#27704=CARTESIAN_POINT('Ctrl Pts',(165.275,4.99883943284626,-14.8339686718481));
#27705=CARTESIAN_POINT('Ctrl Pts',(165.275,5.32286432386021,-14.7070721822145));
#27706=CARTESIAN_POINT('Ctrl Pts',(165.275,5.64507264113224,-14.5808871096274));
#27707=CARTESIAN_POINT('Ctrl Pts',(165.275,5.96314588179039,-14.4441007160084));
#27708=CARTESIAN_POINT('Ctrl Pts',(165.275,6.2765150505169,-14.2968346236721));
#27709=CARTESIAN_POINT('Ctrl Pts',(165.275,6.58483133506045,-14.1519431060639));
#27710=CARTESIAN_POINT('Ctrl Pts',(165.275,6.88859445447486,-13.9969068404714));
#27711=CARTESIAN_POINT('Ctrl Pts',(165.275,7.1872332756858,-13.8318012043831));
#27712=CARTESIAN_POINT('Ctrl Pts',(165.275,7.42926750920022,-13.6979900142722));
#27713=CARTESIAN_POINT('Ctrl Pts',(165.275,7.66793545463417,-13.5575640477772));
#27714=CARTESIAN_POINT('Ctrl Pts',(165.275,7.90291568084398,-13.4105452217265));
#27715=CARTESIAN_POINT('Ctrl Pts',(149.504027251253,-6.69583157622459,14.052211174948));
#27716=CARTESIAN_POINT('Ctrl Pts',(149.543258526747,-9.00505367639947,12.9518745757918));
#27717=CARTESIAN_POINT('Ctrl Pts',(149.621721077736,-13.0684824505813,9.59211511216706));
#27718=CARTESIAN_POINT('Ctrl Pts',(149.739414904219,-16.0518724299814,2.26397071243674));
#27719=CARTESIAN_POINT('Ctrl Pts',(149.857108730702,-15.2118889326799,-5.60192652569123));
#27720=CARTESIAN_POINT('Ctrl Pts',(149.974802557185,-10.7492384929991,-12.1343631343868));
#27721=CARTESIAN_POINT('Ctrl Pts',(150.092496383669,-3.72643497720167,-15.7765283006024));
#27722=CARTESIAN_POINT('Ctrl Pts',(150.210190210152,4.18380951624729,-15.6615050736542));
#27723=CARTESIAN_POINT('Ctrl Pts',(150.327884036635,11.0976583641875,-11.8164414573133));
#27724=CARTESIAN_POINT('Ctrl Pts',(150.445577863118,15.3684657582085,-5.15720159382155));
#27725=CARTESIAN_POINT('Ctrl Pts',(150.563271689601,15.9791097813677,2.73030173509255));
#27726=CARTESIAN_POINT('Ctrl Pts',(150.680965516085,12.7841501358716,9.96754432364079));
#27727=CARTESIAN_POINT('Ctrl Pts',(150.798659342568,6.54450585940981,14.8309111095575));
#27728=CARTESIAN_POINT('Ctrl Pts',(150.916353169051,-1.25378517594862,16.1621310075655));
#27729=CARTESIAN_POINT('Ctrl Pts',(151.034046995534,-8.75347314553567,13.6441626527123));
#27730=CARTESIAN_POINT('Ctrl Pts',(151.151740822017,-14.1684253302768,7.87668630506945));
#27731=CARTESIAN_POINT('Ctrl Pts',(151.2694346485,-16.2090110458911,0.233290702127952));
#27732=CARTESIAN_POINT('Ctrl Pts',(151.387128474984,-14.3892424680134,-7.46566577380577));
#27733=CARTESIAN_POINT('Ctrl Pts',(151.504822301467,-9.14251744982534,-13.3865917383038));
#27734=CARTESIAN_POINT('Ctrl Pts',(151.62251612795,-1.71840131299559,-16.1193536145945));
#27735=CARTESIAN_POINT('Ctrl Pts',(151.740209954433,6.11497100889316,-15.0131140483778));
#27736=CARTESIAN_POINT('Ctrl Pts',(151.857903780916,12.491995698527,-10.3313361861333));
#27737=CARTESIAN_POINT('Ctrl Pts',(151.9755976074,15.8939141615272,-3.18903692982364));
#27738=CARTESIAN_POINT('Ctrl Pts',(152.093291433883,15.510522082331,4.71276655929273));
#27739=CARTESIAN_POINT('Ctrl Pts',(152.210985260366,11.4331285039078,11.4921728375615));
#27740=CARTESIAN_POINT('Ctrl Pts',(152.328679086849,4.63280957101442,15.5345917033455));
#27741=CARTESIAN_POINT('Ctrl Pts',(152.446372913332,-3.2708639369447,15.8772766247591));
#27742=CARTESIAN_POINT('Ctrl Pts',(152.564066739816,-10.3955452083385,12.4386134168428));
#27743=CARTESIAN_POINT('Ctrl Pts',(152.681760566299,-15.0444130039594,6.03755755904503));
#27744=CARTESIAN_POINT('Ctrl Pts',(152.799454392782,-16.1102883058211,-1.80140906399063));
#27745=CARTESIAN_POINT('Ctrl Pts',(152.917148219265,-13.3393211827226,-9.21135029713916));
#27746=CARTESIAN_POINT('Ctrl Pts',(153.034842045748,-7.39144794457472,-14.4275071025847));
#27747=CARTESIAN_POINT('Ctrl Pts',(153.152535872232,0.316779951246796,-16.2075943426206));
#27748=CARTESIAN_POINT('Ctrl Pts',(153.270229698715,7.94956321608139,-14.1276646543581));
#27749=CARTESIAN_POINT('Ctrl Pts',(153.387923525198,13.689070530273,-8.68307617896328));
#27750=CARTESIAN_POINT('Ctrl Pts',(153.505617351681,16.1683750739281,-1.17051756981636));
#27751=CARTESIAN_POINT('Ctrl Pts',(153.623311178164,14.7970031896607,6.62081267803603));
#27752=CARTESIAN_POINT('Ctrl Pts',(153.741005004647,9.90156218120505,12.8353235364053));
#27753=CARTESIAN_POINT('Ctrl Pts',(153.858698831131,2.64795519030276,15.9929608647873));
#27754=CARTESIAN_POINT('Ctrl Pts',(153.976392657614,-5.23629146518378,15.3416985892734));
#27755=CARTESIAN_POINT('Ctrl Pts',(154.094086484097,-11.8734576922091,11.0366419867544));
#27756=CARTESIAN_POINT('Ctrl Pts',(154.21178031058,-15.6828293236568,4.1030876565728));
#27757=CARTESIAN_POINT('Ctrl Pts',(154.329474137063,-15.757162590172,-3.80766214616699));
#27758=CARTESIAN_POINT('Ctrl Pts',(154.447167963547,-12.0787542064295,-10.8115753122814));
#27759=CARTESIAN_POINT('Ctrl Pts',(154.56486179003,-5.52365760332652,-15.2405928557154));
#27760=CARTESIAN_POINT('Ctrl Pts',(154.682555616513,2.34695883598703,-16.039895515079));
#27761=CARTESIAN_POINT('Ctrl Pts',(154.800249442996,9.65862120442349,-13.0191205671478));
#27762=CARTESIAN_POINT('Ctrl Pts',(154.917943269479,14.6699766571649,-6.8976988040002));
#27763=CARTESIAN_POINT('Ctrl Pts',(155.035637095963,16.1875157521321,0.86648582616573));
#27764=CARTESIAN_POINT('Ctrl Pts',(155.153330922446,13.8498198560533,8.4243073227026));
#27765=CARTESIAN_POINT('Ctrl Pts',(155.271024748929,8.21363696874461,13.9757873358942));
#27766=CARTESIAN_POINT('Ctrl Pts',(155.388718575412,0.621286060936392,16.1987798164848));
#27767=CARTESIAN_POINT('Ctrl Pts',(155.506412401895,-7.11903095842639,14.563854645163));
#27768=CARTESIAN_POINT('Ctrl Pts',(155.624106228379,-13.1638724228295,9.4603872409082));
#27769=CARTESIAN_POINT('Ctrl Pts',(155.741800054862,-16.0735928248502,2.10382452058001));
#27770=CARTESIAN_POINT('Ctrl Pts',(155.859493881345,-15.1552102344754,-5.75378715815253));
#27771=CARTESIAN_POINT('Ctrl Pts',(155.977187707828,-10.6274475707617,-12.2410711150283));
#27772=CARTESIAN_POINT('Ctrl Pts',(156.094881534311,-3.56864133200721,-15.8130092947535));
#27773=CARTESIAN_POINT('Ctrl Pts',(156.212575360794,4.34007610648377,-15.6189053170316));
#27774=CARTESIAN_POINT('Ctrl Pts',(156.330269187278,11.215156665436,-11.7049871799245));
#27775=CARTESIAN_POINT('Ctrl Pts',(156.447963013761,15.4192242617626,-5.00339755345713));
#27776=CARTESIAN_POINT('Ctrl Pts',(156.565656840244,15.9510339391494,2.88980625381255));
#27777=CARTESIAN_POINT('Ctrl Pts',(156.683350666727,12.6839293713117,10.0947709045845));
#27778=CARTESIAN_POINT('Ctrl Pts',(156.80104449321,6.39600745972602,14.8955547895202));
#27779=CARTESIAN_POINT('Ctrl Pts',(156.918738319694,-1.41519400502264,16.1487984023771));
#27780=CARTESIAN_POINT('Ctrl Pts',(157.036432146177,-8.88935144579475,13.5560279870475));
#27781=CARTESIAN_POINT('Ctrl Pts',(157.15412597266,-14.246412028328,7.7347403467461));
#27782=CARTESIAN_POINT('Ctrl Pts',(157.271819799143,-16.2105328300161,0.071339185875412));
#27783=CARTESIAN_POINT('Ctrl Pts',(157.389513625626,-14.3139368702984,-7.60905218707177));
#27784=CARTESIAN_POINT('Ctrl Pts',(157.507207452109,-9.00831934563013,-13.4772640576497));
#27785=CARTESIAN_POINT('Ctrl Pts',(157.624901278593,-1.55727144834802,-16.135717199698));
#27786=CARTESIAN_POINT('Ctrl Pts',(157.742595105076,6.26465777934683,-14.9512717459131));
#27787=CARTESIAN_POINT('Ctrl Pts',(157.860288931559,12.5945898255295,-10.2060164138188));
#27788=CARTESIAN_POINT('Ctrl Pts',(157.977982758042,15.9249817238141,-3.03008597380632));
#27789=CARTESIAN_POINT('Ctrl Pts',(158.095676584526,15.4626639986145,4.86749278154799));
#27790=CARTESIAN_POINT('Ctrl Pts',(158.213370411009,11.3177427031671,11.6058245729193));
#27791=CARTESIAN_POINT('Ctrl Pts',(158.331064237492,4.47737645143262,15.5801015408959));
#27792=CARTESIAN_POINT('Ctrl Pts',(158.448758063975,-3.42932626773513,15.8438058957402));
#27793=CARTESIAN_POINT('Ctrl Pts',(158.566451890458,-10.5192972026361,12.3341335437509));
#27794=CARTESIAN_POINT('Ctrl Pts',(158.684145716941,-15.1039817626669,5.886951573225));
#27795=CARTESIAN_POINT('Ctrl Pts',(158.801839543424,-16.0914868735976,-1.96227268984356));
#27796=CARTESIAN_POINT('Ctrl Pts',(158.919533369908,-13.2466273275316,-9.34416012052252));
#27797=CARTESIAN_POINT('Ctrl Pts',(159.037227196391,-7.24693772795856,-14.5006330027196));
#27798=CARTESIAN_POINT('Ctrl Pts',(159.154921022874,0.478689831123546,-16.2036205817727));
#27799=CARTESIAN_POINT('Ctrl Pts',(159.272614849357,8.0903121397976,-14.0475376273962));
#27800=CARTESIAN_POINT('Ctrl Pts',(159.390308675841,13.7751375929553,-8.54587901901382));
#27801=CARTESIAN_POINT('Ctrl Pts',(159.508002502324,16.1792624575846,-1.00892529013043));
#27802=CARTESIAN_POINT('Ctrl Pts',(159.625696328807,14.7301179440772,6.76831509801693));
#27803=CARTESIAN_POINT('Ctrl Pts',(159.74339015529,9.77283376357005,12.9336067723623));
#27804=CARTESIAN_POINT('Ctrl Pts',(159.861083981773,2.48804168970207,16.0186176826459));
#27805=CARTESIAN_POINT('Ctrl Pts',(159.978777808256,-5.3893048890199,15.2886185355531));
#27806=CARTESIAN_POINT('Ctrl Pts',(160.09647163474,-11.9831292087549,10.9174666602997));
#27807=CARTESIAN_POINT('Ctrl Pts',(160.214165461223,-15.7230394545078,3.94619997269045));
#27808=CARTESIAN_POINT('Ctrl Pts',(160.331859287706,-15.7183348502254,-3.9648976592919));
#27809=CARTESIAN_POINT('Ctrl Pts',(160.449553114189,-11.9701358491835,-10.9317112871024));
#27810=CARTESIAN_POINT('Ctrl Pts',(160.567246940672,-5.37111728571021,-15.2950175879472));
#27811=CARTESIAN_POINT('Ctrl Pts',(160.684940767156,2.50709195889985,-16.0156471558938));
#27812=CARTESIAN_POINT('Ctrl Pts',(160.802634593639,9.78820966743234,-12.9219741300954));
#27813=CARTESIAN_POINT('Ctrl Pts',(160.920328420122,14.7381575419149,-6.75079078198745));
#27814=CARTESIAN_POINT('Ctrl Pts',(161.038022246605,16.1780510307112,1.02816767123628));
#27815=CARTESIAN_POINT('Ctrl Pts',(161.155716073088,13.7649636560103,8.56225668040771));
#27816=CARTESIAN_POINT('Ctrl Pts',(161.273409899572,8.07359872781038,14.0571500488103));
#27817=CARTESIAN_POINT('Ctrl Pts',(161.391103726055,0.459417427060223,16.2041784592796));
#27818=CARTESIAN_POINT('Ctrl Pts',(161.508797552538,-7.2641791890122,14.4920034716527));
#27819=CARTESIAN_POINT('Ctrl Pts',(161.626491379021,-13.2577316019136,9.32839839865786));
#27820=CARTESIAN_POINT('Ctrl Pts',(161.744185205504,-16.0938093561825,1.94313260467315));
#27821=CARTESIAN_POINT('Ctrl Pts',(161.861879031987,-15.0969693286697,-5.90491159981625));
#27822=CARTESIAN_POINT('Ctrl Pts',(161.979572858471,-10.5046199403779,-12.3466361338107));
#27823=CARTESIAN_POINT('Ctrl Pts',(162.097266684954,-3.41047972870878,-15.8478734198804));
#27824=CARTESIAN_POINT('Ctrl Pts',(162.214960511437,4.49590375656297,-15.5747652734798));
#27825=CARTESIAN_POINT('Ctrl Pts',(162.33265433792,11.3315382928711,-11.5923554047623));
#27826=CARTESIAN_POINT('Ctrl Pts',(162.450348164404,15.4684423013133,-4.84909854322174));
#27827=CARTESIAN_POINT('Ctrl Pts',(162.568041990887,15.9213665733349,3.04902449198908));
#27828=CARTESIAN_POINT('Ctrl Pts',(162.68573581737,12.5824422093376,10.2209887954907));
#27829=CARTESIAN_POINT('Ctrl Pts',(162.803429643853,6.24687078672089,14.9587121533836));
#27830=CARTESIAN_POINT('Ctrl Pts',(162.921123470336,-1.57646165108159,16.1338536185746));
#27831=CARTESIAN_POINT('Ctrl Pts',(163.038817296819,-9.02434239708718,13.466540319226));
#27832=CARTESIAN_POINT('Ctrl Pts',(163.156511123303,-14.3229767115452,7.59202226981592));
#27833=CARTESIAN_POINT('Ctrl Pts',(163.274204949786,-16.2104365088772,-0.0906194242304325));
#27834=CARTESIAN_POINT('Ctrl Pts',(163.391898776269,-14.2372025145188,-7.75167909617249));
#27835=CARTESIAN_POINT('Ctrl Pts',(163.509592602752,-8.87322202528032,-13.5665911166955));
#27836=CARTESIAN_POINT('Ctrl Pts',(163.627286429235,-1.39598620207817,-16.1504701483178));
#27837=CARTESIAN_POINT('Ctrl Pts',(163.744980255718,6.413719352529,-14.8879370857845));
#27838=CARTESIAN_POINT('Ctrl Pts',(163.862674082202,12.6959265445113,-10.0796778296488));
#27839=CARTESIAN_POINT('Ctrl Pts',(163.980367908685,15.9544602156426,-2.87083272081841));
#27840=CARTESIAN_POINT('Ctrl Pts',(164.098061735168,15.4132614171153,5.0217334684266));
#27841=CARTESIAN_POINT('Ctrl Pts',(164.215755561651,11.2012293687092,11.7183171829071));
#27842=CARTESIAN_POINT('Ctrl Pts',(164.333449388134,4.32149195873656,15.6240575808949));
#27843=CARTESIAN_POINT('Ctrl Pts',(164.451143214618,-3.58743715586971,15.8087508847164));
#27844=CARTESIAN_POINT('Ctrl Pts',(164.568837041101,-10.6420179340868,12.2284282526787));
#27845=CARTESIAN_POINT('Ctrl Pts',(164.686530867584,-15.1620044343422,5.73574619313003));
#27846=CARTESIAN_POINT('Ctrl Pts',(164.804224694067,-16.0711581199633,-2.12291628183429));
#27847=CARTESIAN_POINT('Ctrl Pts',(164.92191852055,-13.1524493936104,-9.4760867792538));
#27848=CARTESIAN_POINT('Ctrl Pts',(165.039612347034,-7.10203868245562,-14.5722070548038));
#27849=CARTESIAN_POINT('Ctrl Pts',(165.157306173517,0.641239642833148,-16.1982319284135));
#27850=CARTESIAN_POINT('Ctrl Pts',(165.235768724506,5.69913956220702,-14.7092438620197));
#27851=CARTESIAN_POINT('Ctrl Pts',(165.275,7.90291568084474,-13.410545221726));
#27852=CARTESIAN_POINT('Ctrl Pts',(149.669351500835,-6.81900757074158,14.3107145537939));
#27853=CARTESIAN_POINT('Ctrl Pts',(149.708582776329,-9.17070994024695,13.1901362485313));
#27854=CARTESIAN_POINT('Ctrl Pts',(149.787045327318,-13.3088892326745,9.76857091231863));
#27855=CARTESIAN_POINT('Ctrl Pts',(149.904739153801,-16.3471614210372,2.30561854077401));
#27856=CARTESIAN_POINT('Ctrl Pts',(150.022432980285,-15.491725652949,-5.70497912836769));
#27857=CARTESIAN_POINT('Ctrl Pts',(150.140126806768,-10.946980644456,-12.3575859305239));
#27858=CARTESIAN_POINT('Ctrl Pts',(150.257820633251,-3.79498618388818,-16.0667520825673));
#27859=CARTESIAN_POINT('Ctrl Pts',(150.375514459734,4.26077454921843,-15.9496128973232));
#27860=CARTESIAN_POINT('Ctrl Pts',(150.493208286218,11.301810020372,-12.033815791119));
#27861=CARTESIAN_POINT('Ctrl Pts',(150.610902112701,15.6511828535263,-5.25207307139863));
#27862=CARTESIAN_POINT('Ctrl Pts',(150.728595939184,16.2730602364247,2.78052815248715));
#27863=CARTESIAN_POINT('Ctrl Pts',(150.846289765667,13.0193263629189,10.1509064902335));
#27864=CARTESIAN_POINT('Ctrl Pts',(150.96398359215,6.6648980778637,15.103739391559));
#27865=CARTESIAN_POINT('Ctrl Pts',(151.081677418633,-1.27684971008452,16.4594483067999));
#27866=CARTESIAN_POINT('Ctrl Pts',(151.199371245116,-8.9145013535939,13.8951596028249));
#27867=CARTESIAN_POINT('Ctrl Pts',(151.3170650716,-14.429066575644,8.02158521091566));
#27868=CARTESIAN_POINT('Ctrl Pts',(151.434758898083,-16.5071907466476,0.237582299656825));
#27869=CARTESIAN_POINT('Ctrl Pts',(151.552452724566,-14.6539458481936,-7.60300357807271));
#27870=CARTESIAN_POINT('Ctrl Pts',(151.670146551049,-9.31070248650847,-13.6328504339994));
#27871=CARTESIAN_POINT('Ctrl Pts',(151.787840377532,-1.75001288928721,-16.41588398425));
#27872=CARTESIAN_POINT('Ctrl Pts',(151.905534204016,6.22746153779737,-15.289294121406));
#27873=CARTESIAN_POINT('Ctrl Pts',(152.023228030499,12.7217974753715,-10.5213906394047));
#27874=CARTESIAN_POINT('Ctrl Pts',(152.140921856982,16.1862973646181,-3.24770220401861));
#27875=CARTESIAN_POINT('Ctrl Pts',(152.258615683465,15.7958524346883,4.79946224469923));
#27876=CARTESIAN_POINT('Ctrl Pts',(152.376309509948,11.6434514425716,11.7035819511739));
#27877=CARTESIAN_POINT('Ctrl Pts',(152.494003336432,4.71803437391177,15.8203648385703));
#27878=CARTESIAN_POINT('Ctrl Pts',(152.611697162915,-3.33103449436932,16.1693537650236));
#27879=CARTESIAN_POINT('Ctrl Pts',(152.729390989398,-10.5867808457656,12.6674331774043));
#27880=CARTESIAN_POINT('Ctrl Pts',(152.847084815881,-15.321168850129,6.14862399617431));
#27881=CARTESIAN_POINT('Ctrl Pts',(152.964778642365,-16.4066519107647,-1.83454764438394));
#27882=CARTESIAN_POINT('Ctrl Pts',(153.082472468847,-13.5847102929711,-9.38080157750341));
#27883=CARTESIAN_POINT('Ctrl Pts',(153.200166295331,-7.52742044345396,-14.6929143959928));
#27884=CARTESIAN_POINT('Ctrl Pts',(153.317860121814,0.322607410479242,-16.5057479818145));
#27885=CARTESIAN_POINT('Ctrl Pts',(153.435553948297,8.09580275988852,-14.3875560695159));
#27886=CARTESIAN_POINT('Ctrl Pts',(153.55324777478,13.9408936021924,-8.84280936992474));
#27887=CARTESIAN_POINT('Ctrl Pts',(153.670941601264,16.4658072385194,-1.19205031957574));
#27888=CARTESIAN_POINT('Ctrl Pts',(153.788635427747,15.0692077042171,6.74260863076332));
#27889=CARTESIAN_POINT('Ctrl Pts',(153.90632925423,10.0837105454609,13.0714411453305));
#27890=CARTESIAN_POINT('Ctrl Pts',(154.024023080713,2.69666676709334,16.2871661232927));
#27891=CARTESIAN_POINT('Ctrl Pts',(154.141716907196,-5.33261787385496,15.6239232778429));
#27892=CARTESIAN_POINT('Ctrl Pts',(154.25941073368,-12.0918808922171,11.239671190427));
#27893=CARTESIAN_POINT('Ctrl Pts',(154.377104560163,-15.9713294265628,4.17856773652037));
#27894=CARTESIAN_POINT('Ctrl Pts',(154.494798386646,-16.047030122041,-3.87770760150731));
#27895=CARTESIAN_POINT('Ctrl Pts',(154.612492213129,-12.3009540250728,-11.0104642069953));
#27896=CARTESIAN_POINT('Ctrl Pts',(154.730186039612,-5.62527037702249,-15.52095761111));
#27897=CARTESIAN_POINT('Ctrl Pts',(154.847879866096,2.39013330736106,-16.3349641797441));
#27898=CARTESIAN_POINT('Ctrl Pts',(154.965573692578,9.83630044545192,-13.2586192918901));
#27899=CARTESIAN_POINT('Ctrl Pts',(155.083267519062,14.9398444015544,-7.02458833226706));
#27900=CARTESIAN_POINT('Ctrl Pts',(155.200961345545,16.4853000271441,0.88242563172352));
#27901=CARTESIAN_POINT('Ctrl Pts',(155.318655172028,14.1046000600101,8.5792802220024));
#27902=CARTESIAN_POINT('Ctrl Pts',(155.436348998511,8.36473439267312,14.2328848277681));
#27903=CARTESIAN_POINT('Ctrl Pts',(155.554042824995,0.632715190771028,16.4967713043446));
#27904=CARTESIAN_POINT('Ctrl Pts',(155.671736651478,-7.24999209571292,14.8317701773112));
#27905=CARTESIAN_POINT('Ctrl Pts',(155.789430477961,-13.4060339913992,9.63441978543227));
#27906=CARTESIAN_POINT('Ctrl Pts',(155.907124304444,-16.369281382593,2.14252631208443));
#27907=CARTESIAN_POINT('Ctrl Pts',(156.024818130927,-15.4340042978408,-5.85963337715855));
#27908=CARTESIAN_POINT('Ctrl Pts',(156.142511957411,-10.8229492659289,-12.46625690284));
#27909=CARTESIAN_POINT('Ctrl Pts',(156.260205783894,-3.63428977912547,-16.1039041782365));
#27910=CARTESIAN_POINT('Ctrl Pts',(156.377899610377,4.41991580743947,-15.9062294789062));
#27911=CARTESIAN_POINT('Ctrl Pts',(156.49559343686,11.4214698111898,-11.9203112095514));
#27912=CARTESIAN_POINT('Ctrl Pts',(156.613287263343,15.702875106546,-5.0954396639247));
#27913=CARTESIAN_POINT('Ctrl Pts',(156.730981089826,16.2444679132066,2.94296690387111));
#27914=CARTESIAN_POINT('Ctrl Pts',(156.84867491631,12.9172619450047,10.2804735214198));
#27915=CARTESIAN_POINT('Ctrl Pts',(156.966368742793,6.5136679132218,15.1695722516076));
#27916=CARTESIAN_POINT('Ctrl Pts',(157.084062569276,-1.44122780336697,16.4458704360481));
#27917=CARTESIAN_POINT('Ctrl Pts',(157.201756395759,-9.0528792604481,13.8054036187367));
#27918=CARTESIAN_POINT('Ctrl Pts',(157.319450222242,-14.5084879108993,7.87702802583353));
#27919=CARTESIAN_POINT('Ctrl Pts',(157.437144048726,-16.5087405253944,0.0726515359649123));
#27920=CARTESIAN_POINT('Ctrl Pts',(157.554837875209,-14.5772549345868,-7.74902771659407));
#27921=CARTESIAN_POINT('Ctrl Pts',(157.672531701692,-9.17403568447366,-13.7251907542476));
#27922=CARTESIAN_POINT('Ctrl Pts',(157.790225528175,-1.58591889223899,-16.4325485925865));
#27923=CARTESIAN_POINT('Ctrl Pts',(157.907919354658,6.37990193438496,-15.226314172777));
#27924=CARTESIAN_POINT('Ctrl Pts',(158.025613181142,12.8262789159184,-10.3937654943502));
#27925=CARTESIAN_POINT('Ctrl Pts',(158.143307007625,16.2179364433534,-3.08582719863357));
#27926=CARTESIAN_POINT('Ctrl Pts',(158.261000834108,15.7471139574029,4.95703479845001));
#27927=CARTESIAN_POINT('Ctrl Pts',(158.378694660591,11.5259430136559,11.8193244149755));
#27928=CARTESIAN_POINT('Ctrl Pts',(158.496388487074,4.55974191880648,15.8667118715365));
#27929=CARTESIAN_POINT('Ctrl Pts',(158.614082313558,-3.492411885816,16.1352673110888));
#27930=CARTESIAN_POINT('Ctrl Pts',(158.731776140041,-10.7128093720813,12.5610313007303));
#27931=CARTESIAN_POINT('Ctrl Pts',(158.849469966524,-15.3818334310674,5.99524747440632));
#27932=CARTESIAN_POINT('Ctrl Pts',(158.967163793007,-16.387504608863,-1.99837050492948));
#27933=CARTESIAN_POINT('Ctrl Pts',(159.08485761949,-13.4903112488624,-9.51605456002099));
#27934=CARTESIAN_POINT('Ctrl Pts',(159.202551445973,-7.3802518281838,-14.7673855144731));
#27935=CARTESIAN_POINT('Ctrl Pts',(159.320245272457,0.487495771855852,-16.5017011199725));
#27936=CARTESIAN_POINT('Ctrl Pts',(159.43793909894,8.23914088980841,-14.3059550320265));
#27937=CARTESIAN_POINT('Ctrl Pts',(159.555632925423,14.0285439478352,-8.70308834174033));
#27938=CARTESIAN_POINT('Ctrl Pts',(159.673326751906,16.4768949056349,-1.02748540093825));
#27939=CARTESIAN_POINT('Ctrl Pts',(159.791020578389,15.0010920428818,6.89282449373751));
#27940=CARTESIAN_POINT('Ctrl Pts',(159.908714404872,9.95261404991291,13.1715323920171));
#27941=CARTESIAN_POINT('Ctrl Pts',(160.026408231356,2.53381151022997,16.3132949219679));
#27942=CARTESIAN_POINT('Ctrl Pts',(160.144102057839,-5.4884461206807,15.5698667676016));
#27943=CARTESIAN_POINT('Ctrl Pts',(160.261795884322,-12.2035699174123,11.1183035239783));
#27944=CARTESIAN_POINT('Ctrl Pts',(160.379489710805,-16.0122792598392,4.01879395906327));
#27945=CARTESIAN_POINT('Ctrl Pts',(160.497183537288,-16.007488110024,-4.03783560684653));
#27946=CARTESIAN_POINT('Ctrl Pts',(160.614877363772,-12.1903375330135,-11.1328101938226));
#27947=CARTESIAN_POINT('Ctrl Pts',(160.732571190255,-5.4699239396416,-15.5763835364636));
#27948=CARTESIAN_POINT('Ctrl Pts',(160.850265016738,2.55321222669146,-16.3102697496379));
#27949=CARTESIAN_POINT('Ctrl Pts',(160.967958843221,9.96827280770127,-13.1596857565719));
#27950=CARTESIAN_POINT('Ctrl Pts',(161.085652669704,15.0092795365331,-6.8749778017596));
#27951=CARTESIAN_POINT('Ctrl Pts',(161.203346496188,16.4756611934474,1.04708176338345));
#27952=CARTESIAN_POINT('Ctrl Pts',(161.321040322671,14.0181828519411,8.71976728531359));
#27953=CARTESIAN_POINT('Ctrl Pts',(161.438734149154,8.22212001920016,14.3157442827939));
#27954=CARTESIAN_POINT('Ctrl Pts',(161.556427975637,0.467868834153206,16.5022692601504));
#27955=CARTESIAN_POINT('Ctrl Pts',(161.67412180212,-7.39781046180786,14.7585972352269));
#27956=CARTESIAN_POINT('Ctrl Pts',(161.791815628604,-13.5016197966082,9.50000288675245));
#27957=CARTESIAN_POINT('Ctrl Pts',(161.909509455087,-16.3898698156561,1.97887832024774));
#27958=CARTESIAN_POINT('Ctrl Pts',(162.02720328157,-15.3746919968823,-6.01353789224345));
#27959=CARTESIAN_POINT('Ctrl Pts',(162.144897108053,-10.6978621080534,-12.5737638874599));
#27960=CARTESIAN_POINT('Ctrl Pts',(162.262590934536,-3.47321864733025,-16.1394096610853));
#27961=CARTESIAN_POINT('Ctrl Pts',(162.380284761019,4.57861005079439,-15.861277438562));
#27962=CARTESIAN_POINT('Ctrl Pts',(162.497978587503,11.5399923859502,-11.8056074690535));
#27963=CARTESIAN_POINT('Ctrl Pts',(162.615672413986,15.7529985573068,-4.93830218115272));
#27964=CARTESIAN_POINT('Ctrl Pts',(162.733366240469,16.2142547888485,3.10511410831708));
#27965=CARTESIAN_POINT('Ctrl Pts',(162.851060066952,12.8139078331282,10.4090133067854));
#27966=CARTESIAN_POINT('Ctrl Pts',(162.968753893435,6.36178773363243,15.233891453402));
#27967=CARTESIAN_POINT('Ctrl Pts',(163.086447719919,-1.60546211644266,16.4306507291704));
#27968=CARTESIAN_POINT('Ctrl Pts',(163.204141546402,-9.19035349473336,13.7142697427697));
#27969=CARTESIAN_POINT('Ctrl Pts',(163.321835372885,-14.5864610720469,7.73168451831101));
#27970=CARTESIAN_POINT('Ctrl Pts',(163.439529199368,-16.5086424323394,-0.0922864520782876));
#27971=CARTESIAN_POINT('Ctrl Pts',(163.557223025851,-14.4991089795936,-7.89427837917087));
#27972=CARTESIAN_POINT('Ctrl Pts',(163.674916852335,-9.03645312437413,-13.8161610668922));
#27973=CARTESIAN_POINT('Ctrl Pts',(163.792610678818,-1.42166665518031,-16.4475729352965));
#27974=CARTESIAN_POINT('Ctrl Pts',(163.910304505301,6.5317056326209,-15.1618144131892));
#27975=CARTESIAN_POINT('Ctrl Pts',(164.027998331784,12.929479817265,-10.2651027954568));
#27976=CARTESIAN_POINT('Ctrl Pts',(164.145692158267,16.2479572192145,-2.92364433524647));
#27977=CARTESIAN_POINT('Ctrl Pts',(164.263385984751,15.6968025698744,5.1141128849533));
#27978=CARTESIAN_POINT('Ctrl Pts',(164.381079811234,11.4072863090007,11.9338864302274));
#27979=CARTESIAN_POINT('Ctrl Pts',(164.498773637717,4.40098978716235,15.9114765234129));
#27980=CARTESIAN_POINT('Ctrl Pts',(164.6164674642,-3.65343136949515,16.0995674308211));
#27981=CARTESIAN_POINT('Ctrl Pts',(164.734161290683,-10.8377876645193,12.4533814633825));
#27982=CARTESIAN_POINT('Ctrl Pts',(164.851855117167,-15.4409234832775,5.8412605319531));
#27983=CARTESIAN_POINT('Ctrl Pts',(164.96954894365,-16.3668018890651,-2.16196928388703));
#27984=CARTESIAN_POINT('Ctrl Pts',(165.087242770133,-13.3944008250271,-9.65040813125861));
#27985=CARTESIAN_POINT('Ctrl Pts',(165.204936596616,-7.23268723116105,-14.8402762372271));
#27986=CARTESIAN_POINT('Ctrl Pts',(165.322630423099,0.6530358372013,-16.4962133373671));
#27987=CARTESIAN_POINT('Ctrl Pts',(165.401092974088,5.80398048830776,-14.9798339628417));
#27988=CARTESIAN_POINT('Ctrl Pts',(165.440324249582,8.04829710023833,-13.6572445638311));
#27989=CARTESIAN_POINT('Ctrl Pts',(149.834675750418,-6.94218356525857,14.5692179326398));
#27990=CARTESIAN_POINT('Ctrl Pts',(149.873907025912,-9.33636620409445,13.4283979212707));
#27991=CARTESIAN_POINT('Ctrl Pts',(149.952369576901,-13.5492960147677,9.9450267124702));
#27992=CARTESIAN_POINT('Ctrl Pts',(150.070063403384,-16.642450412093,2.34726636911127));
#27993=CARTESIAN_POINT('Ctrl Pts',(150.187757229867,-15.7715623732181,-5.80803173104413));
#27994=CARTESIAN_POINT('Ctrl Pts',(150.30545105635,-11.1447227959129,-12.5808087266611));
#27995=CARTESIAN_POINT('Ctrl Pts',(150.423144882834,-3.86353739057469,-16.3569758645323));
#27996=CARTESIAN_POINT('Ctrl Pts',(150.540838709317,4.33773958218958,-16.2377207209922));
#27997=CARTESIAN_POINT('Ctrl Pts',(150.6585325358,11.5059616765565,-12.2511901249246));
#27998=CARTESIAN_POINT('Ctrl Pts',(150.776226362283,15.9338999488442,-5.34694454897571));
#27999=CARTESIAN_POINT('Ctrl Pts',(150.893920188766,16.5670106914817,2.83075456988176));
#28000=CARTESIAN_POINT('Ctrl Pts',(151.011614015249,13.2545025899662,10.3342686568263));
#28001=CARTESIAN_POINT('Ctrl Pts',(151.129307841733,6.78529029631758,15.3765676735605));
#28002=CARTESIAN_POINT('Ctrl Pts',(151.247001668216,-1.29991424422042,16.7567656060342));
#28003=CARTESIAN_POINT('Ctrl Pts',(151.364695494699,-9.07552956165211,14.1461565529374));
#28004=CARTESIAN_POINT('Ctrl Pts',(151.482389321182,-14.6897078210113,8.16648411676187));
#28005=CARTESIAN_POINT('Ctrl Pts',(151.600083147665,-16.8053704474042,0.241873897185706));
#28006=CARTESIAN_POINT('Ctrl Pts',(151.717776974149,-14.9186492283738,-7.74034138233968));
#28007=CARTESIAN_POINT('Ctrl Pts',(151.835470800632,-9.47888752319158,-13.8791091296951));
#28008=CARTESIAN_POINT('Ctrl Pts',(151.953164627115,-1.78162446557883,-16.7124143539056));
#28009=CARTESIAN_POINT('Ctrl Pts',(152.070858453598,6.33995206670156,-15.5654741944342));
#28010=CARTESIAN_POINT('Ctrl Pts',(152.188552280081,12.951599252216,-10.7114450926761));
#28011=CARTESIAN_POINT('Ctrl Pts',(152.306246106565,16.478680567709,-3.30636747821358));
#28012=CARTESIAN_POINT('Ctrl Pts',(152.423939933048,16.0811827870456,4.88615793010572));
#28013=CARTESIAN_POINT('Ctrl Pts',(152.541633759531,11.8537743812354,11.9149910647864));
#28014=CARTESIAN_POINT('Ctrl Pts',(152.659327586014,4.80325917680914,16.1061379737952));
#28015=CARTESIAN_POINT('Ctrl Pts',(152.777021412497,-3.39120505179396,16.4614309052881));
#28016=CARTESIAN_POINT('Ctrl Pts',(152.89471523898,-10.7780164831926,12.8962529379659));
#28017=CARTESIAN_POINT('Ctrl Pts',(153.012409065464,-15.5979246962986,6.25969043330361));
#28018=CARTESIAN_POINT('Ctrl Pts',(153.130102891947,-16.7030155157083,-1.86768622477728));
#28019=CARTESIAN_POINT('Ctrl Pts',(153.24779671843,-13.8300994032196,-9.55025285786763));
#28020=CARTESIAN_POINT('Ctrl Pts',(153.365490544913,-7.66339294233319,-14.9583216894008));
#28021=CARTESIAN_POINT('Ctrl Pts',(153.483184371396,0.328434869711692,-16.8039016210083));
#28022=CARTESIAN_POINT('Ctrl Pts',(153.60087819788,8.24204230369565,-14.6474474846737));
#28023=CARTESIAN_POINT('Ctrl Pts',(153.718572024363,14.1927166741118,-9.00254256088617));
#28024=CARTESIAN_POINT('Ctrl Pts',(153.836265850846,16.7632394031106,-1.21358306933514));
#28025=CARTESIAN_POINT('Ctrl Pts',(153.953959677329,15.3414122187735,6.86440458349061));
#28026=CARTESIAN_POINT('Ctrl Pts',(154.071653503812,10.2658589097167,13.3075587542557));
#28027=CARTESIAN_POINT('Ctrl Pts',(154.189347330296,2.74537834388392,16.5813713817981));
#28028=CARTESIAN_POINT('Ctrl Pts',(154.307041156779,-5.42894428252613,15.9061479664124));
#28029=CARTESIAN_POINT('Ctrl Pts',(154.424734983262,-12.310304092225,11.4427003940996));
#28030=CARTESIAN_POINT('Ctrl Pts',(154.542428809745,-16.2598295294687,4.25404781646794));
#28031=CARTESIAN_POINT('Ctrl Pts',(154.660122636228,-16.33689765391,-3.94775305684763));
#28032=CARTESIAN_POINT('Ctrl Pts',(154.777816462712,-12.5231538437161,-11.2093531017091));
#28033=CARTESIAN_POINT('Ctrl Pts',(154.895510289195,-5.72688315071847,-15.8013223665045));
#28034=CARTESIAN_POINT('Ctrl Pts',(155.013204115678,2.4333077787351,-16.6300328444091));
#28035=CARTESIAN_POINT('Ctrl Pts',(155.130897942161,10.0139796864803,-13.4981180166325));
#28036=CARTESIAN_POINT('Ctrl Pts',(155.248591768644,15.2097121459439,-7.15147786053393));
#28037=CARTESIAN_POINT('Ctrl Pts',(155.366285595127,16.7830843021561,0.898365437281314));
#28038=CARTESIAN_POINT('Ctrl Pts',(155.483979421611,14.3593802639669,8.7342531213022));
#28039=CARTESIAN_POINT('Ctrl Pts',(155.601673248094,8.51583181660166,14.4899823196419));
#28040=CARTESIAN_POINT('Ctrl Pts',(155.719367074577,0.64414432060565,16.7947627922043));
#28041=CARTESIAN_POINT('Ctrl Pts',(155.83706090106,-7.38095323299944,15.0996857094594));
#28042=CARTESIAN_POINT('Ctrl Pts',(155.954754727543,-13.6481955599689,9.80845232995632));
#28043=CARTESIAN_POINT('Ctrl Pts',(156.072448554027,-16.6649699403357,2.18122810358885));
#28044=CARTESIAN_POINT('Ctrl Pts',(156.19014238051,-15.7127983612061,-5.96547959616457));
#28045=CARTESIAN_POINT('Ctrl Pts',(156.307836206993,-11.0184509610961,-12.6914426906518));
#28046=CARTESIAN_POINT('Ctrl Pts',(156.425530033476,-3.69993822624373,-16.3947990617195));
#28047=CARTESIAN_POINT('Ctrl Pts',(156.543223859959,4.49975550839517,-16.1935536407808));
#28048=CARTESIAN_POINT('Ctrl Pts',(156.660917686443,11.6277829569437,-12.1356352391784));
#28049=CARTESIAN_POINT('Ctrl Pts',(156.778611512926,15.9865259513294,-5.18748177439226));
#28050=CARTESIAN_POINT('Ctrl Pts',(156.896305339409,16.5379018872638,2.99612755392965));
#28051=CARTESIAN_POINT('Ctrl Pts',(157.013999165892,13.1505945186976,10.4661761382551));
#28052=CARTESIAN_POINT('Ctrl Pts',(157.131692992375,6.63132836671759,15.443589713695));
#28053=CARTESIAN_POINT('Ctrl Pts',(157.249386818858,-1.4672616017113,16.7429424697191));
#28054=CARTESIAN_POINT('Ctrl Pts',(157.367080645342,-9.21640707510144,14.0547792504258));
#28055=CARTESIAN_POINT('Ctrl Pts',(157.484774471825,-14.7705637934707,8.01931570492096));
#28056=CARTESIAN_POINT('Ctrl Pts',(157.602468298308,-16.8069482207728,0.0739638860544137));
#28057=CARTESIAN_POINT('Ctrl Pts',(157.720162124791,-14.8405729988752,-7.88900324611639));
#28058=CARTESIAN_POINT('Ctrl Pts',(157.837855951274,-9.33975202331718,-13.9731174508455));
#28059=CARTESIAN_POINT('Ctrl Pts',(157.955549777758,-1.61456633612997,-16.7293799854751));
#28060=CARTESIAN_POINT('Ctrl Pts',(158.073243604241,6.49514608942308,-15.5013565996409));
#28061=CARTESIAN_POINT('Ctrl Pts',(158.190937430724,13.0579680063074,-10.5815145748816));
#28062=CARTESIAN_POINT('Ctrl Pts',(158.308631257207,16.5108911628928,-3.14156842346082));
#28063=CARTESIAN_POINT('Ctrl Pts',(158.42632508369,16.0315639161914,5.04657681535204));
#28064=CARTESIAN_POINT('Ctrl Pts',(158.544018910174,11.7341433241446,12.0328242570317));
#28065=CARTESIAN_POINT('Ctrl Pts',(158.661712736657,4.64210738618032,16.1533222021771));
#28066=CARTESIAN_POINT('Ctrl Pts',(158.77940656314,-3.55549750389685,16.4267287264374));
#28067=CARTESIAN_POINT('Ctrl Pts',(158.897100389623,-10.9063215415264,12.7879290577097));
#28068=CARTESIAN_POINT('Ctrl Pts',(159.014794216106,-15.659685099468,6.10354337558762));
#28069=CARTESIAN_POINT('Ctrl Pts',(159.13248804259,-16.6835223441284,-2.03446832001538));
#28070=CARTESIAN_POINT('Ctrl Pts',(159.250181869073,-13.7339951701931,-9.68794899951949));
#28071=CARTESIAN_POINT('Ctrl Pts',(159.367875695556,-7.51356592840906,-15.0341380262265));
#28072=CARTESIAN_POINT('Ctrl Pts',(159.485569522039,0.496301712588155,-16.7997816581723));
#28073=CARTESIAN_POINT('Ctrl Pts',(159.603263348522,8.38796963981923,-14.5643724366568));
#28074=CARTESIAN_POINT('Ctrl Pts',(159.720957175005,14.281950302715,-8.86029766446685));
#28075=CARTESIAN_POINT('Ctrl Pts',(159.838651001489,16.7745273536853,-1.04604551174608));
#28076=CARTESIAN_POINT('Ctrl Pts',(159.956344827972,15.2720661416863,7.01733388945811));
#28077=CARTESIAN_POINT('Ctrl Pts',(160.074038654455,10.1323943362558,13.4094580116719));
#28078=CARTESIAN_POINT('Ctrl Pts',(160.191732480938,2.57958133075788,16.60797216129));
#28079=CARTESIAN_POINT('Ctrl Pts',(160.309426307421,-5.58758735234152,15.8511149996501));
#28080=CARTESIAN_POINT('Ctrl Pts',(160.427120133904,-12.4240106260698,11.3191403876568));
#28081=CARTESIAN_POINT('Ctrl Pts',(160.544813960388,-16.3015190651706,4.0913879454361));
#28082=CARTESIAN_POINT('Ctrl Pts',(160.662507786871,-16.2966413698226,-4.11077355440117));
#28083=CARTESIAN_POINT('Ctrl Pts',(160.780201613354,-12.4105392168435,-11.3339091005428));
#28084=CARTESIAN_POINT('Ctrl Pts',(160.897895439837,-5.56873059357299,-15.85774948498));
#28085=CARTESIAN_POINT('Ctrl Pts',(161.015589266321,2.59933249448306,-16.6048923433819));
#28086=CARTESIAN_POINT('Ctrl Pts',(161.133283092804,10.1483359479702,-13.3973973830485));
#28087=CARTESIAN_POINT('Ctrl Pts',(161.250976919287,15.2804015311513,-6.99916482153175));
#28088=CARTESIAN_POINT('Ctrl Pts',(161.36867074577,16.7732713561836,1.06599585553062));
#28089=CARTESIAN_POINT('Ctrl Pts',(161.486364572253,14.2714020478718,8.87727789021946));
#28090=CARTESIAN_POINT('Ctrl Pts',(161.604058398736,8.37064131058994,14.5743385167775));
#28091=CARTESIAN_POINT('Ctrl Pts',(161.72175222522,0.476320241246173,16.8003600610212));
#28092=CARTESIAN_POINT('Ctrl Pts',(161.839446051703,-7.53144173460349,15.0251909988012));
#28093=CARTESIAN_POINT('Ctrl Pts',(161.957139878186,-13.745507991303,9.67160737484704));
#28094=CARTESIAN_POINT('Ctrl Pts',(162.074833704669,-16.6859302751296,2.01462403582233));
#28095=CARTESIAN_POINT('Ctrl Pts',(162.192527531152,-15.652414665095,-6.12216418467065));
#28096=CARTESIAN_POINT('Ctrl Pts',(162.310221357636,-10.8911042757288,-12.8008916411092));
#28097=CARTESIAN_POINT('Ctrl Pts',(162.427915184119,-3.53595756595174,-16.4309459022901));
#28098=CARTESIAN_POINT('Ctrl Pts',(162.545609010602,4.66131634502582,-16.1477896036442));
#28099=CARTESIAN_POINT('Ctrl Pts',(162.663302837085,11.7484464790292,-12.0188595333448));
#28100=CARTESIAN_POINT('Ctrl Pts',(162.780996663568,16.0375548133002,-5.02750581908371));
#28101=CARTESIAN_POINT('Ctrl Pts',(162.898690490052,16.5071430043621,3.16120372464508));
#28102=CARTESIAN_POINT('Ctrl Pts',(163.016384316535,13.0453734569189,10.5970378180802));
#28103=CARTESIAN_POINT('Ctrl Pts',(163.134078143018,6.47670468054396,15.5090707534204));
#28104=CARTESIAN_POINT('Ctrl Pts',(163.251771969501,-1.63446258180371,16.7274478397662));
#28105=CARTESIAN_POINT('Ctrl Pts',(163.369465795984,-9.35636459237956,13.9619991663135));
#28106=CARTESIAN_POINT('Ctrl Pts',(163.487159622468,-14.8499454325485,7.87134676680609));
#28107=CARTESIAN_POINT('Ctrl Pts',(163.604853448951,-16.8068483558016,-0.0939534799261245));
#28108=CARTESIAN_POINT('Ctrl Pts',(163.722547275434,-14.7610154446685,-8.03687766216926));
#28109=CARTESIAN_POINT('Ctrl Pts',(163.840241101917,-9.19968422346793,-14.065731017089));
#28110=CARTESIAN_POINT('Ctrl Pts',(163.9579349284,-1.44734710828245,-16.7446757222752));
#28111=CARTESIAN_POINT('Ctrl Pts',(164.075628754883,6.64969191271279,-15.4356917405938));
#28112=CARTESIAN_POINT('Ctrl Pts',(164.193322581367,13.1630330900188,-10.4505277612649));
#28113=CARTESIAN_POINT('Ctrl Pts',(164.31101640785,16.5414542227863,-2.97645594967455));
#28114=CARTESIAN_POINT('Ctrl Pts',(164.428710234333,15.9803437226336,5.20649230148));
#28115=CARTESIAN_POINT('Ctrl Pts',(164.546404060816,11.6133432492922,12.1494556775476));
#28116=CARTESIAN_POINT('Ctrl Pts',(164.664097887299,4.48048761558814,16.198895465931));
#28117=CARTESIAN_POINT('Ctrl Pts',(164.781791713783,-3.7194255831206,16.3903839769258));
#28118=CARTESIAN_POINT('Ctrl Pts',(164.899485540266,-11.0335573949518,12.6783346740863));
#28119=CARTESIAN_POINT('Ctrl Pts',(165.017179366749,-15.7198425322127,5.94677487077617));
#28120=CARTESIAN_POINT('Ctrl Pts',(165.134873193232,-16.662445658167,-2.20102228593978));
#28121=CARTESIAN_POINT('Ctrl Pts',(165.252567019715,-13.6363522564438,-9.82472948326341));
#28122=CARTESIAN_POINT('Ctrl Pts',(165.370260846199,-7.3633357798665,-15.1083454196505));
#28123=CARTESIAN_POINT('Ctrl Pts',(165.487954672682,0.664832031569472,-16.7941947463207));
#28124=CARTESIAN_POINT('Ctrl Pts',(165.56641722367,5.90882141440849,-15.2504240636636));
#28125=CARTESIAN_POINT('Ctrl Pts',(165.605648499165,8.19367851963193,-13.9039439059363));
#28126=CARTESIAN_POINT('Ctrl Pts',(150.,-7.06535955977555,14.8277213114857));
#28127=CARTESIAN_POINT('Ctrl Pts',(150.039231275494,-9.50202246794194,13.6666595940101));
#28128=CARTESIAN_POINT('Ctrl Pts',(150.117693826483,-13.7897027968609,10.1214825126218));
#28129=CARTESIAN_POINT('Ctrl Pts',(150.235387652966,-16.9377394031488,2.38891419744853));
#28130=CARTESIAN_POINT('Ctrl Pts',(150.35308147945,-16.0513990934872,-5.91108433372057));
#28131=CARTESIAN_POINT('Ctrl Pts',(150.470775305933,-11.3424649473698,-12.8040315227983));
#28132=CARTESIAN_POINT('Ctrl Pts',(150.588469132416,-3.9320885972612,-16.6471996464972));
#28133=CARTESIAN_POINT('Ctrl Pts',(150.706162958899,4.41470461516072,-16.5258285446613));
#28134=CARTESIAN_POINT('Ctrl Pts',(150.823856785382,11.710113332741,-12.4685644587302));
#28135=CARTESIAN_POINT('Ctrl Pts',(150.941550611866,16.2166170441621,-5.44181602655281));
#28136=CARTESIAN_POINT('Ctrl Pts',(151.059244438349,16.8609611465387,2.88098098727637));
#28137=CARTESIAN_POINT('Ctrl Pts',(151.176938264832,13.4896788170136,10.517630823419));
#28138=CARTESIAN_POINT('Ctrl Pts',(151.294632091315,6.90568251477146,15.6493959555621));
#28139=CARTESIAN_POINT('Ctrl Pts',(151.412325917798,-1.32297877835631,17.0540829052685));
#28140=CARTESIAN_POINT('Ctrl Pts',(151.530019744282,-9.23655776971034,14.39715350305));
#28141=CARTESIAN_POINT('Ctrl Pts',(151.647713570765,-14.9503490663786,8.31138302260808));
#28142=CARTESIAN_POINT('Ctrl Pts',(151.765407397248,-17.1035501481607,0.246165494714576));
#28143=CARTESIAN_POINT('Ctrl Pts',(151.883101223731,-15.183352608554,-7.87767918660661));
#28144=CARTESIAN_POINT('Ctrl Pts',(152.000795050214,-9.64707255987471,-14.1253678253907));
#28145=CARTESIAN_POINT('Ctrl Pts',(152.118488876697,-1.81323604187045,-17.0089447235611));
#28146=CARTESIAN_POINT('Ctrl Pts',(152.236182703181,6.45244259560576,-15.8416542674624));
#28147=CARTESIAN_POINT('Ctrl Pts',(152.353876529664,13.1814010290606,-10.9014995459474));
#28148=CARTESIAN_POINT('Ctrl Pts',(152.471570356147,16.7710637708,-3.36503275240856));
#28149=CARTESIAN_POINT('Ctrl Pts',(152.58926418263,16.3665131394028,4.97285361551223));
#28150=CARTESIAN_POINT('Ctrl Pts',(152.706958009113,12.0640973198993,12.1264001783988));
#28151=CARTESIAN_POINT('Ctrl Pts',(152.824651835597,4.8884839797065,16.39191110902));
#28152=CARTESIAN_POINT('Ctrl Pts',(152.94234566208,-3.45137560921858,16.7535080455525));
#28153=CARTESIAN_POINT('Ctrl Pts',(153.060039488563,-10.9692521206197,13.1250726985274));
#28154=CARTESIAN_POINT('Ctrl Pts',(153.177733315046,-15.8746805424682,6.37075687043291));
#28155=CARTESIAN_POINT('Ctrl Pts',(153.295427141529,-16.9993791206519,-1.90082480517061));
#28156=CARTESIAN_POINT('Ctrl Pts',(153.413120968012,-14.0754885134681,-9.71970413823186));
#28157=CARTESIAN_POINT('Ctrl Pts',(153.530814794496,-7.79936544121243,-15.2237289828089));
#28158=CARTESIAN_POINT('Ctrl Pts',(153.648508620979,0.33426232894414,-17.1020552602022));
#28159=CARTESIAN_POINT('Ctrl Pts',(153.766202447462,8.38828184750279,-14.9073388998315));
#28160=CARTESIAN_POINT('Ctrl Pts',(153.883896273945,14.4445397460312,-9.16227575184762));
#28161=CARTESIAN_POINT('Ctrl Pts',(154.001590100428,17.0606715677019,-1.23511581909452));
#28162=CARTESIAN_POINT('Ctrl Pts',(154.119283926912,15.6136167333299,6.9862005362179));
#28163=CARTESIAN_POINT('Ctrl Pts',(154.236977753395,10.4480072739726,13.5436763631809));
#28164=CARTESIAN_POINT('Ctrl Pts',(154.354671579878,2.79408992067451,16.8755766403035));
#28165=CARTESIAN_POINT('Ctrl Pts',(154.472365406361,-5.52527069119732,16.1883726549819));
#28166=CARTESIAN_POINT('Ctrl Pts',(154.590059232844,-12.528727292233,11.6457295977722));
#28167=CARTESIAN_POINT('Ctrl Pts',(154.707753059327,-16.5483296323747,4.3295278964155));
#28168=CARTESIAN_POINT('Ctrl Pts',(154.825446885811,-16.6267651857789,-4.01779851218795));
#28169=CARTESIAN_POINT('Ctrl Pts',(154.943140712294,-12.7453536623595,-11.408241996423));
#28170=CARTESIAN_POINT('Ctrl Pts',(155.060834538777,-5.82849592441443,-16.0816871218991));
#28171=CARTESIAN_POINT('Ctrl Pts',(155.17852836526,2.47648225010914,-16.9251015090742));
#28172=CARTESIAN_POINT('Ctrl Pts',(155.296222191744,10.1916589275088,-13.7376167413748));
#28173=CARTESIAN_POINT('Ctrl Pts',(155.413916018227,15.4795798903333,-7.2783673888008));
#28174=CARTESIAN_POINT('Ctrl Pts',(155.53160984471,17.0808685771681,0.91430524283911));
#28175=CARTESIAN_POINT('Ctrl Pts',(155.649303671193,14.6141604679237,8.88922602060199));
#28176=CARTESIAN_POINT('Ctrl Pts',(155.766997497676,8.66692924053017,14.7470798115157));
#28177=CARTESIAN_POINT('Ctrl Pts',(155.884691324159,0.655573450440289,17.0927542800641));
#28178=CARTESIAN_POINT('Ctrl Pts',(156.002385150643,-7.51191437028597,15.3676012416077));
#28179=CARTESIAN_POINT('Ctrl Pts',(156.120078977126,-13.8903571285385,9.98248487448037));
#28180=CARTESIAN_POINT('Ctrl Pts',(156.237772803609,-16.9606584980785,2.21992989509328));
#28181=CARTESIAN_POINT('Ctrl Pts',(156.355466630092,-15.9915924245715,-6.07132581517059));
#28182=CARTESIAN_POINT('Ctrl Pts',(156.473160456575,-11.2139526562633,-12.9166284784635));
#28183=CARTESIAN_POINT('Ctrl Pts',(156.590854283059,-3.76558667336199,-16.6856939452026));
#28184=CARTESIAN_POINT('Ctrl Pts',(156.708548109542,4.57959520935088,-16.4808778026554));
#28185=CARTESIAN_POINT('Ctrl Pts',(156.826241936025,11.8340961026976,-12.3509592688053));
#28186=CARTESIAN_POINT('Ctrl Pts',(156.943935762508,16.2701767961127,-5.27952388485984));
#28187=CARTESIAN_POINT('Ctrl Pts',(157.061629588991,16.831335861321,3.04928820398821));
#28188=CARTESIAN_POINT('Ctrl Pts',(157.179323415474,13.3839270923905,10.6518787550904));
#28189=CARTESIAN_POINT('Ctrl Pts',(157.297017241958,6.74898882021338,15.7176071757824));
#28190=CARTESIAN_POINT('Ctrl Pts',(157.414711068441,-1.49329540005564,17.04001450339));
#28191=CARTESIAN_POINT('Ctrl Pts',(157.532404894924,-9.37993488975477,14.3041548821149));
#28192=CARTESIAN_POINT('Ctrl Pts',(157.650098721407,-15.032639676042,8.16160338400838));
#28193=CARTESIAN_POINT('Ctrl Pts',(157.76779254789,-17.1051559161512,0.0752762361439129));
#28194=CARTESIAN_POINT('Ctrl Pts',(157.885486374374,-15.1038910631636,-8.0289787756387));
#28195=CARTESIAN_POINT('Ctrl Pts',(158.003180200857,-9.50546836216071,-14.2210441474433));
#28196=CARTESIAN_POINT('Ctrl Pts',(158.12087402734,-1.64321378002094,-17.0262113783636));
#28197=CARTESIAN_POINT('Ctrl Pts',(158.238567853823,6.61039024446121,-15.7763990265048));
#28198=CARTESIAN_POINT('Ctrl Pts',(158.356261680306,13.2896570966964,-10.7692636554129));
#28199=CARTESIAN_POINT('Ctrl Pts',(158.47395550679,16.8038458824322,-3.19730964828806));
#28200=CARTESIAN_POINT('Ctrl Pts',(158.591649333273,16.3160138749799,5.13611883225406));
#28201=CARTESIAN_POINT('Ctrl Pts',(158.709343159756,11.9423436346333,12.246324099088));
#28202=CARTESIAN_POINT('Ctrl Pts',(158.827036986239,4.72447285355417,16.4399325328178));
#28203=CARTESIAN_POINT('Ctrl Pts',(158.944730812722,-3.61858312197772,16.7181901417859));
#28204=CARTESIAN_POINT('Ctrl Pts',(159.062424639206,-11.0998337109716,13.0148268146891));
#28205=CARTESIAN_POINT('Ctrl Pts',(159.180118465689,-15.9375367678685,6.21183927676893));
#28206=CARTESIAN_POINT('Ctrl Pts',(159.297812292172,-16.9795400793939,-2.07056613510129));
#28207=CARTESIAN_POINT('Ctrl Pts',(159.415506118655,-13.9776790915239,-9.85984343901797));
#28208=CARTESIAN_POINT('Ctrl Pts',(159.533199945138,-7.6468800286343,-15.30089053798));
#28209=CARTESIAN_POINT('Ctrl Pts',(159.650893771621,0.50510765332046,-17.097862196372));
#28210=CARTESIAN_POINT('Ctrl Pts',(159.768587598105,8.53679838983004,-14.8227898412871));
#28211=CARTESIAN_POINT('Ctrl Pts',(159.886281424588,14.5353566575949,-9.01750698719337));
#28212=CARTESIAN_POINT('Ctrl Pts',(160.003975251071,17.0721598017356,-1.06460562255391));
#28213=CARTESIAN_POINT('Ctrl Pts',(160.121669077554,15.5430402404909,7.1418432851787));
#28214=CARTESIAN_POINT('Ctrl Pts',(160.239362904038,10.3121746225986,13.6473836313267));
#28215=CARTESIAN_POINT('Ctrl Pts',(160.35705673052,2.62535115128579,16.9026494006121));
#28216=CARTESIAN_POINT('Ctrl Pts',(160.474750557004,-5.68672858400233,16.1323632316986));
#28217=CARTESIAN_POINT('Ctrl Pts',(160.592444383487,-12.6444513347273,11.5199772513354));
#28218=CARTESIAN_POINT('Ctrl Pts',(160.71013820997,-16.590758870502,4.16398193180893));
#28219=CARTESIAN_POINT('Ctrl Pts',(160.827832036453,-16.5857946296213,-4.1837115019558));
#28220=CARTESIAN_POINT('Ctrl Pts',(160.945525862937,-12.6307409006735,-11.535008007263));
#28221=CARTESIAN_POINT('Ctrl Pts',(161.06321968942,-5.66753724750438,-16.1391154334964));
#28222=CARTESIAN_POINT('Ctrl Pts',(161.180913515903,2.64545276227466,-16.899514937126));
#28223=CARTESIAN_POINT('Ctrl Pts',(161.298607342386,10.3283990882391,-13.6351090095251));
#28224=CARTESIAN_POINT('Ctrl Pts',(161.416301168869,15.5515235257695,-7.1233518413039));
#28225=CARTESIAN_POINT('Ctrl Pts',(161.533994995353,17.0708815189199,1.0849099476778));
#28226=CARTESIAN_POINT('Ctrl Pts',(161.651688821836,14.5246212438026,9.03478849512532));
#28227=CARTESIAN_POINT('Ctrl Pts',(161.769382648319,8.51916260197972,14.8329327507611));
#28228=CARTESIAN_POINT('Ctrl Pts',(161.887076474802,0.484771648339155,17.098450861892));
#28229=CARTESIAN_POINT('Ctrl Pts',(162.004770301285,-7.66507300739915,15.2917847623754));
#28230=CARTESIAN_POINT('Ctrl Pts',(162.122464127769,-13.9893961859976,9.84321186294161));
#28231=CARTESIAN_POINT('Ctrl Pts',(162.240157954252,-16.9819907346032,2.05036975139694));
#28232=CARTESIAN_POINT('Ctrl Pts',(162.357851780735,-15.9301373333076,-6.23079047709786));
#28233=CARTESIAN_POINT('Ctrl Pts',(162.475545607218,-11.0843464434042,-13.0280193947584));
#28234=CARTESIAN_POINT('Ctrl Pts',(162.593239433701,-3.59869648457321,-16.722482143495));
#28235=CARTESIAN_POINT('Ctrl Pts',(162.710933260184,4.74402263925723,-16.4343017687264));
#28236=CARTESIAN_POINT('Ctrl Pts',(162.828627086668,11.9569005721082,-12.232111597636));
#28237=CARTESIAN_POINT('Ctrl Pts',(162.946320913151,16.3221110692936,-5.11670945701468));
#28238=CARTESIAN_POINT('Ctrl Pts',(163.064014739634,16.8000312198758,3.21729334097308));
#28239=CARTESIAN_POINT('Ctrl Pts',(163.181708566117,13.2768390807095,10.785062329375));
#28240=CARTESIAN_POINT('Ctrl Pts',(163.2994023926,6.59162162745551,15.7842500534388));
#28241=CARTESIAN_POINT('Ctrl Pts',(163.417096219084,-1.66346304716478,17.0242449503621));
#28242=CARTESIAN_POINT('Ctrl Pts',(163.534790045567,-9.52237569002574,14.2097285898572));
#28243=CARTESIAN_POINT('Ctrl Pts',(163.65248387205,-15.1134297930502,8.01100901530118));
#28244=CARTESIAN_POINT('Ctrl Pts',(163.770177698533,-17.1050542792638,-0.0956205077739737));
#28245=CARTESIAN_POINT('Ctrl Pts',(163.887871525016,-15.0229219097434,-8.17947694516765));
#28246=CARTESIAN_POINT('Ctrl Pts',(164.0055653515,-9.36291532256174,-14.3153009672858));
#28247=CARTESIAN_POINT('Ctrl Pts',(164.123259177983,-1.47302756138459,-17.0417785092538));
#28248=CARTESIAN_POINT('Ctrl Pts',(164.240953004466,6.76767819280469,-15.7095690679985));
#28249=CARTESIAN_POINT('Ctrl Pts',(164.358646830949,13.3965863627725,-10.635952727073));
#28250=CARTESIAN_POINT('Ctrl Pts',(164.476340657432,16.8349512263582,-3.02926756410262));
#28251=CARTESIAN_POINT('Ctrl Pts',(164.594034483916,16.2638848753927,5.2988717180067));
#28252=CARTESIAN_POINT('Ctrl Pts',(164.711728310399,11.8194001895836,12.3650249248679));
#28253=CARTESIAN_POINT('Ctrl Pts',(164.829422136882,4.55998544401394,16.4863144084491));
#28254=CARTESIAN_POINT('Ctrl Pts',(164.947115963365,-3.78541979674606,16.6812005230305));
#28255=CARTESIAN_POINT('Ctrl Pts',(165.064809789848,-11.2293271253843,12.9032878847901));
#28256=CARTESIAN_POINT('Ctrl Pts',(165.182503616331,-15.998761581148,6.05228920959924));
#28257=CARTESIAN_POINT('Ctrl Pts',(165.300197442814,-16.9580894272689,-2.24007528799254));
#28258=CARTESIAN_POINT('Ctrl Pts',(165.417891269298,-13.8783036878605,-9.99905083526821));
#28259=CARTESIAN_POINT('Ctrl Pts',(165.535585095781,-7.49398432857193,-15.3764146020739));
#28260=CARTESIAN_POINT('Ctrl Pts',(165.653278922264,0.676628225937629,-17.0921761552743));
#28261=CARTESIAN_POINT('Ctrl Pts',(165.731741473253,6.01366234050923,-15.5210141644856));
#28262=CARTESIAN_POINT('Ctrl Pts',(165.770972748747,8.33905993902552,-14.1506432480414));
#28263=CARTESIAN_POINT('Ctrl Pts',(165.268843152848,-16.4247445391107,-0.000389063610209933));
#28264=CARTESIAN_POINT('Ctrl Pts',(165.270895435232,-16.4248785782203,-0.141592307580833));
#28265=CARTESIAN_POINT('Ctrl Pts',(165.272947717616,-16.4231982118296,-0.282792220533225));
#28266=CARTESIAN_POINT('Ctrl Pts',(165.275,-16.4196979759281,-0.423941685645475));
#28267=CARTESIAN_POINT('Ctrl Pts',(150.,-9.03713009573195,-12.6741506013615));
#28268=CARTESIAN_POINT('Ctrl Pts',(150.030832127889,-7.39916843321553,-13.8395576086113));
#28269=CARTESIAN_POINT('Ctrl Pts',(150.100895531273,-3.16192523972154,-15.7683197386922));
#28270=CARTESIAN_POINT('Ctrl Pts',(150.210190210152,4.18380951624729,-15.6615050736542));
#28271=CARTESIAN_POINT('Ctrl Pts',(150.327884036635,11.0976583641875,-11.8164414573133));
#28272=CARTESIAN_POINT('Ctrl Pts',(150.445577863118,15.3684657582085,-5.15720159382155));
#28273=CARTESIAN_POINT('Ctrl Pts',(150.563271689601,15.9791097813677,2.73030173509255));
#28274=CARTESIAN_POINT('Ctrl Pts',(150.680965516085,12.7841501358716,9.96754432364079));
#28275=CARTESIAN_POINT('Ctrl Pts',(150.798659342568,6.54450585940981,14.8309111095575));
#28276=CARTESIAN_POINT('Ctrl Pts',(150.916353169051,-1.25378517594862,16.1621310075655));
#28277=CARTESIAN_POINT('Ctrl Pts',(151.034046995534,-8.75347314553567,13.6441626527123));
#28278=CARTESIAN_POINT('Ctrl Pts',(151.151740822017,-14.1684253302768,7.87668630506945));
#28279=CARTESIAN_POINT('Ctrl Pts',(151.231348624873,-15.5486722830063,2.7067130916238));
#28280=CARTESIAN_POINT('Ctrl Pts',(151.271725152234,-15.5672190915335,0.0747297253538588));
#28281=CARTESIAN_POINT('Ctrl Pts',(151.272870404101,-15.5671986622434,7.50751021387757E-5));
#28282=CARTESIAN_POINT('Origin',(147.227129595899,0.,0.));
#28283=CARTESIAN_POINT('Ctrl Pts',(150.,9.03673727728059,-12.6742328676692));
#28284=CARTESIAN_POINT('Ctrl Pts',(150.039231275494,11.1195140215529,-11.1892115301467));
#28285=CARTESIAN_POINT('Ctrl Pts',(150.117693826483,14.5370057041716,-7.17421629738743));
#28286=CARTESIAN_POINT('Ctrl Pts',(150.235387652966,16.2010328735656,0.560984685021083));
#28287=CARTESIAN_POINT('Ctrl Pts',(150.35308147945,14.0064191663237,8.1610886176298));
#28288=CARTESIAN_POINT('Ctrl Pts',(150.470775305933,8.47610941309655,13.8182656780649));
#28289=CARTESIAN_POINT('Ctrl Pts',(150.588469132416,0.927077910240183,16.1841184068341));
#28290=CARTESIAN_POINT('Ctrl Pts',(150.706162958899,-6.84272643302437,14.6957170013813));
#28291=CARTESIAN_POINT('Ctrl Pts',(150.823856785382,-12.9828704069121,9.70728517421879));
#28292=CARTESIAN_POINT('Ctrl Pts',(150.914178997716,-15.3221047690584,4.10479808015603));
#28293=CARTESIAN_POINT('Ctrl Pts',(150.965269934555,-15.5660958690062,0.773696244953541));
#28294=CARTESIAN_POINT('Ctrl Pts',(150.977129595899,-15.5654260231298,0.000355229555255854));
#28295=CARTESIAN_POINT('Ctrl Pts',(149.504027251253,9.53545461596197,-13.3736954603778));
#28296=CARTESIAN_POINT('Ctrl Pts',(149.543258526747,11.7331751550021,-11.8067191133635));
#28297=CARTESIAN_POINT('Ctrl Pts',(149.621721077736,15.3392705675541,-7.57014526479843));
#28298=CARTESIAN_POINT('Ctrl Pts',(149.739414904219,17.0951316783309,0.591944176325289));
#28299=CARTESIAN_POINT('Ctrl Pts',(149.857108730702,14.7794021442229,8.61148086333111));
#28300=CARTESIAN_POINT('Ctrl Pts',(149.974802557185,8.94388695261846,14.5808648853565));
#28301=CARTESIAN_POINT('Ctrl Pts',(150.092496383669,0.978241268647,17.0772837399741));
#28302=CARTESIAN_POINT('Ctrl Pts',(150.210190210152,-7.2203612155008,15.5067407866328));
#28303=CARTESIAN_POINT('Ctrl Pts',(150.327884036635,-13.6993660157928,10.2430085530626));
#28304=CARTESIAN_POINT('Ctrl Pts',(150.445577863118,-16.9157108038983,2.53983419096766));
#28305=CARTESIAN_POINT('Ctrl Pts',(150.563271689601,-16.1033955003998,-5.76825062376693));
#28306=CARTESIAN_POINT('Ctrl Pts',(150.680965516084,-11.4558781196984,-12.7025528487927));
#28307=CARTESIAN_POINT('Ctrl Pts',(150.798659342568,-4.08001792255419,-16.6116073332124));
#28308=CARTESIAN_POINT('Ctrl Pts',(150.916353169051,4.26754373314548,-16.5644223179528));
#28309=CARTESIAN_POINT('Ctrl Pts',(151.034046995534,11.5987427473219,-12.5722390515179));
#28310=CARTESIAN_POINT('Ctrl Pts',(151.151740822017,16.1675736233743,-5.58583814191949));
#28311=CARTESIAN_POINT('Ctrl Pts',(151.2694346485,16.8859189113636,2.73089130155499));
#28312=CARTESIAN_POINT('Ctrl Pts',(151.387128474984,13.5826968280316,10.3972290703567));
#28313=CARTESIAN_POINT('Ctrl Pts',(151.504822301467,7.04460603362714,15.5873522661647));
#28314=CARTESIAN_POINT('Ctrl Pts',(151.62251612795,-1.17123519699634,17.0651760414828));
#28315=CARTESIAN_POINT('Ctrl Pts',(151.740209954433,-9.10813388004872,14.4787403548484));
#28316=CARTESIAN_POINT('Ctrl Pts',(151.857903780917,-14.8758302598876,8.44403334780864));
#28317=CARTESIAN_POINT('Ctrl Pts',(151.975597607399,-17.1006839818747,0.398286883712695));
#28318=CARTESIAN_POINT('Ctrl Pts',(152.093291433883,-15.2528216508935,-7.74231598233075));
#28319=CARTESIAN_POINT('Ctrl Pts',(152.210985260366,-9.77233201382398,-14.0390011077331));
#28320=CARTESIAN_POINT('Ctrl Pts',(152.328679086849,-1.96445398056304,-16.9921436447781));
#28321=CARTESIAN_POINT('Ctrl Pts',(152.446372913332,6.31128038344754,-15.8984202048656));
#28322=CARTESIAN_POINT('Ctrl Pts',(152.564066739816,13.0839138797936,-11.0183130593643));
#28323=CARTESIAN_POINT('Ctrl Pts',(152.681760566299,16.7404693205759,-3.51407342198624));
#28324=CARTESIAN_POINT('Ctrl Pts',(152.799454392782,16.4100977937248,4.82708146695919));
#28325=CARTESIAN_POINT('Ctrl Pts',(152.917148219265,12.1714809135036,12.0186137911331));
#28326=CARTESIAN_POINT('Ctrl Pts',(153.034842045748,5.03409192834135,16.3477809975931));
#28327=CARTESIAN_POINT('Ctrl Pts',(153.152535872231,-3.30222144073897,16.7835442813653));
#28328=CARTESIAN_POINT('Ctrl Pts',(153.270229698715,-10.8520744386629,13.2221218216275));
#28329=CARTESIAN_POINT('Ctrl Pts',(153.387923525198,-15.8173865013383,6.51170556425243));
#28330=CARTESIAN_POINT('Ctrl Pts',(153.505617351681,-17.0156139266551,-1.74954502292907));
#28331=CARTESIAN_POINT('Ctrl Pts',(153.623311178164,-14.1613856689232,-9.59412221228455));
#28332=CARTESIAN_POINT('Ctrl Pts',(153.741005004647,-7.93446759340149,-15.1537536306189));
#28333=CARTESIAN_POINT('Ctrl Pts',(153.858698831131,0.182131244121732,-17.1043518818501));
#28334=CARTESIAN_POINT('Ctrl Pts',(153.976392657614,8.25535352182861,-14.9813605296003));
#28335=CARTESIAN_POINT('Ctrl Pts',(154.094086484097,14.362472522903,-9.29039332413286));
#28336=CARTESIAN_POINT('Ctrl Pts',(154.21178031058,17.0490106593108,-1.38681672435119));
#28337=CARTESIAN_POINT('Ctrl Pts',(154.329474137064,15.6751393133167,6.84704553777379));
#28338=CARTESIAN_POINT('Ctrl Pts',(154.447167963546,10.5680610629674,13.4502085655809));
#28339=CARTESIAN_POINT('Ctrl Pts',(154.56486179003,2.9440827878509,16.850056427992));
#28340=CARTESIAN_POINT('Ctrl Pts',(154.682555616513,-5.38106119756087,16.2368779473254));
#28341=CARTESIAN_POINT('Ctrl Pts',(154.800249442996,-12.4246462498137,11.7567083256848));
#28342=CARTESIAN_POINT('Ctrl Pts',(154.917943269479,-16.5091650866505,4.47654925472243));
#28343=CARTESIAN_POINT('Ctrl Pts',(155.035637095962,-16.6618446042499,-3.86974927767475));
#28344=CARTESIAN_POINT('Ctrl Pts',(155.153330922446,-12.8463224955304,-11.2944244399201));
#28345=CARTESIAN_POINT('Ctrl Pts',(155.271024748929,-5.97130733368415,-16.0292081468463));
#28346=CARTESIAN_POINT('Ctrl Pts',(155.388718575412,2.32584037324249,-16.9464595608177));
#28347=CARTESIAN_POINT('Ctrl Pts',(155.506412401895,10.0690636035655,-13.8277251648847));
#28348=CARTESIAN_POINT('Ctrl Pts',(155.624106228379,15.414228544653,-7.41576587153617));
#28349=CARTESIAN_POINT('Ctrl Pts',(155.741800054862,17.0883253517992,0.762339661366479));
#28350=CARTESIAN_POINT('Ctrl Pts',(155.859493881345,14.6926494499394,8.75888561572939));
#28351=CARTESIAN_POINT('Ctrl Pts',(155.977187707828,8.79775741523248,14.6694065848267));
#28352=CARTESIAN_POINT('Ctrl Pts',(156.094881534311,0.807582648493649,17.0862469651497));
#28353=CARTESIAN_POINT('Ctrl Pts',(156.212575360794,-7.37492681198748,15.4338096271162));
#28354=CARTESIAN_POINT('Ctrl Pts',(156.330269187278,-13.8010163043069,10.1056407048979));
#28355=CARTESIAN_POINT('Ctrl Pts',(156.447963013761,-16.9402419082406,2.37070225429615));
#28356=CARTESIAN_POINT('Ctrl Pts',(156.565656840244,-16.0449625046453,-5.92884502350692));
#28357=CARTESIAN_POINT('Ctrl Pts',(156.683350666727,-11.3283987344367,-12.8163726226201));
#28358=CARTESIAN_POINT('Ctrl Pts',(156.80104449321,-3.91385215684362,-16.651540060385));
#28359=CARTESIAN_POINT('Ctrl Pts',(156.918738319694,4.43282137684879,-16.5209600123355));
#28360=CARTESIAN_POINT('Ctrl Pts',(157.036432146177,11.7237697243691,-12.4557315537146));
#28361=CARTESIAN_POINT('Ctrl Pts',(157.15412597266,16.2225733129014,-5.42403357251556));
#28362=CARTESIAN_POINT('Ctrl Pts',(157.271819799143,16.8577925665448,2.89945768577206));
#28363=CARTESIAN_POINT('Ctrl Pts',(157.389513625626,13.4781430305917,10.5324111928441));
#28364=CARTESIAN_POINT('Ctrl Pts',(157.50720745211,6.8885254290314,15.6569550839818));
#28365=CARTESIAN_POINT('Ctrl Pts',(157.624901278593,-1.34167029936179,17.0526228450654));
#28366=CARTESIAN_POINT('Ctrl Pts',(157.742595105076,-9.25233248327858,14.3870208419639));
#28367=CARTESIAN_POINT('Ctrl Pts',(157.860288931559,-14.9594498809222,8.29499152190118));
#28368=CARTESIAN_POINT('Ctrl Pts',(157.977982758042,-17.1038096874183,0.227418699343366));
#28369=CARTESIAN_POINT('Ctrl Pts',(158.095676584525,-15.1747090200033,-7.89431638879937));
#28370=CARTESIAN_POINT('Ctrl Pts',(158.213370411009,-9.63158442892658,-14.1359331661088));
#28371=CARTESIAN_POINT('Ctrl Pts',(158.331064237492,-1.79459202773081,-17.010921919233));
#28372=CARTESIAN_POINT('Ctrl Pts',(158.448758063975,6.46980221114646,-15.8345724425031));
#28373=CARTESIAN_POINT('Ctrl Pts',(158.566451890458,13.1933418648307,-10.8870453074258));
#28374=CARTESIAN_POINT('Ctrl Pts',(158.684145716941,16.7747419842613,-3.346648539912));
#28375=CARTESIAN_POINT('Ctrl Pts',(158.801839543425,16.3610527240895,4.99078940126682));
#28376=CARTESIAN_POINT('Ctrl Pts',(158.919533369908,12.0507987335361,12.1396159318177));
#28377=CARTESIAN_POINT('Ctrl Pts',(159.037227196391,4.87051442709172,16.3972593534324));
#28378=CARTESIAN_POINT('Ctrl Pts',(159.154921022874,-3.46973648146967,16.7497150374982));
#28379=CARTESIAN_POINT('Ctrl Pts',(159.272614849357,-10.9836314687213,13.11304178471));
#28380=CARTESIAN_POINT('Ctrl Pts',(159.390308675841,-15.8816537664659,6.35335334530791));
#28381=CARTESIAN_POINT('Ctrl Pts',(159.508002502324,-16.9972854705154,-1.91945610057624));
#28382=CARTESIAN_POINT('Ctrl Pts',(159.625696328807,-14.0648266150179,-9.73512595592479));
#28383=CARTESIAN_POINT('Ctrl Pts',(159.74339015529,-7.78267454287779,-15.2322684472103));
#28384=CARTESIAN_POINT('Ctrl Pts',(159.861083981773,0.353007106070388,-17.1016786039061));
#28385=CARTESIAN_POINT('Ctrl Pts',(159.978777808256,8.40461622849572,-14.898135827678));
#28386=CARTESIAN_POINT('Ctrl Pts',(160.09647163474,14.4545735183265,-9.146438076734));
#28387=CARTESIAN_POINT('Ctrl Pts',(160.214165461223,17.0620150780238,-1.21641545761408));
#28388=CARTESIAN_POINT('Ctrl Pts',(160.331859287706,15.6059500099123,7.00330988721436));
#28389=CARTESIAN_POINT('Ctrl Pts',(160.449553114189,10.4331562313559,13.5551199234958));
#28390=CARTESIAN_POINT('Ctrl Pts',(160.567246940672,2.77559149806718,16.8786290001319));
#28391=CARTESIAN_POINT('Ctrl Pts',(160.684940767155,-5.54301089090938,16.182306861245));
#28392=CARTESIAN_POINT('Ctrl Pts',(160.802634593639,-12.5414842452891,11.6319902859914));
#28393=CARTESIAN_POINT('Ctrl Pts',(160.920328420122,-16.5530651300371,4.31138723486822));
#28394=CARTESIAN_POINT('Ctrl Pts',(161.038022246605,-16.6223514171736,-4.03602012534875));
#28395=CARTESIAN_POINT('Ctrl Pts',(161.155716073088,-12.7328418150455,-11.4222048835269));
#28396=CARTESIAN_POINT('Ctrl Pts',(161.273409899572,-5.8108658325,-16.0880658677455));
#28397=CARTESIAN_POINT('Ctrl Pts',(161.391103726055,2.49503178624673,-16.9223769451532));
#28398=CARTESIAN_POINT('Ctrl Pts',(161.508797552538,10.2067101317342,-13.7264377525632));
#28399=CARTESIAN_POINT('Ctrl Pts',(161.626491379021,15.4875481527481,-7.26139637428879));
#28400=CARTESIAN_POINT('Ctrl Pts',(161.744185205504,17.079856168403,0.933026449209681));
#28401=CARTESIAN_POINT('Ctrl Pts',(161.861879031988,14.604408504263,8.90523875754094));
#28402=CARTESIAN_POINT('Ctrl Pts',(161.979572858471,8.65076025942847,14.7565704695287));
#28403=CARTESIAN_POINT('Ctrl Pts',(162.097266684954,0.636838272645602,17.0934625545191));
#28404=CARTESIAN_POINT('Ctrl Pts',(162.214960511437,-7.52875375600992,15.3593584491469));
#28405=CARTESIAN_POINT('Ctrl Pts',(162.33265433792,-13.901290237245,9.96725412683175));
#28406=CARTESIAN_POINT('Ctrl Pts',(162.450348164403,-16.9630814895256,2.2013385623837));
#28407=CARTESIAN_POINT('Ctrl Pts',(162.568041990887,-15.984928236899,-6.08885000246564));
#28408=CARTESIAN_POINT('Ctrl Pts',(162.68573581737,-11.1997884386548,-12.9289119423714));
#28409=CARTESIAN_POINT('Ctrl Pts',(162.803429643853,-3.74729579099151,-16.6898112435252));
#28410=CARTESIAN_POINT('Ctrl Pts',(162.921123470336,4.59765658343188,-16.4758483557211));
#28411=CARTESIAN_POINT('Ctrl Pts',(163.038817296819,11.8476264497369,-12.3379808942753));
#28412=CARTESIAN_POINT('Ctrl Pts',(163.156511123302,16.275953722843,-5.26168752638849));
#28413=CARTESIAN_POINT('Ctrl Pts',(163.274204949786,16.8279835131639,3.06773462333517));
#28414=CARTESIAN_POINT('Ctrl Pts',(163.391898776269,13.3722439005881,10.6665420135521));
#28415=CARTESIAN_POINT('Ctrl Pts',(163.509592602752,6.73175719848808,15.7249950652666));
#28416=CARTESIAN_POINT('Ctrl Pts',(163.627286429235,-1.51197141403623,17.0383674997955));
#28417=CARTESIAN_POINT('Ctrl Pts',(163.744980255719,-9.39560767951175,14.2938652721985));
#28418=CARTESIAN_POINT('Ctrl Pts',(163.862674082202,-15.0415760162977,8.14512168035195));
#28419=CARTESIAN_POINT('Ctrl Pts',(163.980367908685,-17.1052287046836,0.0565278839563854));
#28420=CARTESIAN_POINT('Ctrl Pts',(164.098061735168,-15.0950805326928,-8.04552894975068));
#28421=CARTESIAN_POINT('Ctrl Pts',(164.215755561651,-9.48987782598886,-14.2314539225157));
#28422=CARTESIAN_POINT('Ctrl Pts',(164.333449388134,-1.62454606293885,-17.0280028132521));
#28423=CARTESIAN_POINT('Ctrl Pts',(164.451143214618,6.62766822942697,-15.7691428839178));
#28424=CARTESIAN_POINT('Ctrl Pts',(164.568837041101,13.3014734656906,-10.754693373019));
#28425=CARTESIAN_POINT('Ctrl Pts',(164.686530867584,16.8072981115472,-3.17888441199923));
#28426=CARTESIAN_POINT('Ctrl Pts',(164.804224694067,16.3104609706914,5.15398850889241));
#28427=CARTESIAN_POINT('Ctrl Pts',(164.92191852055,11.9287363733997,12.2594281650536));
#28428=CARTESIAN_POINT('Ctrl Pts',(165.039612347034,4.70681762497127,16.4450537503718));
#28429=CARTESIAN_POINT('Ctrl Pts',(165.157306173517,-3.63765716981974,16.714298405546));
#28430=CARTESIAN_POINT('Ctrl Pts',(165.235768724506,-8.620294072214,14.2392607093337));
#28431=CARTESIAN_POINT('Ctrl Pts',(165.275,-10.6720568218315,12.4855047231419));
#28432=CARTESIAN_POINT('Ctrl Pts',(149.669351500835,9.36921550306818,-13.1405412628083));
#28433=CARTESIAN_POINT('Ctrl Pts',(149.708582776329,11.5286214438524,-11.6008832522912));
#28434=CARTESIAN_POINT('Ctrl Pts',(149.787045327318,15.0718489464266,-7.43816894232811));
#28435=CARTESIAN_POINT('Ctrl Pts',(149.904739153801,16.7970987434091,0.581624345890556));
#28436=CARTESIAN_POINT('Ctrl Pts',(150.022432980285,14.5217411515898,8.46135011476401));
#28437=CARTESIAN_POINT('Ctrl Pts',(150.140126806768,8.78796110611117,14.3266651495927));
#28438=CARTESIAN_POINT('Ctrl Pts',(150.257820633251,0.96118681584472,16.7795619622608));
#28439=CARTESIAN_POINT('Ctrl Pts',(150.375514459734,-7.09448295467532,15.2363995248823));
#28440=CARTESIAN_POINT('Ctrl Pts',(150.493208286218,-13.4605341461659,10.064434093448));
#28441=CARTESIAN_POINT('Ctrl Pts',(150.610902112701,-16.6208058548148,2.49555525516348));
#28442=CARTESIAN_POINT('Ctrl Pts',(150.728595939184,-15.8226522856942,-5.66768815398822));
#28443=CARTESIAN_POINT('Ctrl Pts',(150.846289765667,-11.2561587468171,-12.481099210543));
#28444=CARTESIAN_POINT('Ctrl Pts',(150.96398359215,-4.00888774708244,-16.3220040601612));
#28445=CARTESIAN_POINT('Ctrl Pts',(151.081677418633,4.19314427208089,-16.2756416585466));
#28446=CARTESIAN_POINT('Ctrl Pts',(151.199371245117,11.3965327025307,-12.353057276638));
#28447=CARTESIAN_POINT('Ctrl Pts',(151.3170650716,15.8857115407531,-5.48845581303432));
#28448=CARTESIAN_POINT('Ctrl Pts',(151.434758898083,16.5915333478769,2.68328151621556));
#28449=CARTESIAN_POINT('Ctrl Pts',(151.552452724566,13.3458989445182,10.215965962637));
#28450=CARTESIAN_POINT('Ctrl Pts',(151.670146551049,6.92179185172581,15.3156056408121));
#28451=CARTESIAN_POINT('Ctrl Pts',(151.787840377533,-1.15081612858479,16.7676653468417));
#28452=CARTESIAN_POINT('Ctrl Pts',(151.905534204016,-8.94934458710798,14.2263210366986));
#28453=CARTESIAN_POINT('Ctrl Pts',(152.023228030499,-14.6164881597404,8.2968218440555));
#28454=CARTESIAN_POINT('Ctrl Pts',(152.140921856982,-16.8025542492592,0.391343233840468));
#28455=CARTESIAN_POINT('Ctrl Pts',(152.258615683465,-14.9869071620209,-7.6073380717347));
#28456=CARTESIAN_POINT('Ctrl Pts',(152.376309509948,-9.60196323013091,-13.7942481112521));
#28457=CARTESIAN_POINT('Ctrl Pts',(152.494003336432,-1.93020610249092,-16.6959061816011));
#28458=CARTESIAN_POINT('Ctrl Pts',(152.611697162915,6.20125084689959,-15.6212504864081));
#28459=CARTESIAN_POINT('Ctrl Pts',(152.729390989398,12.8558116734326,-10.8262221038362));
#28460=CARTESIAN_POINT('Ctrl Pts',(152.847084815881,16.4486194947039,-3.45280980406319));
#28461=CARTESIAN_POINT('Ctrl Pts',(152.964778642364,16.1240075956589,4.74292714257176));
#28462=CARTESIAN_POINT('Ctrl Pts',(153.082472468848,11.9592858718244,11.8090838027562));
#28463=CARTESIAN_POINT('Ctrl Pts',(153.200166295331,4.94632862705181,16.0627772174616));
#28464=CARTESIAN_POINT('Ctrl Pts',(153.317860121814,-3.24465120575843,16.4909434956746));
#28465=CARTESIAN_POINT('Ctrl Pts',(153.435553948297,-10.6628816523304,12.9916101270386));
#28466=CARTESIAN_POINT('Ctrl Pts',(153.55324777478,-15.5416295074474,6.39818185720075));
#28467=CARTESIAN_POINT('Ctrl Pts',(153.670941601263,-16.7189672875137,-1.71904382248367));
#28468=CARTESIAN_POINT('Ctrl Pts',(153.788635427747,-13.9144990457088,-9.42686030083935));
#28469=CARTESIAN_POINT('Ctrl Pts',(153.90632925423,-7.79613975197862,-14.8895662728029));
#28470=CARTESIAN_POINT('Ctrl Pts',(154.024023080713,0.178956006267607,-16.8061582038369));
#28471=CARTESIAN_POINT('Ctrl Pts',(154.141716907196,8.11143142253025,-14.7201786368971));
#28472=CARTESIAN_POINT('Ctrl Pts',(154.25941073368,14.1120801937138,-9.12842655832674));
#28473=CARTESIAN_POINT('Ctrl Pts',(154.377104560162,16.7517817885471,-1.36263925287367));
#28474=CARTESIAN_POINT('Ctrl Pts',(154.494798386646,15.4018622270234,6.72767558406047));
#28475=CARTESIAN_POINT('Ctrl Pts',(154.612492213129,10.383819706171,13.2157204546066));
#28476=CARTESIAN_POINT('Ctrl Pts',(154.730186039612,2.89275626691932,16.5562960835077));
#28477=CARTESIAN_POINT('Ctrl Pts',(154.847879866095,-5.28724890691117,15.9538076276774));
#28478=CARTESIAN_POINT('Ctrl Pts',(154.965573692579,-12.2080375768375,11.5517443421804));
#28479=CARTESIAN_POINT('Ctrl Pts',(155.083267519062,-16.2213477702083,4.39850603529533));
#28480=CARTESIAN_POINT('Ctrl Pts',(155.200961345545,-16.3713655051676,-3.80228488159183));
#28481=CARTESIAN_POINT('Ctrl Pts',(155.318655172028,-12.6223624074577,-11.0975198165794));
#28482=CARTESIAN_POINT('Ctrl Pts',(155.436348998512,-5.86720481587589,-15.7497582988799));
#28483=CARTESIAN_POINT('Ctrl Pts',(155.554042824994,2.28529216070807,-16.6510185443647));
#28484=CARTESIAN_POINT('Ctrl Pts',(155.671736651478,9.89352166366411,-13.5866555088138));
#28485=CARTESIAN_POINT('Ctrl Pts',(155.789430477961,15.1455001218973,-7.28648096698123));
#28486=CARTESIAN_POINT('Ctrl Pts',(155.907124304444,16.7904110769446,0.74904919183636));
#28487=CARTESIAN_POINT('Ctrl Pts',(156.024818130927,14.4365008855564,8.60618504367071));
#28488=CARTESIAN_POINT('Ctrl Pts',(156.142511957411,8.64437916038609,14.413663231672));
#28489=CARTESIAN_POINT('Ctrl Pts',(156.260205783894,0.793503422229031,16.7883689244513));
#28490=CARTESIAN_POINT('Ctrl Pts',(156.377899610377,-7.24635388701869,15.1647398318818));
#28491=CARTESIAN_POINT('Ctrl Pts',(156.49559343686,-13.5604122849012,9.92946108749472));
#28492=CARTESIAN_POINT('Ctrl Pts',(156.613287263343,-16.6449092890366,2.32937192915047));
#28493=CARTESIAN_POINT('Ctrl Pts',(156.730981089826,-15.765237998514,-5.8254827846953));
#28494=CARTESIAN_POINT('Ctrl Pts',(156.84867491631,-11.1309018103816,-12.5929346743409));
#28495=CARTESIAN_POINT('Ctrl Pts',(156.966368742793,-3.84561888042886,-16.361240608556));
#28496=CARTESIAN_POINT('Ctrl Pts',(157.084062569276,4.35554050005972,-16.2329370656364));
#28497=CARTESIAN_POINT('Ctrl Pts',(157.201756395759,11.5193799855214,-12.2385809460795));
#28498=CARTESIAN_POINT('Ctrl Pts',(157.319450222242,15.9397523772454,-5.32947211050702));
#28499=CARTESIAN_POINT('Ctrl Pts',(157.437144048726,16.5638973518458,2.84890914949683));
#28500=CARTESIAN_POINT('Ctrl Pts',(157.554837875209,13.2431679160219,10.3487913483953));
#28501=CARTESIAN_POINT('Ctrl Pts',(157.672531701692,6.76843232360655,15.3839950177231));
#28502=CARTESIAN_POINT('Ctrl Pts',(157.790225528175,-1.31827990117477,16.755331000214));
#28503=CARTESIAN_POINT('Ctrl Pts',(157.907919354658,-9.0910292621774,14.1362005425364));
#28504=CARTESIAN_POINT('Ctrl Pts',(158.025613181142,-14.6986499738657,8.15037838203533));
#28505=CARTESIAN_POINT('Ctrl Pts',(158.143307007625,-16.8056254619089,0.223453929507307));
#28506=CARTESIAN_POINT('Ctrl Pts',(158.261000834108,-14.9101563303303,-7.75668853504396));
#28507=CARTESIAN_POINT('Ctrl Pts',(158.378694660591,-9.46366940906519,-13.8894902764823));
#28508=CARTESIAN_POINT('Ctrl Pts',(158.496388487074,-1.76330548726561,-16.7143570795634));
#28509=CARTESIAN_POINT('Ctrl Pts',(158.614082313557,6.35700903835122,-15.5585158325238));
#28510=CARTESIAN_POINT('Ctrl Pts',(158.731776140041,12.9633319139634,-10.6972428463128));
#28511=CARTESIAN_POINT('Ctrl Pts',(158.849469966524,16.4822946559695,-3.28830377221617));
#28512=CARTESIAN_POINT('Ctrl Pts',(158.967163793007,16.0758175674659,4.90378102713882));
#28513=CARTESIAN_POINT('Ctrl Pts',(159.08485761949,11.8407076396336,11.927976417536));
#28514=CARTESIAN_POINT('Ctrl Pts',(159.202551445973,4.78560290160023,16.1113929780379));
#28515=CARTESIAN_POINT('Ctrl Pts',(159.320245272457,-3.40924582445485,16.4577040237394));
#28516=CARTESIAN_POINT('Ctrl Pts',(159.43793909894,-10.7921451447597,12.8844317685729));
#28517=CARTESIAN_POINT('Ctrl Pts',(159.555632925423,-15.6047763505738,6.2425903175801));
#28518=CARTESIAN_POINT('Ctrl Pts',(159.673326751906,-16.7009583658286,-1.88599270609223));
#28519=CARTESIAN_POINT('Ctrl Pts',(159.791020578389,-13.8196233820674,-9.56540581483018));
#28520=CARTESIAN_POINT('Ctrl Pts',(159.908714404873,-7.64699302961428,-14.9667122785735));
#28521=CARTESIAN_POINT('Ctrl Pts',(160.026408231356,0.346852854330788,-16.803531531259));
#28522=CARTESIAN_POINT('Ctrl Pts',(160.144102057839,8.25809191452131,-14.638404856947));
#28523=CARTESIAN_POINT('Ctrl Pts',(160.261795884322,14.2025755197285,-8.98698099647384));
#28524=CARTESIAN_POINT('Ctrl Pts',(160.379489710805,16.7645594909558,-1.19520872602881));
#28525=CARTESIAN_POINT('Ctrl Pts',(160.497183537289,15.3338791554016,6.88121565365554));
#28526=CARTESIAN_POINT('Ctrl Pts',(160.614877363772,10.2512667770577,13.3188028099438));
#28527=CARTESIAN_POINT('Ctrl Pts',(160.732571190255,2.72720241889082,16.5843705274264));
#28528=CARTESIAN_POINT('Ctrl Pts',(160.850265016738,-5.44637520332267,15.9001879224494));
#28529=CARTESIAN_POINT('Ctrl Pts',(160.967958843221,-12.3228386432412,11.4292006105945));
#28530=CARTESIAN_POINT('Ctrl Pts',(161.085652669705,-16.2644824694596,4.23622341540371));
#28531=CARTESIAN_POINT('Ctrl Pts',(161.203346496188,-16.3325608340194,-3.96565699823196));
#28532=CARTESIAN_POINT('Ctrl Pts',(161.321040322671,-12.5108601253202,-11.223072562772));
#28533=CARTESIAN_POINT('Ctrl Pts',(161.438734149154,-5.70956041812335,-15.8075899066357));
#28534=CARTESIAN_POINT('Ctrl Pts',(161.556427975637,2.45153392615592,-16.6273557799633));
#28535=CARTESIAN_POINT('Ctrl Pts',(161.674121802121,10.0287684911728,-13.4871339199638));
#28536=CARTESIAN_POINT('Ctrl Pts',(161.791815628603,15.2175414913454,-7.13480271512424));
#28537=CARTESIAN_POINT('Ctrl Pts',(161.909509455087,16.7820895435127,0.916760262072329));
#28538=CARTESIAN_POINT('Ctrl Pts',(162.02720328157,14.3497983139923,8.74998669554875));
#28539=CARTESIAN_POINT('Ctrl Pts',(162.144897108053,8.49994472212025,14.4993075195166));
#28540=CARTESIAN_POINT('Ctrl Pts',(162.262590934536,0.625735767965398,16.7954587187512));
#28541=CARTESIAN_POINT('Ctrl Pts',(162.38028476102,-7.39749904440972,15.0915866201111));
#28542=CARTESIAN_POINT('Ctrl Pts',(162.497978587503,-13.6589380631546,9.79348711196305));
#28543=CARTESIAN_POINT('Ctrl Pts',(162.615672413986,-16.6673506898589,2.16296088826871));
#28544=CARTESIAN_POINT('Ctrl Pts',(162.733366240469,-15.7062503555818,-5.9826982704592));
#28545=CARTESIAN_POINT('Ctrl Pts',(162.851060066952,-11.0045336794823,-12.70351200723));
#28546=CARTESIAN_POINT('Ctrl Pts',(162.968753893435,-3.68196622327458,-16.3988445799281));
#28547=CARTESIAN_POINT('Ctrl Pts',(163.086447719919,4.51750200427417,-16.1886118761679));
#28548=CARTESIAN_POINT('Ctrl Pts',(163.204141546402,11.6410774187547,-12.1228831269039));
#28549=CARTESIAN_POINT('Ctrl Pts',(163.321835372885,15.9922021643325,-5.16995637124805));
#28550=CARTESIAN_POINT('Ctrl Pts',(163.439529199368,16.5346079832404,3.0142523822763));
#28551=CARTESIAN_POINT('Ctrl Pts',(163.557223025851,13.1391150092071,10.4805837605487));
#28552=CARTESIAN_POINT('Ctrl Pts',(163.674916852335,6.61439715746602,15.4508488042657));
#28553=CARTESIAN_POINT('Ctrl Pts',(163.792610678818,-1.48561202198696,16.7413241796393));
#28554=CARTESIAN_POINT('Ctrl Pts',(163.910304505301,-9.2318066287338,14.0446690274074));
#28555=CARTESIAN_POINT('Ctrl Pts',(164.027998331784,-14.7793443394474,8.00312133982417));
#28556=CARTESIAN_POINT('Ctrl Pts',(164.145692158267,-16.8070197403253,0.0555423887009042));
#28557=CARTESIAN_POINT('Ctrl Pts',(164.26338598475,-14.831916069342,-7.90526488796918));
#28558=CARTESIAN_POINT('Ctrl Pts',(164.381079811234,-9.32443328927823,-13.9833457440858));
#28559=CARTESIAN_POINT('Ctrl Pts',(164.498773637717,-1.59622406810641,-16.7311401888639));
#28560=CARTESIAN_POINT('Ctrl Pts',(164.6164674642,6.51212285362811,-15.4942269591197));
#28561=CARTESIAN_POINT('Ctrl Pts',(164.734161290683,13.0695783712066,-10.5671983077305));
#28562=CARTESIAN_POINT('Ctrl Pts',(164.851855117166,16.5142832065705,-3.1234644088713));
#28563=CARTESIAN_POINT('Ctrl Pts',(164.96954894365,16.0261078200699,5.06413495580132));
#28564=CARTESIAN_POINT('Ctrl Pts',(165.087242770133,11.7207732890452,12.0456998694637));
#28565=CARTESIAN_POINT('Ctrl Pts',(165.204936596616,4.62475995514413,16.1583541375));
#28566=CARTESIAN_POINT('Ctrl Pts',(165.322630423099,-3.57423901879522,16.4229048379096));
#28567=CARTESIAN_POINT('Ctrl Pts',(165.401092974088,-8.47000967601441,13.9910164290221));
#28568=CARTESIAN_POINT('Ctrl Pts',(165.440324249582,-10.486002424819,12.2678350563248));
#28569=CARTESIAN_POINT('Ctrl Pts',(149.834675750418,9.20297639017438,-12.9073870652388));
#28570=CARTESIAN_POINT('Ctrl Pts',(149.873907025912,11.3240677327026,-11.395047391219));
#28571=CARTESIAN_POINT('Ctrl Pts',(149.952369576901,14.8044273252991,-7.30619261985777));
#28572=CARTESIAN_POINT('Ctrl Pts',(150.070063403384,16.4990658084874,0.571304515455822));
#28573=CARTESIAN_POINT('Ctrl Pts',(150.187757229867,14.2640801589567,8.3112193661969));
#28574=CARTESIAN_POINT('Ctrl Pts',(150.30545105635,8.63203525960385,14.0724654138288));
#28575=CARTESIAN_POINT('Ctrl Pts',(150.423144882833,0.944132363042452,16.4818401845475));
#28576=CARTESIAN_POINT('Ctrl Pts',(150.540838709317,-6.96860469384984,14.9660582631318));
#28577=CARTESIAN_POINT('Ctrl Pts',(150.6585325358,-13.221702276539,9.88585963383337));
#28578=CARTESIAN_POINT('Ctrl Pts',(150.776226362283,-16.3259009057313,2.45127631935929));
#28579=CARTESIAN_POINT('Ctrl Pts',(150.893920188766,-15.5419090709886,-5.5671256842095));
#28580=CARTESIAN_POINT('Ctrl Pts',(151.011614015249,-11.0564393739357,-12.2596455722933));
#28581=CARTESIAN_POINT('Ctrl Pts',(151.129307841733,-3.93775757161068,-16.03240078711));
#28582=CARTESIAN_POINT('Ctrl Pts',(151.247001668216,4.11874481101629,-15.9868609991405));
#28583=CARTESIAN_POINT('Ctrl Pts',(151.364695494699,11.1943226577395,-12.1338755017581));
#28584=CARTESIAN_POINT('Ctrl Pts',(151.482389321182,15.6038494581319,-5.39107348414916));
#28585=CARTESIAN_POINT('Ctrl Pts',(151.600083147665,16.2971477843902,2.63567173087615));
#28586=CARTESIAN_POINT('Ctrl Pts',(151.717776974149,13.1091010610049,10.0347028549172));
#28587=CARTESIAN_POINT('Ctrl Pts',(151.835470800632,6.79897766982448,15.0438590154596));
#28588=CARTESIAN_POINT('Ctrl Pts',(151.953164627115,-1.13039706017324,16.4701546522007));
#28589=CARTESIAN_POINT('Ctrl Pts',(152.070858453598,-8.79055529416723,13.9739017185488));
#28590=CARTESIAN_POINT('Ctrl Pts',(152.188552280082,-14.3571460595931,8.14961034030235));
#28591=CARTESIAN_POINT('Ctrl Pts',(152.306246106564,-16.5044245166437,0.384399583968249));
#28592=CARTESIAN_POINT('Ctrl Pts',(152.423939933048,-14.7209926731482,-7.47236016113865));
#28593=CARTESIAN_POINT('Ctrl Pts',(152.541633759531,-9.43159444643784,-13.5494951147712));
#28594=CARTESIAN_POINT('Ctrl Pts',(152.659327586014,-1.89595822441881,-16.3996687184241));
#28595=CARTESIAN_POINT('Ctrl Pts',(152.777021412497,6.09122131035165,-15.3440807679507));
#28596=CARTESIAN_POINT('Ctrl Pts',(152.89471523898,12.6277094670717,-10.6341311483081));
#28597=CARTESIAN_POINT('Ctrl Pts',(153.012409065464,16.156769668832,-3.39154618614015));
#28598=CARTESIAN_POINT('Ctrl Pts',(153.130102891947,15.8379173975929,4.65877281818433));
#28599=CARTESIAN_POINT('Ctrl Pts',(153.24779671843,11.7470908301451,11.5995538143793));
#28600=CARTESIAN_POINT('Ctrl Pts',(153.365490544913,4.85856532576227,15.77777343733));
#28601=CARTESIAN_POINT('Ctrl Pts',(153.483184371396,-3.18708097077789,16.1983427099839));
#28602=CARTESIAN_POINT('Ctrl Pts',(153.60087819788,-10.4736888659979,12.7610984324496));
#28603=CARTESIAN_POINT('Ctrl Pts',(153.718572024363,-15.2658725135565,6.28465815014907));
#28604=CARTESIAN_POINT('Ctrl Pts',(153.836265850846,-16.4223206483723,-1.6885426220383));
#28605=CARTESIAN_POINT('Ctrl Pts',(153.953959677329,-13.6676124224945,-9.25959838939414));
#28606=CARTESIAN_POINT('Ctrl Pts',(154.071653503812,-7.65781191055575,-14.6253789149869));
#28607=CARTESIAN_POINT('Ctrl Pts',(154.189347330296,0.175780768413483,-16.5079645258236));
#28608=CARTESIAN_POINT('Ctrl Pts',(154.307041156779,7.9675093232319,-14.4589967441938));
#28609=CARTESIAN_POINT('Ctrl Pts',(154.424734983262,13.8616878645245,-8.96645979252062));
#28610=CARTESIAN_POINT('Ctrl Pts',(154.542428809745,16.4545529177835,-1.33846178139616));
#28611=CARTESIAN_POINT('Ctrl Pts',(154.660122636228,15.12858514073,6.60830563034714));
#28612=CARTESIAN_POINT('Ctrl Pts',(154.777816462711,10.1995783493746,12.9812323436322));
#28613=CARTESIAN_POINT('Ctrl Pts',(154.895510289195,2.84142974598773,16.2625357390233));
#28614=CARTESIAN_POINT('Ctrl Pts',(155.013204115678,-5.19343661626147,15.6707373080295));
#28615=CARTESIAN_POINT('Ctrl Pts',(155.130897942161,-11.9914289038613,11.3467803586759));
#28616=CARTESIAN_POINT('Ctrl Pts',(155.248591768644,-15.9335304537662,4.32046281586825));
#28617=CARTESIAN_POINT('Ctrl Pts',(155.366285595128,-16.0808864060852,-3.73482048550892));
#28618=CARTESIAN_POINT('Ctrl Pts',(155.483979421611,-12.3984023193849,-10.9006151932387));
#28619=CARTESIAN_POINT('Ctrl Pts',(155.601673248094,-5.76310229806762,-15.4703084509134));
#28620=CARTESIAN_POINT('Ctrl Pts',(155.719367074577,2.24474394817366,-16.3555775279118));
#28621=CARTESIAN_POINT('Ctrl Pts',(155.83706090106,9.71797972376269,-13.3455858527429));
#28622=CARTESIAN_POINT('Ctrl Pts',(155.954754727543,14.8767716991417,-7.15719606242632));
#28623=CARTESIAN_POINT('Ctrl Pts',(156.072448554027,16.4924968020899,0.735758722306252));
#28624=CARTESIAN_POINT('Ctrl Pts',(156.19014238051,14.1803523211734,8.45348447161203));
#28625=CARTESIAN_POINT('Ctrl Pts',(156.307836206993,8.49100090553969,14.1579198785174));
#28626=CARTESIAN_POINT('Ctrl Pts',(156.425530033476,0.77942419596441,16.490490883753));
#28627=CARTESIAN_POINT('Ctrl Pts',(156.543223859959,-7.1177809620499,14.8956700366474));
#28628=CARTESIAN_POINT('Ctrl Pts',(156.660917686442,-13.3198082654956,9.75328147009152));
#28629=CARTESIAN_POINT('Ctrl Pts',(156.778611512926,-16.3495766698327,2.28804160400477));
#28630=CARTESIAN_POINT('Ctrl Pts',(156.896305339409,-15.4855134923828,-5.72212054588366));
#28631=CARTESIAN_POINT('Ctrl Pts',(157.013999165892,-10.9334048863264,-12.3694967260616));
#28632=CARTESIAN_POINT('Ctrl Pts',(157.131692992375,-3.7773856040141,-16.070941156727));
#28633=CARTESIAN_POINT('Ctrl Pts',(157.249386818858,4.27825962327065,-15.9449141189373));
#28634=CARTESIAN_POINT('Ctrl Pts',(157.367080645342,11.3149902466737,-12.0214303384444));
#28635=CARTESIAN_POINT('Ctrl Pts',(157.484774471825,15.6569314415894,-5.23491064849851));
#28636=CARTESIAN_POINT('Ctrl Pts',(157.602468298308,16.2700021371469,2.79836061322161));
#28637=CARTESIAN_POINT('Ctrl Pts',(157.720162124791,13.008192801452,10.1651715039466));
#28638=CARTESIAN_POINT('Ctrl Pts',(157.837855951274,6.64833921818169,15.1110349514645));
#28639=CARTESIAN_POINT('Ctrl Pts',(157.955549777758,-1.29488950298773,16.4580391553625));
#28640=CARTESIAN_POINT('Ctrl Pts',(158.073243604241,-8.92972604107625,13.8853802431089));
#28641=CARTESIAN_POINT('Ctrl Pts',(158.190937430724,-14.4378500668093,8.00576524216949));
#28642=CARTESIAN_POINT('Ctrl Pts',(158.308631257207,-16.5074412363995,0.219489159671254));
#28643=CARTESIAN_POINT('Ctrl Pts',(158.426325083691,-14.6456036406574,-7.61906068128856));
#28644=CARTESIAN_POINT('Ctrl Pts',(158.544018910173,-9.29575438920379,-13.6430473868558));
#28645=CARTESIAN_POINT('Ctrl Pts',(158.661712736657,-1.73201894680041,-16.4177922398939));
#28646=CARTESIAN_POINT('Ctrl Pts',(158.77940656314,6.24421586555601,-15.2824592225444));
#28647=CARTESIAN_POINT('Ctrl Pts',(158.897100389623,12.7333219630962,-10.5074403851997));
#28648=CARTESIAN_POINT('Ctrl Pts',(159.014794216106,16.1898473276777,-3.22995900452034));
#28649=CARTESIAN_POINT('Ctrl Pts',(159.13248804259,15.7905824108423,4.81677265301081));
#28650=CARTESIAN_POINT('Ctrl Pts',(159.250181869073,11.6306165457311,11.7163369032544));
#28651=CARTESIAN_POINT('Ctrl Pts',(159.367875695556,4.70069137610872,15.8255266026433));
#28652=CARTESIAN_POINT('Ctrl Pts',(159.485569522039,-3.34875516744001,16.1656930099807));
#28653=CARTESIAN_POINT('Ctrl Pts',(159.603263348522,-10.6006588207982,12.6558217524358));
#28654=CARTESIAN_POINT('Ctrl Pts',(159.720957175005,-15.3278989346817,6.13182728985231));
#28655=CARTESIAN_POINT('Ctrl Pts',(159.838651001489,-16.4046312611417,-1.85252931160823));
#28656=CARTESIAN_POINT('Ctrl Pts',(159.956344827972,-13.574420149117,-9.39568567373559));
#28657=CARTESIAN_POINT('Ctrl Pts',(160.074038654455,-7.51131151635076,-14.7011561099368));
#28658=CARTESIAN_POINT('Ctrl Pts',(160.191732480938,0.34069860259118,-16.5053844586119));
#28659=CARTESIAN_POINT('Ctrl Pts',(160.309426307421,8.11156760054691,-14.3786738862161));
#28660=CARTESIAN_POINT('Ctrl Pts',(160.427120133905,13.9505775211304,-8.8275239162137));
#28661=CARTESIAN_POINT('Ctrl Pts',(160.544813960388,16.4671039038878,-1.17400199444354));
#28662=CARTESIAN_POINT('Ctrl Pts',(160.662507786871,15.0618083008908,6.75912142009672));
#28663=CARTESIAN_POINT('Ctrl Pts',(160.780201613354,10.0693773227594,13.0824856963917));
#28664=CARTESIAN_POINT('Ctrl Pts',(160.897895439837,2.67881333971445,16.2901120547209));
#28665=CARTESIAN_POINT('Ctrl Pts',(161.01558926632,-5.34973951573596,15.6180689836538));
#28666=CARTESIAN_POINT('Ctrl Pts',(161.133283092804,-12.1041930411931,11.2264109351977));
#28667=CARTESIAN_POINT('Ctrl Pts',(161.250976919287,-15.975899808882,4.16105959593918));
#28668=CARTESIAN_POINT('Ctrl Pts',(161.36867074577,-16.0427702508652,-3.89529387111515));
#28669=CARTESIAN_POINT('Ctrl Pts',(161.486364572253,-12.2888784355949,-11.0239402420172));
#28670=CARTESIAN_POINT('Ctrl Pts',(161.604058398736,-5.60825500374669,-15.5271139455259));
#28671=CARTESIAN_POINT('Ctrl Pts',(161.72175222522,2.40803606606511,-16.3323346147733));
#28672=CARTESIAN_POINT('Ctrl Pts',(161.839446051703,9.85082685061131,-13.2478300873643));
#28673=CARTESIAN_POINT('Ctrl Pts',(161.957139878186,14.9475348299427,-7.00820905595969));
#28674=CARTESIAN_POINT('Ctrl Pts',(162.074833704669,16.4843229186225,0.900494074934982));
#28675=CARTESIAN_POINT('Ctrl Pts',(162.192527531152,14.0951881237216,8.59473463355657));
#28676=CARTESIAN_POINT('Ctrl Pts',(162.310221357636,8.34912918481203,14.2420445695044));
#28677=CARTESIAN_POINT('Ctrl Pts',(162.427915184119,0.614633263285196,16.4974548829834));
#28678=CARTESIAN_POINT('Ctrl Pts',(162.545609010602,-7.26624433280952,14.8238147910752));
#28679=CARTESIAN_POINT('Ctrl Pts',(162.663302837085,-13.4165858890642,9.61972009709434));
#28680=CARTESIAN_POINT('Ctrl Pts',(162.780996663568,-16.3716198901922,2.12458321415372));
#28681=CARTESIAN_POINT('Ctrl Pts',(162.898690490051,-15.4275724742645,-5.87654653845276));
#28682=CARTESIAN_POINT('Ctrl Pts',(163.016384316535,-10.8092789203097,-12.4781120720886));
#28683=CARTESIAN_POINT('Ctrl Pts',(163.134078143018,-3.61663665555766,-16.1078779163309));
#28684=CARTESIAN_POINT('Ctrl Pts',(163.251771969501,4.43734742511645,-15.9013753966148));
#28685=CARTESIAN_POINT('Ctrl Pts',(163.369465795984,11.4345283877725,-11.9077853595324));
#28686=CARTESIAN_POINT('Ctrl Pts',(163.487159622467,15.7084506058219,-5.07822521610762));
#28687=CARTESIAN_POINT('Ctrl Pts',(163.604853448951,16.2412324533168,2.96077014121744));
#28688=CARTESIAN_POINT('Ctrl Pts',(163.722547275434,12.9059861178261,10.2946255075453));
#28689=CARTESIAN_POINT('Ctrl Pts',(163.840241101917,6.49703711644397,15.1767025432649));
#28690=CARTESIAN_POINT('Ctrl Pts',(163.9579349284,-1.45925262993771,16.444280859483));
#28691=CARTESIAN_POINT('Ctrl Pts',(164.075628754883,-9.06800557795583,13.7954727826163));
#28692=CARTESIAN_POINT('Ctrl Pts',(164.193322581366,-14.517112662597,7.86112099929637));
#28693=CARTESIAN_POINT('Ctrl Pts',(164.31101640785,-16.5088107759669,0.0545568934454388));
#28694=CARTESIAN_POINT('Ctrl Pts',(164.428710234333,-14.5687516059912,-7.7650008261877));
#28695=CARTESIAN_POINT('Ctrl Pts',(164.546404060816,-9.15898875256761,-13.7352375656558));
#28696=CARTESIAN_POINT('Ctrl Pts',(164.664097887299,-1.56790207327398,-16.4342775644758));
#28697=CARTESIAN_POINT('Ctrl Pts',(164.781791713783,6.39657747782926,-15.2193110343215));
#28698=CARTESIAN_POINT('Ctrl Pts',(164.899485540266,12.8376832767225,-10.379703242442));
#28699=CARTESIAN_POINT('Ctrl Pts',(165.017179366749,16.2212683015939,-3.06804440574336));
#28700=CARTESIAN_POINT('Ctrl Pts',(165.134873193232,15.7417546694485,4.97428140271022));
#28701=CARTESIAN_POINT('Ctrl Pts',(165.252567019715,11.5128102046906,11.8319715738739));
#28702=CARTESIAN_POINT('Ctrl Pts',(165.370260846199,4.542702285317,15.8716545246283));
#28703=CARTESIAN_POINT('Ctrl Pts',(165.487954672682,-3.51082086777072,16.1315112702732));
#28704=CARTESIAN_POINT('Ctrl Pts',(165.56641722367,-8.31972527981482,13.7427721487105));
#28705=CARTESIAN_POINT('Ctrl Pts',(165.605648499165,-10.2999480278064,12.0501653895076));
#28706=CARTESIAN_POINT('Ctrl Pts',(150.,9.03673727728059,-12.6742328676692));
#28707=CARTESIAN_POINT('Ctrl Pts',(150.039231275494,11.1195140215529,-11.1892115301467));
#28708=CARTESIAN_POINT('Ctrl Pts',(150.117693826483,14.5370057041716,-7.17421629738743));
#28709=CARTESIAN_POINT('Ctrl Pts',(150.235387652966,16.2010328735656,0.560984685021083));
#28710=CARTESIAN_POINT('Ctrl Pts',(150.35308147945,14.0064191663237,8.1610886176298));
#28711=CARTESIAN_POINT('Ctrl Pts',(150.470775305933,8.47610941309655,13.8182656780649));
#28712=CARTESIAN_POINT('Ctrl Pts',(150.588469132416,0.927077910240183,16.1841184068341));
#28713=CARTESIAN_POINT('Ctrl Pts',(150.706162958899,-6.84272643302437,14.6957170013813));
#28714=CARTESIAN_POINT('Ctrl Pts',(150.823856785382,-12.9828704069121,9.70728517421879));
#28715=CARTESIAN_POINT('Ctrl Pts',(150.941550611866,-16.0309959566478,2.40699738355509));
#28716=CARTESIAN_POINT('Ctrl Pts',(151.059244438349,-15.261165856283,-5.46656321443077));
#28717=CARTESIAN_POINT('Ctrl Pts',(151.176938264832,-10.8567200010544,-12.0381919340435));
#28718=CARTESIAN_POINT('Ctrl Pts',(151.294632091315,-3.86662739613892,-15.7427975140589));
#28719=CARTESIAN_POINT('Ctrl Pts',(151.412325917798,4.04434534995169,-15.6980803397344));
#28720=CARTESIAN_POINT('Ctrl Pts',(151.530019744281,10.9921126129483,-11.9146937268782));
#28721=CARTESIAN_POINT('Ctrl Pts',(151.647713570765,15.3219873755107,-5.293691155264));
#28722=CARTESIAN_POINT('Ctrl Pts',(151.765407397248,16.0027622209035,2.58806194553672));
#28723=CARTESIAN_POINT('Ctrl Pts',(151.883101223731,12.8723031774915,9.8534397471975));
#28724=CARTESIAN_POINT('Ctrl Pts',(152.000795050214,6.67616348792316,14.772112390107));
#28725=CARTESIAN_POINT('Ctrl Pts',(152.118488876698,-1.1099779917617,16.1726439575597));
#28726=CARTESIAN_POINT('Ctrl Pts',(152.23618270318,-8.63176600122648,13.7214824003989));
#28727=CARTESIAN_POINT('Ctrl Pts',(152.353876529664,-14.0978039594459,8.00239883654923));
#28728=CARTESIAN_POINT('Ctrl Pts',(152.471570356147,-16.2062947840282,0.377455934096013));
#28729=CARTESIAN_POINT('Ctrl Pts',(152.58926418263,-14.4550781842755,-7.33738225054259));
#28730=CARTESIAN_POINT('Ctrl Pts',(152.706958009113,-9.26122566274478,-13.3047421182903));
#28731=CARTESIAN_POINT('Ctrl Pts',(152.824651835596,-1.8617103463467,-16.1034312552471));
#28732=CARTESIAN_POINT('Ctrl Pts',(152.94234566208,5.98119177380371,-15.0669110494933));
#28733=CARTESIAN_POINT('Ctrl Pts',(153.060039488563,12.3996072607107,-10.44204019278));
#28734=CARTESIAN_POINT('Ctrl Pts',(153.177733315046,15.86491984296,-3.3302825682171));
#28735=CARTESIAN_POINT('Ctrl Pts',(153.295427141529,15.551827199527,4.5746184937969));
#28736=CARTESIAN_POINT('Ctrl Pts',(153.413120968012,11.5348957884658,11.3900238260024));
#28737=CARTESIAN_POINT('Ctrl Pts',(153.530814794496,4.77080202447272,15.4927696571985));
#28738=CARTESIAN_POINT('Ctrl Pts',(153.648508620979,-3.12951073579735,15.9057419242933));
#28739=CARTESIAN_POINT('Ctrl Pts',(153.766202447462,-10.2844960796655,12.5305867378607));
#28740=CARTESIAN_POINT('Ctrl Pts',(153.883896273945,-14.9901155196656,6.17113444309738));
#28741=CARTESIAN_POINT('Ctrl Pts',(154.001590100428,-16.1256740092309,-1.6580414215929));
#28742=CARTESIAN_POINT('Ctrl Pts',(154.119283926912,-13.4207257992801,-9.09233647794895));
#28743=CARTESIAN_POINT('Ctrl Pts',(154.236977753395,-7.51948406913288,-14.3611915571709));
#28744=CARTESIAN_POINT('Ctrl Pts',(154.354671579878,0.172605530559356,-16.2097708478104));
#28745=CARTESIAN_POINT('Ctrl Pts',(154.472365406361,7.82358722393355,-14.1978148514905));
#28746=CARTESIAN_POINT('Ctrl Pts',(154.590059232844,13.6112955353353,-8.80449302671448));
#28747=CARTESIAN_POINT('Ctrl Pts',(154.707753059327,16.1573240470198,-1.31428430991864));
#28748=CARTESIAN_POINT('Ctrl Pts',(154.825446885811,14.8553080544366,6.48893567663383));
#28749=CARTESIAN_POINT('Ctrl Pts',(154.943140712294,10.0153369925782,12.7467442326578));
#28750=CARTESIAN_POINT('Ctrl Pts',(155.060834538777,2.79010322505614,15.968775394539));
#28751=CARTESIAN_POINT('Ctrl Pts',(155.17852836526,-5.09962432561176,15.3876669883817));
#28752=CARTESIAN_POINT('Ctrl Pts',(155.296222191744,-11.7748202308851,11.1418163751715));
#28753=CARTESIAN_POINT('Ctrl Pts',(155.413916018227,-15.645713137324,4.24241959644116));
#28754=CARTESIAN_POINT('Ctrl Pts',(155.53160984471,-15.7904073070029,-3.66735608942599));
#28755=CARTESIAN_POINT('Ctrl Pts',(155.649303671193,-12.1744422313121,-10.703710569898));
#28756=CARTESIAN_POINT('Ctrl Pts',(155.766997497676,-5.65899978025936,-15.1908586029469));
#28757=CARTESIAN_POINT('Ctrl Pts',(155.884691324159,2.20419573563924,-16.0601365114588));
#28758=CARTESIAN_POINT('Ctrl Pts',(156.002385150643,9.54243778386128,-13.104516196672));
#28759=CARTESIAN_POINT('Ctrl Pts',(156.120078977126,14.6080432763861,-7.02791115787139));
#28760=CARTESIAN_POINT('Ctrl Pts',(156.237772803609,16.1945825272352,0.72246825277614));
#28761=CARTESIAN_POINT('Ctrl Pts',(156.355466630092,13.9242037567905,8.30078389955334));
#28762=CARTESIAN_POINT('Ctrl Pts',(156.473160456575,8.3376226506933,13.9021765253628));
#28763=CARTESIAN_POINT('Ctrl Pts',(156.590854283059,0.765344969699789,16.1926128430546));
#28764=CARTESIAN_POINT('Ctrl Pts',(156.708548109542,-6.9892080370811,14.626600241413));
#28765=CARTESIAN_POINT('Ctrl Pts',(156.826241936025,-13.0792042460899,9.5771018526883));
#28766=CARTESIAN_POINT('Ctrl Pts',(156.943935762508,-16.0542440506288,2.24671127885909));
#28767=CARTESIAN_POINT('Ctrl Pts',(157.061629588991,-15.2057889862516,-5.61875830707204));
#28768=CARTESIAN_POINT('Ctrl Pts',(157.179323415475,-10.7359079622712,-12.1460587777823));
#28769=CARTESIAN_POINT('Ctrl Pts',(157.297017241958,-3.70915232759935,-15.780641704898));
#28770=CARTESIAN_POINT('Ctrl Pts',(157.414711068441,4.20097874648159,-15.6568911722382));
#28771=CARTESIAN_POINT('Ctrl Pts',(157.532404894924,11.1106005078261,-11.8042797308094));
#28772=CARTESIAN_POINT('Ctrl Pts',(157.650098721407,15.3741105059335,-5.14034918648998));
#28773=CARTESIAN_POINT('Ctrl Pts',(157.76779254789,15.976106922448,2.74781207694638));
#28774=CARTESIAN_POINT('Ctrl Pts',(157.885486374374,12.7732176868821,9.98155165949782));
#28775=CARTESIAN_POINT('Ctrl Pts',(158.003180200857,6.52824611275682,14.8380748852059));
#28776=CARTESIAN_POINT('Ctrl Pts',(158.12087402734,-1.27149910480069,16.1607473105111));
#28777=CARTESIAN_POINT('Ctrl Pts',(158.238567853823,-8.76842281997508,13.6345599436814));
#28778=CARTESIAN_POINT('Ctrl Pts',(158.356261680306,-14.1770501597529,7.86115210230364));
#28779=CARTESIAN_POINT('Ctrl Pts',(158.47395550679,-16.20925701089,0.215524389835196));
#28780=CARTESIAN_POINT('Ctrl Pts',(158.591649333273,-14.3810509509845,-7.48143282753315));
#28781=CARTESIAN_POINT('Ctrl Pts',(158.709343159756,-9.12783936934241,-13.3966044972293));
#28782=CARTESIAN_POINT('Ctrl Pts',(158.827036986239,-1.70073240633521,-16.1212274002243));
#28783=CARTESIAN_POINT('Ctrl Pts',(158.944730812722,6.13142269276078,-15.0064026125651));
#28784=CARTESIAN_POINT('Ctrl Pts',(159.062424639206,12.503312012229,-10.3176379240867));
#28785=CARTESIAN_POINT('Ctrl Pts',(159.180118465689,15.8973999993859,-3.17161423682451));
#28786=CARTESIAN_POINT('Ctrl Pts',(159.297812292172,15.5053472542187,4.7297642788828));
#28787=CARTESIAN_POINT('Ctrl Pts',(159.415506118655,11.4205254518286,11.5046973889728));
#28788=CARTESIAN_POINT('Ctrl Pts',(159.533199945138,4.61577985061722,15.5396602272488));
#28789=CARTESIAN_POINT('Ctrl Pts',(159.650893771622,-3.28826451042518,15.8736819962219));
#28790=CARTESIAN_POINT('Ctrl Pts',(159.768587598105,-10.4091724968367,12.4272117362987));
#28791=CARTESIAN_POINT('Ctrl Pts',(159.886281424588,-15.0510215187897,6.02106426212451));
#28792=CARTESIAN_POINT('Ctrl Pts',(160.003975251071,-16.1083041564548,-1.81906591712422));
#28793=CARTESIAN_POINT('Ctrl Pts',(160.121669077554,-13.3292169161666,-9.22596553264098));
#28794=CARTESIAN_POINT('Ctrl Pts',(160.239362904037,-7.37563000308724,-14.4355999413));
#28795=CARTESIAN_POINT('Ctrl Pts',(160.357056730521,0.334544350851575,-16.2072373859648));
#28796=CARTESIAN_POINT('Ctrl Pts',(160.474750557004,7.96504328657251,-14.1189429154851));
#28797=CARTESIAN_POINT('Ctrl Pts',(160.592444383487,13.6985795225324,-8.66806683595355));
#28798=CARTESIAN_POINT('Ctrl Pts',(160.71013820997,16.1696483168198,-1.15279526285827));
#28799=CARTESIAN_POINT('Ctrl Pts',(160.827832036453,14.7897374463801,6.6370271865379));
#28800=CARTESIAN_POINT('Ctrl Pts',(160.945525862937,9.88748786846115,12.8461685828396));
#28801=CARTESIAN_POINT('Ctrl Pts',(161.06321968942,2.63042426053809,15.9958535820154));
#28802=CARTESIAN_POINT('Ctrl Pts',(161.180913515903,-5.25310382814925,15.3359500448582));
#28803=CARTESIAN_POINT('Ctrl Pts',(161.298607342386,-11.8855474391451,11.0236212598008));
#28804=CARTESIAN_POINT('Ctrl Pts',(161.416301168869,-15.6873171483045,4.08589577647466));
#28805=CARTESIAN_POINT('Ctrl Pts',(161.533994995353,-15.752979667711,-3.82493074399836));
#28806=CARTESIAN_POINT('Ctrl Pts',(161.651688821836,-12.0668967458695,-10.8248079212624));
#28807=CARTESIAN_POINT('Ctrl Pts',(161.769382648319,-5.50694958937003,-15.2466379844161));
#28808=CARTESIAN_POINT('Ctrl Pts',(161.887076474802,2.3645382059743,-16.0373134495834));
#28809=CARTESIAN_POINT('Ctrl Pts',(162.004770301285,9.67288521004985,-13.0085262547648));
#28810=CARTESIAN_POINT('Ctrl Pts',(162.122464127768,14.67752816854,-6.88161539679513));
#28811=CARTESIAN_POINT('Ctrl Pts',(162.240157954252,16.1865562937323,0.884227887797634));
#28812=CARTESIAN_POINT('Ctrl Pts',(162.357851780735,13.840577933451,8.43948257156437));
#28813=CARTESIAN_POINT('Ctrl Pts',(162.475545607218,8.19831364750381,13.9847816194923));
#28814=CARTESIAN_POINT('Ctrl Pts',(162.593239433701,0.603530758605001,16.1994510472156));
#28815=CARTESIAN_POINT('Ctrl Pts',(162.710933260184,-7.13498962120933,14.5560429620394));
#28816=CARTESIAN_POINT('Ctrl Pts',(162.828627086668,-13.1742337149738,9.44595308222564));
#28817=CARTESIAN_POINT('Ctrl Pts',(162.946320913151,-16.0758890905255,2.08620554003872));
#28818=CARTESIAN_POINT('Ctrl Pts',(163.064014739634,-15.1488945929473,-5.77039480644631));
#28819=CARTESIAN_POINT('Ctrl Pts',(163.181708566117,-10.6140241611372,-12.2527121369471));
#28820=CARTESIAN_POINT('Ctrl Pts',(163.2994023926,-3.55130708784071,-15.8169112527338));
#28821=CARTESIAN_POINT('Ctrl Pts',(163.417096219084,4.35719284595873,-15.6141389170616));
#28822=CARTESIAN_POINT('Ctrl Pts',(163.534790045567,11.2279793567904,-11.692687592161));
#28823=CARTESIAN_POINT('Ctrl Pts',(163.65248387205,15.4246990473113,-4.9864940609672));
#28824=CARTESIAN_POINT('Ctrl Pts',(163.770177698533,15.9478569233932,2.90728790015858));
#28825=CARTESIAN_POINT('Ctrl Pts',(163.887871525016,12.672857226445,10.108667254542));
#28826=CARTESIAN_POINT('Ctrl Pts',(164.005565351499,6.37967707542191,14.902556282264));
#28827=CARTESIAN_POINT('Ctrl Pts',(164.123259177983,-1.43289323788845,16.1472375393268));
#28828=CARTESIAN_POINT('Ctrl Pts',(164.240953004466,-8.90420452717788,13.5462765378252));
#28829=CARTESIAN_POINT('Ctrl Pts',(164.358646830949,-14.2548809857467,7.71912065876858));
#28830=CARTESIAN_POINT('Ctrl Pts',(164.476340657432,-16.2106018116086,0.0535713981899616));
#28831=CARTESIAN_POINT('Ctrl Pts',(164.594034483915,-14.3055871426404,-7.62473676440622));
#28832=CARTESIAN_POINT('Ctrl Pts',(164.711728310399,-8.99354421585697,-13.4871293872258));
#28833=CARTESIAN_POINT('Ctrl Pts',(164.829422136882,-1.53958007844154,-16.1374149400877));
#28834=CARTESIAN_POINT('Ctrl Pts',(164.947115963365,6.2810321020304,-14.9443951095233));
#28835=CARTESIAN_POINT('Ctrl Pts',(165.064809789848,12.6057881822385,-10.1922081771534));
#28836=CARTESIAN_POINT('Ctrl Pts',(165.182503616331,15.9282533966172,-3.01262440261544));
#28837=CARTESIAN_POINT('Ctrl Pts',(165.300197442815,15.457401518827,4.88442784961914));
#28838=CARTESIAN_POINT('Ctrl Pts',(165.417891269298,11.3048471203361,11.6182432782841));
#28839=CARTESIAN_POINT('Ctrl Pts',(165.535585095781,4.46064461548986,15.5849549117565));
#28840=CARTESIAN_POINT('Ctrl Pts',(165.653278922264,-3.4474027167462,15.8401177026368));
#28841=CARTESIAN_POINT('Ctrl Pts',(165.731741473253,-8.16944088361523,13.4945278683989));
#28842=CARTESIAN_POINT('Ctrl Pts',(165.770972748747,-10.1138936307938,11.8324957226905));
#28843=CARTESIAN_POINT('Origin',(157.6,0.,0.));
#28844=CARTESIAN_POINT('Origin',(165.275,0.,0.));
#28845=CARTESIAN_POINT('Ctrl Pts',(68.2290272512527,-8.6315465241079,18.1146005753553));
#28846=CARTESIAN_POINT('Ctrl Pts',(68.2686455391672,-11.6377133328369,16.682172156035));
#28847=CARTESIAN_POINT('Ctrl Pts',(68.3478821149964,-16.920167839264,12.2933105870388));
#28848=CARTESIAN_POINT('Ctrl Pts',(68.4667369787402,-20.7364191237466,2.71910129728484));
#28849=CARTESIAN_POINT('Ctrl Pts',(68.5855918424838,-19.5178285413225,-7.51269261680735));
#28850=CARTESIAN_POINT('Ctrl Pts',(68.7044467062276,-13.560781282725,-15.9217739264575));
#28851=CARTESIAN_POINT('Ctrl Pts',(68.8233015699713,-4.3112850075781,-20.4646502512393));
#28852=CARTESIAN_POINT('Ctrl Pts',(68.9421564337151,5.98487983261901,-20.039336396671));
#28853=CARTESIAN_POINT('Ctrl Pts',(69.0610112974588,14.8280289192567,-14.7486055907437));
#28854=CARTESIAN_POINT('Ctrl Pts',(69.1798661612025,20.0711408256307,-5.87721609629587));
#28855=CARTESIAN_POINT('Ctrl Pts',(69.2987210249463,20.4412844203846,4.42111651613181));
#28856=CARTESIAN_POINT('Ctrl Pts',(69.4175758886899,15.8485849447886,13.6460461909995));
#28857=CARTESIAN_POINT('Ctrl Pts',(69.5364307524338,7.40808631971404,19.5579297437878));
#28858=CARTESIAN_POINT('Ctrl Pts',(69.6552856161775,-2.83098632764961,20.7214331897253));
#28859=CARTESIAN_POINT('Ctrl Pts',(69.7741404799212,-12.3827371735606,16.8540836193131));
#28860=CARTESIAN_POINT('Ctrl Pts',(69.892995343665,-18.928143773215,8.89481171599467));
#28861=CARTESIAN_POINT('Ctrl Pts',(70.0118502074086,-20.8780784123747,-1.22398747391038));
#28862=CARTESIAN_POINT('Ctrl Pts',(70.1307050711525,-17.7591261183169,-11.0456210793205));
#28863=CARTESIAN_POINT('Ctrl Pts',(70.2495599348961,-10.3285220474192,-18.1855419414053));
#28864=CARTESIAN_POINT('Ctrl Pts',(70.36841479864,-0.390306419466782,-20.9102837301104));
#28865=CARTESIAN_POINT('Ctrl Pts',(70.4872696623836,9.64266981062011,-18.5583195092622));
#28866=CARTESIAN_POINT('Ctrl Pts',(70.6061245261274,17.3345491904711,-11.7006712929421));
#28867=CARTESIAN_POINT('Ctrl Pts',(70.724979389871,20.8178577880174,-2.00227405925465));
#28868=CARTESIAN_POINT('Ctrl Pts',(70.843834253615,19.2469000686554,8.18224553636222));
#28869=CARTESIAN_POINT('Ctrl Pts',(70.9626891173585,13.0030812084345,16.3802375864514));
#28870=CARTESIAN_POINT('Ctrl Pts',(71.0815439811024,3.602307582272,20.6013515178363));
#28871=CARTESIAN_POINT('Ctrl Pts',(71.200398844846,-6.67305275956469,19.8207636371352));
#28872=CARTESIAN_POINT('Ctrl Pts',(71.3192537085899,-15.3282951176304,14.2279890734018));
#28873=CARTESIAN_POINT('Ctrl Pts',(71.4381085723335,-20.2620553480119,5.1808703285721));
#28874=CARTESIAN_POINT('Ctrl Pts',(71.5569634360773,-20.2764898302783,-5.12408669424093));
#28875=CARTESIAN_POINT('Ctrl Pts',(71.6758182998211,-15.3680940867467,-14.1849916611866));
#28876=CARTESIAN_POINT('Ctrl Pts',(71.7946731635647,-6.72855361766429,-19.8019915791725));
#28877=CARTESIAN_POINT('Ctrl Pts',(71.9135280273086,3.54457961832131,-20.6113623910834));
#28878=CARTESIAN_POINT('Ctrl Pts',(72.0323828910522,12.9571416297572,-16.416600898898));
#28879=CARTESIAN_POINT('Ctrl Pts',(72.151237754796,19.2239023220937,-8.2361328181285));
#28880=CARTESIAN_POINT('Ctrl Pts',(72.2700926185397,20.8233853839836,1.94394584218601));
#28881=CARTESIAN_POINT('Ctrl Pts',(72.3889474822834,17.3672601118087,11.6520633578796));
#28882=CARTESIAN_POINT('Ctrl Pts',(72.5078023460272,9.69462233016103,18.5312331527829));
#28883=CARTESIAN_POINT('Ctrl Pts',(72.6266572097709,-0.331725597276454,
20.9112950917769));
#28884=CARTESIAN_POINT('Ctrl Pts',(72.7455120735146,-10.2775354823501,18.2144055268431));
#28885=CARTESIAN_POINT('Ctrl Pts',(72.8643669372584,-17.7281125760169,11.0953291424513));
#28886=CARTESIAN_POINT('Ctrl Pts',(72.9832218010021,-20.8745675476636,1.28247182631354));
#28887=CARTESIAN_POINT('Ctrl Pts',(73.1020766647459,-18.9529879169663,-8.84175057930195));
#28888=CARTESIAN_POINT('Ctrl Pts',(73.2209315284896,-12.429904644976,-16.8193274183025));
#28889=CARTESIAN_POINT('Ctrl Pts',(73.3397863922333,-2.88902535394313,-20.7134216582276));
#28890=CARTESIAN_POINT('Ctrl Pts',(73.4586412559771,7.35326633413225,-19.5786051215753));
#28891=CARTESIAN_POINT('Ctrl Pts',(73.5774961197208,15.8102942970291,-13.6903943890812));
#28892=CARTESIAN_POINT('Ctrl Pts',(73.6963509834645,20.4288178986918,-4.47835947076039));
#28893=CARTESIAN_POINT('Ctrl Pts',(73.8152058472083,20.0875282846243,5.82095453526969));
#28894=CARTESIAN_POINT('Ctrl Pts',(73.934060710952,14.8692854982535,14.7070273358924));
#28895=CARTESIAN_POINT('Ctrl Pts',(74.0529155746958,6.04100129448752,20.0224525882135));
#28896=CARTESIAN_POINT('Ctrl Pts',(74.1717704384394,-4.25394819579815,20.4767240796648));
#28897=CARTESIAN_POINT('Ctrl Pts',(74.2906253021834,-13.5161023190106,15.9595514469955));
#28898=CARTESIAN_POINT('Ctrl Pts',(74.4094801659269,-19.4967477793413,7.56763703648682));
#28899=CARTESIAN_POINT('Ctrl Pts',(74.5283350296708,-20.7438727893319,-2.66158711810738));
#28900=CARTESIAN_POINT('Ctrl Pts',(74.6471898934143,-16.9546939409116,-12.2446174973853));
#28901=CARTESIAN_POINT('Ctrl Pts',(74.7660447571583,-9.04916751458383,-18.8548368218943));
#28902=CARTESIAN_POINT('Ctrl Pts',(74.8848996209018,1.05336222602103,-20.8873821315178));
#28903=CARTESIAN_POINT('Ctrl Pts',(75.0037544846458,10.9001512813116,-17.8487816483865));
#28904=CARTESIAN_POINT('Ctrl Pts',(75.1226093483893,18.1005456873079,-10.4767623867747));
#28905=CARTESIAN_POINT('Ctrl Pts',(75.2414642121331,20.9063967498254,-0.561141003802912));
#28906=CARTESIAN_POINT('Ctrl Pts',(75.3603190758769,18.6364855530042,9.4907170709027));
#28907=CARTESIAN_POINT('Ctrl Pts',(75.4791739396206,11.8419127825698,17.2383701647594));
#28908=CARTESIAN_POINT('Ctrl Pts',(75.5980288033644,2.1722996740317,20.8008033117344));
#28909=CARTESIAN_POINT('Ctrl Pts',(75.7168836671081,-8.02471549395103,19.3131107159981));
#28910=CARTESIAN_POINT('Ctrl Pts',(75.8357385308518,-16.2734490649882,13.1364820182761));
#28911=CARTESIAN_POINT('Ctrl Pts',(75.9545933945955,-20.5712311840959,3.77051082185677));
#28912=CARTESIAN_POINT('Ctrl Pts',(76.0734482583393,-19.8746242594179,-6.51088433580387));
#28913=CARTESIAN_POINT('Ctrl Pts',(76.192303122083,-14.352754093941,-15.2115335915258));
#28914=CARTESIAN_POINT('Ctrl Pts',(76.3111579858267,-5.34624865537712,-20.2190486819271));
#28915=CARTESIAN_POINT('Ctrl Pts',(76.4300128495705,4.95824645968282,-20.3176794032267));
#28916=CARTESIAN_POINT('Ctrl Pts',(76.5488677133142,14.0589530618911,-15.4834796829007));
#28917=CARTESIAN_POINT('Ctrl Pts',(76.667722577058,19.7463549128656,-6.8901213300209));
#28918=CARTESIAN_POINT('Ctrl Pts',(76.7865774408017,20.6396354130593,3.3760560278593));
#28919=CARTESIAN_POINT('Ctrl Pts',(76.9054323045454,16.5219193398244,12.8225771830625));
#28920=CARTESIAN_POINT('Ctrl Pts',(77.0242871682892,8.39292692660435,19.1559672658923));
#28921=CARTESIAN_POINT('Ctrl Pts',(77.1431420320329,-1.77374334422174,20.8385733397488));
#28922=CARTESIAN_POINT('Ctrl Pts',(77.2619968957766,-11.5097751060743,17.4618836697204));
#28923=CARTESIAN_POINT('Ctrl Pts',(77.3808517595204,-18.451404618894,9.84570829738103));
#28924=CARTESIAN_POINT('Ctrl Pts',(77.4997066232641,-20.9133074568072,-0.160858646988668));
#28925=CARTESIAN_POINT('Ctrl Pts',(77.6185614870079,-18.2977702184867,-10.1283715037868));
#28926=CARTESIAN_POINT('Ctrl Pts',(77.7374163507516,-11.2398064531836,-17.636866365152));
#28927=CARTESIAN_POINT('Ctrl Pts',(77.8562712144954,-1.45298481342087,-20.8633923276927));
#28928=CARTESIAN_POINT('Ctrl Pts',(77.975126078239,8.68659993361501,-19.0245968651264));
#28929=CARTESIAN_POINT('Ctrl Pts',(78.0939809419828,16.7172073837676,-12.5669121734563));
#28930=CARTESIAN_POINT('Ctrl Pts',(78.2128358057265,20.6891254607372,-3.05816807208725));
#28931=CARTESIAN_POINT('Ctrl Pts',(78.3316906694703,19.6380315166033,7.19305376319089));
#28932=CARTESIAN_POINT('Ctrl Pts',(78.450545533214,13.8191155315665,15.6979091032047));
#28933=CARTESIAN_POINT('Ctrl Pts',(78.5694003969578,4.6451237813503,20.3915455359125));
#28934=CARTESIAN_POINT('Ctrl Pts',(78.6882552607015,-5.65663495145375,20.1344179283447));
#28935=CARTESIAN_POINT('Ctrl Pts',(78.8071101244452,-14.5850468304206,14.9889530402125));
#28936=CARTESIAN_POINT('Ctrl Pts',(78.925964988189,-19.9724262140028,6.20439323491602));
#28937=CARTESIAN_POINT('Ctrl Pts',(79.0448198519327,-20.5107974964971,-4.08650099044958));
#28938=CARTESIAN_POINT('Ctrl Pts',(79.1636747156764,-16.0694521359249,-13.3852535403135));
#28939=CARTESIAN_POINT('Ctrl Pts',(79.2825295794202,-7.72668274442983,-19.4342655650835));
#28940=CARTESIAN_POINT('Ctrl Pts',(79.401384443164,2.49201032407988,-20.7649268920441));
#28941=CARTESIAN_POINT('Ctrl Pts',(79.5202393069076,12.1056803413097,-17.0541727375234));
#28942=CARTESIAN_POINT('Ctrl Pts',(79.6390941706514,18.7802711793142,-9.20291903249607));
#28943=CARTESIAN_POINT('Ctrl Pts',(79.7579490343951,20.8952914316842,0.882666569120876));
#28944=CARTESIAN_POINT('Ctrl Pts',(79.8768038981389,17.9372456308276,10.7539538527284));
#28945=CARTESIAN_POINT('Ctrl Pts',(79.9956587618826,10.6243033119855,18.014341048792));
#28946=CARTESIAN_POINT('Ctrl Pts',(80.1145136256262,0.731938129029032,20.9011141057727));
#28947=CARTESIAN_POINT('Ctrl Pts',(80.2333684893701,-9.33813074796676,18.7134074508395));
#28948=CARTESIAN_POINT('Ctrl Pts',(80.3522233531138,-17.1410403344121,11.982363729303));
#28949=CARTESIAN_POINT('Ctrl Pts',(80.4710782168576,-20.7823602095201,2.34218026825721));
#28950=CARTESIAN_POINT('Ctrl Pts',(80.5899330806012,-19.3780320528914,-7.86664973444038));
#28951=CARTESIAN_POINT('Ctrl Pts',(80.708787944345,-13.2690058590392,-16.1655741562136));
#28952=CARTESIAN_POINT('Ctrl Pts',(80.8276428080888,-3.93846234853991,-20.5397375498421));
#28953=CARTESIAN_POINT('Ctrl Pts',(80.9464976718324,6.34828125649317,-19.9271580857812));
#28954=CARTESIAN_POINT('Ctrl Pts',(81.0653525355762,15.0937565693877,-14.4765609490419));
#28955=CARTESIAN_POINT('Ctrl Pts',(81.1842073993199,20.1746922266295,-5.51127007576585));
#28956=CARTESIAN_POINT('Ctrl Pts',(81.3030622630637,20.3575126025494,4.7920752210601));
#28957=CARTESIAN_POINT('Ctrl Pts',(81.4219171268074,15.5978316283554,13.9319759108582));
#28958=CARTESIAN_POINT('Ctrl Pts',(81.5407719905512,7.05122906962834,19.6894000135831));
#28959=CARTESIAN_POINT('Ctrl Pts',(81.6596268542949,-3.20730705765452,20.6665305681718));
#28960=CARTESIAN_POINT('Ctrl Pts',(81.7784817180386,-12.6871567229822,16.6261348055928));
#28961=CARTESIAN_POINT('Ctrl Pts',(81.8973365817824,-19.0867533899846,8.54916073759119));
#28962=CARTESIAN_POINT('Ctrl Pts',(82.0161914455261,-20.8523701478954,-1.60342243417667));
#28963=CARTESIAN_POINT('Ctrl Pts',(82.1350463092699,-17.5553415020576,-11.3667184813117));
#28964=CARTESIAN_POINT('Ctrl Pts',(82.2539011730136,-9.99613698190578,-18.3703443006992));
#28965=CARTESIAN_POINT('Ctrl Pts',(82.3727560367574,-0.0100190419482207,
-20.9139236850969));
#28966=CARTESIAN_POINT('Ctrl Pts',(82.4916109005011,9.9785313724145,-18.3799133821952));
#28967=CARTESIAN_POINT('Ctrl Pts',(82.6104657642448,17.544442747166,-11.3835334136054));
#28968=CARTESIAN_POINT('Ctrl Pts',(82.7293206279886,20.8508243032301,-1.62340080174));
#28969=CARTESIAN_POINT('Ctrl Pts',(82.8481754917323,19.0949357636439,8.53086938533054));
#28970=CARTESIAN_POINT('Ctrl Pts',(82.9670303554759,12.7030807563111,16.6139713369771));
#28971=CARTESIAN_POINT('Ctrl Pts',(83.0858852192198,3.22710663214606,20.6634480925139));
#28972=CARTESIAN_POINT('Ctrl Pts',(83.2047400829634,-7.03236099624711,19.6961469101375));
#28973=CARTESIAN_POINT('Ctrl Pts',(83.3235949467073,-15.5844759437393,13.9469141334658));
#28974=CARTESIAN_POINT('Ctrl Pts',(83.4424498104509,-20.3529118683285,4.81157799139837));
#28975=CARTESIAN_POINT('Ctrl Pts',(83.5613046741947,-20.1799634326612,-5.49193774033512));
#28976=CARTESIAN_POINT('Ctrl Pts',(83.6801595379384,-15.1076199452285,-14.4620926520955));
#28977=CARTESIAN_POINT('Ctrl Pts',(83.7990144016822,-6.36737098063297,-19.9210665146787));
#28978=CARTESIAN_POINT('Ctrl Pts',(83.9178692654259,3.91878097726412,-20.5435016474673));
#28979=CARTESIAN_POINT('Ctrl Pts',(84.0367241291697,13.2535111849172,-16.1782800556342));
#28980=CARTESIAN_POINT('Ctrl Pts',(84.1555789929134,19.3704859523993,-7.88521263220971));
#28981=CARTESIAN_POINT('Ctrl Pts',(84.2744338566571,20.7845947636492,2.32226716769303));
#28982=CARTESIAN_POINT('Ctrl Pts',(84.3932887204008,17.152513026647,11.9659350306595));
#28983=CARTESIAN_POINT('Ctrl Pts',(84.5121435841446,9.3560561792281,18.7044517978578));
#28984=CARTESIAN_POINT('Ctrl Pts',(84.6309984478883,-0.711911986905901,
20.901805797829));
#28985=CARTESIAN_POINT('Ctrl Pts',(84.7498533116321,-10.6070385085257,18.0245121533403));
#28986=CARTESIAN_POINT('Ctrl Pts',(84.8687081753758,-17.9269338035892,10.7711349768254));
#28987=CARTESIAN_POINT('Ctrl Pts',(84.9875630391195,-20.8944361389867,0.902686391313687));
#28988=CARTESIAN_POINT('Ctrl Pts',(85.1064179028633,-18.7890800735068,-9.18492102734728));
#28989=CARTESIAN_POINT('Ctrl Pts',(85.225272766607,-12.122014753868,-17.0425661974441));
#28990=CARTESIAN_POINT('Ctrl Pts',(85.3441276303508,-2.51190450252216,-20.7625297123801));
#28991=CARTESIAN_POINT('Ctrl Pts',(85.4629824940945,7.70805881080918,-19.4416597454118));
#28992=CARTESIAN_POINT('Ctrl Pts',(85.5818373578382,16.0566200612769,-13.4006438835997));
#28993=CARTESIAN_POINT('Ctrl Pts',(85.700692221582,20.5068727177375,-4.10615095019311));
#28994=CARTESIAN_POINT('Ctrl Pts',(85.8195470853257,19.9783616090541,6.18525437675218));
#28995=CARTESIAN_POINT('Ctrl Pts',(85.9384019490693,14.5994013736218,14.9749719138016));
#28996=CARTESIAN_POINT('Ctrl Pts',(86.0572568128132,5.67592357316316,20.1289889432845));
#28997=CARTESIAN_POINT('Ctrl Pts',(86.1761116765568,-4.62558407166802,20.3959867690482));
#28998=CARTESIAN_POINT('Ctrl Pts',(86.2949665403008,-13.8040686848729,15.7111422891708));
#28999=CARTESIAN_POINT('Ctrl Pts',(86.4138214040442,-19.6311306835337,7.21186608120808));
#29000=CARTESIAN_POINT('Ctrl Pts',(86.5326762677881,-20.6920460609478,-3.03834397310024));
#29001=CARTESIAN_POINT('Ctrl Pts',(86.6515311315318,-16.7292403389556,-12.5508892899555));
#29002=CARTESIAN_POINT('Ctrl Pts',(86.7703859952756,-8.70482382118687,-19.0162653149707));
#29003=CARTESIAN_POINT('Ctrl Pts',(86.8892408590193,1.432994482384,-20.8647748873721));
#29004=CARTESIAN_POINT('Ctrl Pts',(87.0080957227631,11.2229030338076,-17.6476273697347));
#29005=CARTESIAN_POINT('Ctrl Pts',(87.1269505865067,18.2880576096475,-10.1458983413729));
#29006=CARTESIAN_POINT('Ctrl Pts',(87.2458054502506,20.9131437355076,-0.180896062030789));
#29007=CARTESIAN_POINT('Ctrl Pts',(87.3646603139942,18.460829534231,9.82802509130509));
#29008=CARTESIAN_POINT('Ctrl Pts',(87.4835151777381,11.5265004287498,17.4508478921023));
#29009=CARTESIAN_POINT('Ctrl Pts',(87.6023700414816,1.79370841459017,20.8368643132955));
#29010=CARTESIAN_POINT('Ctrl Pts',(87.7212249052256,-8.37456933075415,19.1639999168141));
#29011=CARTESIAN_POINT('Ctrl Pts',(87.8400797689691,-16.5096261697931,12.8384013031585));
#29012=CARTESIAN_POINT('Ctrl Pts',(87.958934632713,-20.636391267735,3.39582975606967));
#29013=CARTESIAN_POINT('Ctrl Pts',(88.0777894964567,-19.7529474224935,-6.87119876087563));
#29014=CARTESIAN_POINT('Ctrl Pts',(88.1966443602004,-14.0737816631622,-15.4700023912384));
#29015=CARTESIAN_POINT('Ctrl Pts',(88.3154992239441,-4.97771098870528,-20.312919475056));
#29016=CARTESIAN_POINT('Ctrl Pts',(88.4343540876879,5.32687389681903,-20.2241617570368));
#29017=CARTESIAN_POINT('Ctrl Pts',(88.5532089514316,14.3381730091277,-15.2252782912942));
#29018=CARTESIAN_POINT('Ctrl Pts',(88.6720638151754,19.868376918928,-6.52992365153576));
#29019=CARTESIAN_POINT('Ctrl Pts',(88.790918678919,20.5748343493,3.75079935297009));
#29020=CARTESIAN_POINT('Ctrl Pts',(88.9097735426629,16.2860279409612,13.1208840476639));
#29021=CARTESIAN_POINT('Ctrl Pts',(89.0286284064065,8.04321611663378,19.3054131992102));
#29022=CARTESIAN_POINT('Ctrl Pts',(89.1474832701505,-2.15236898069497,20.8028750909506));
#29023=CARTESIAN_POINT('Ctrl Pts',(89.2663381338938,-11.8253908946233,17.2497082436515));
#29024=CARTESIAN_POINT('Ctrl Pts',(89.3851929976379,-18.6273837390381,9.50856873082095));
#29025=CARTESIAN_POINT('Ctrl Pts',(89.5040478613814,-20.9069247951813,-0.541109877118889));
#29026=CARTESIAN_POINT('Ctrl Pts',(89.6229027251253,-18.1105753899303,-10.4594150595525));
#29027=CARTESIAN_POINT('Ctrl Pts',(89.7417575888689,-10.9172475795155,-17.8383297808979));
#29028=CARTESIAN_POINT('Ctrl Pts',(89.8606124526128,-1.07337439090547,-20.886363306994));
#29029=CARTESIAN_POINT('Ctrl Pts',(89.9794673163564,9.03109813531615,-18.8634983461956));
#29030=CARTESIAN_POINT('Ctrl Pts',(90.0983221801003,16.9429543312567,-12.2608565786884));
#29031=CARTESIAN_POINT('Ctrl Pts',(90.2171770438438,20.7413131374097,-2.68146095729082));
#29032=CARTESIAN_POINT('Ctrl Pts',(90.3360319075878,19.5039895591631,7.5489531352732));
#29033=CARTESIAN_POINT('Ctrl Pts',(90.4548867713314,13.531387277919,15.9465943979035));
#29034=CARTESIAN_POINT('Ctrl Pts',(90.5737416350752,4.2735654835411,20.4726382052112));
#29035=CARTESIAN_POINT('Ctrl Pts',(90.6925964988188,-6.021814680891,20.0282327411152));
#29036=CARTESIAN_POINT('Ctrl Pts',(90.8114513625627,-14.8551873562319,14.7212645520118));
#29037=CARTESIAN_POINT('Ctrl Pts',(90.9303062263063,-20.0819422730131,5.84020329677328));
#29038=CARTESIAN_POINT('Ctrl Pts',(91.0491610900501,-20.4330985674198,-4.45879423375491));
#29039=CARTESIAN_POINT('Ctrl Pts',(91.1680159537938,-15.8234056085072,-13.6752200512566));
#29040=CARTESIAN_POINT('Ctrl Pts',(91.2868708175377,-7.37201867707368,-19.5715898806077));
#29041=CARTESIAN_POINT('Ctrl Pts',(91.4057256812812,2.86917222790772,-20.7161033751214));
#29042=CARTESIAN_POINT('Ctrl Pts',(91.5245805450251,12.4137954244847,-16.8313801312361));
#29043=CARTESIAN_POINT('Ctrl Pts',(91.6434354087687,18.9444853649975,-8.85960809395612));
#29044=CARTESIAN_POINT('Ctrl Pts',(91.7622902725126,20.8758294198323,1.26187795552705));
#29045=CARTESIAN_POINT('Ctrl Pts',(91.8811451362562,17.7386656817295,11.0795895560304));
#29046=CARTESIAN_POINT('Ctrl Pts',(91.9603817120854,12.7761628790883,15.8272202722995));
#29047=CARTESIAN_POINT('Ctrl Pts',(92.,9.87756200380534,17.4664283201656));
#29048=CARTESIAN_POINT('Ctrl Pts',(68.3943515008351,-8.75472251862488,18.3731039542012));
#29049=CARTESIAN_POINT('Ctrl Pts',(68.4339697887497,-11.8037886600882,16.9202341464656));
#29050=CARTESIAN_POINT('Ctrl Pts',(68.5132063645789,-17.1616261335772,12.4687415776771));
#29051=CARTESIAN_POINT('Ctrl Pts',(68.6320612283225,-21.0323370153035,2.75790407793953));
#29052=CARTESIAN_POINT('Ctrl Pts',(68.7509160920664,-19.7963566051723,-7.61990207017598));
#29053=CARTESIAN_POINT('Ctrl Pts',(68.86977095581,-13.7542996419509,-16.1489846971332));
#29054=CARTESIAN_POINT('Ctrl Pts',(68.9886258195538,-4.37280895545597,-20.7566898805338));
#29055=CARTESIAN_POINT('Ctrl Pts',(69.1074806832975,6.07028672041002,-20.325306608756));
#29056=CARTESIAN_POINT('Ctrl Pts',(69.2263355470413,15.0396314639171,-14.9590747293047));
#29057=CARTESIAN_POINT('Ctrl Pts',(69.345190410785,20.3575649010131,-5.96108657485157));
#29058=CARTESIAN_POINT('Ctrl Pts',(69.4640452745288,20.7329906089168,4.48420780831553));
#29059=CARTESIAN_POINT('Ctrl Pts',(69.5829001382724,16.0747512762576,13.840781318257));
#29060=CARTESIAN_POINT('Ctrl Pts',(69.7017550020163,7.51380299486025,19.8370300695702));
#29061=CARTESIAN_POINT('Ctrl Pts',(69.8206098657599,-2.8713857572765,21.0171372253617));
#29062=CARTESIAN_POINT('Ctrl Pts',(69.9394647295037,-12.5594443212236,17.0945988625182));
#29063=CARTESIAN_POINT('Ctrl Pts',(70.0583195932474,-19.1982567740677,9.02174462148259));
#29064=CARTESIAN_POINT('Ctrl Pts',(70.1771744569911,-21.1760178447656,-1.24145431765083));
#29065=CARTESIAN_POINT('Ctrl Pts',(70.2960293207349,-18.0125567191098,-11.2032469876909));
#29066=CARTESIAN_POINT('Ctrl Pts',(70.4148841844786,-10.4759146347763,-18.4450576849868));
#29067=CARTESIAN_POINT('Ctrl Pts',(70.5337390482224,-0.395876265061667,
-21.2086827466592));
#29068=CARTESIAN_POINT('Ctrl Pts',(70.6525939119661,9.78027498257911,-18.8231549539572));
#29069=CARTESIAN_POINT('Ctrl Pts',(70.7714487757098,17.5819208903253,-11.867645058188));
#29070=CARTESIAN_POINT('Ctrl Pts',(70.8903036394535,21.1149378454081,-2.03084739751513));
#29071=CARTESIAN_POINT('Ctrl Pts',(71.0091585031973,19.5215618631211,8.29900980664779));
#29072=CARTESIAN_POINT('Ctrl Pts',(71.128013366941,13.1886409404201,16.6139908367525));
#29073=CARTESIAN_POINT('Ctrl Pts',(71.2468682306848,3.65371410806238,20.895341934793));
#29074=CARTESIAN_POINT('Ctrl Pts',(71.3657230944285,-6.76828018003073,20.1036147190673));
#29075=CARTESIAN_POINT('Ctrl Pts',(71.4845779581723,-15.5470366826663,14.4310287835161));
#29076=CARTESIAN_POINT('Ctrl Pts',(71.603432821916,-20.5512038582445,5.25480364439256));
#29077=CARTESIAN_POINT('Ctrl Pts',(71.7222876856597,-20.5658443269705,-5.19720968243216));
#29078=CARTESIAN_POINT('Ctrl Pts',(71.8411425494035,-15.5874036007114,-14.3874177791715));
#29079=CARTESIAN_POINT('Ctrl Pts',(71.9599974131472,-6.82457305997421,-20.0845747755174));
#29080=CARTESIAN_POINT('Ctrl Pts',(72.078852276891,3.59516234048029,-20.9054956676383));
#29081=CARTESIAN_POINT('Ctrl Pts',(72.1977071406347,13.1420457835939,-16.6508730697845));
#29082=CARTESIAN_POINT('Ctrl Pts',(72.3165620043785,19.4982359285231,-8.35366608380849));
#29083=CARTESIAN_POINT('Ctrl Pts',(72.4354168681221,21.1205443226187,1.97168681093702));
#29084=CARTESIAN_POINT('Ctrl Pts',(72.5542717318659,17.6150986110084,11.8183434663484));
#29085=CARTESIAN_POINT('Ctrl Pts',(72.6731265956096,9.83296888759997,18.7956820631658));
#29086=CARTESIAN_POINT('Ctrl Pts',(72.7919814593534,-0.336459468574833,
21.2097085409049));
#29087=CARTESIAN_POINT('Ctrl Pts',(72.9108363230971,-10.4242004688258,18.4743331665816));
#29088=CARTESIAN_POINT('Ctrl Pts',(73.0296911868409,-17.9811005998156,11.2536644069138));
#29089=CARTESIAN_POINT('Ctrl Pts',(73.1485460505845,-21.172456878459,1.30077326768389));
#29090=CARTESIAN_POINT('Ctrl Pts',(73.2674009143283,-19.2234554547616,-8.96792627885183));
#29091=CARTESIAN_POINT('Ctrl Pts',(73.386255778072,-12.6072848933614,-17.0593466751147));
#29092=CARTESIAN_POINT('Ctrl Pts',(73.5051106418158,-2.93025302619897,-21.0090113657587));
#29093=CARTESIAN_POINT('Ctrl Pts',(73.6239655055595,7.45820070378722,-19.8580004941624));
#29094=CARTESIAN_POINT('Ctrl Pts',(73.7428203693033,16.0359142039836,-13.8857623847811));
#29095=CARTESIAN_POINT('Ctrl Pts',(73.8616752330469,20.720346184434,-4.54226764527755));
#29096=CARTESIAN_POINT('Ctrl Pts',(73.9805300967909,20.3741862163097,5.90402213641362));
#29097=CARTESIAN_POINT('Ctrl Pts',(74.0993849605344,15.0814767925817,14.9169031343287));
#29098=CARTESIAN_POINT('Ctrl Pts',(74.2182398242783,6.12720906041322,20.3081818608687));
#29099=CARTESIAN_POINT('Ctrl Pts',(74.3370946880219,-4.31465392195945,20.7689360078422));
#29100=CARTESIAN_POINT('Ctrl Pts',(74.4559495517657,-13.7089830896219,16.1873013196328));
#29101=CARTESIAN_POINT('Ctrl Pts',(74.5748044155094,-19.7749750113744,7.67563057107641));
#29102=CARTESIAN_POINT('Ctrl Pts',(74.6936592792532,-21.0398970480001,-2.69956914593409));
#29103=CARTESIAN_POINT('Ctrl Pts',(74.8125141429968,-17.1966449379978,-12.4193536160528));
#29104=CARTESIAN_POINT('Ctrl Pts',(74.9313690067407,-9.17830314573018,-19.123903700061));
#29105=CARTESIAN_POINT('Ctrl Pts',(75.0502238704843,1.06839417185068,-21.1854543321044));
#29106=CARTESIAN_POINT('Ctrl Pts',(75.1690787342282,11.0557012711902,-18.10349167333));
#29107=CARTESIAN_POINT('Ctrl Pts',(75.2879335979718,18.358848496672,-10.6262704294766));
#29108=CARTESIAN_POINT('Ctrl Pts',(75.4067884617156,21.2047402974427,-0.569148734632473));
#29109=CARTESIAN_POINT('Ctrl Pts',(75.5256433254594,18.9024364617877,9.62615380991842));
#29110=CARTESIAN_POINT('Ctrl Pts',(75.644498189203,12.0109021264727,17.484369347289));
#29111=CARTESIAN_POINT('Ctrl Pts',(75.7633530529468,2.2032993531727,21.0976399941897));
#29112=CARTESIAN_POINT('Ctrl Pts',(75.8822079166905,-8.13923174071195,19.5887173657469));
#29113=CARTESIAN_POINT('Ctrl Pts',(76.0010627804342,-16.505678395758,13.3239454389432));
#29114=CARTESIAN_POINT('Ctrl Pts',(76.119917644178,-20.8647917705404,3.824317682426));
#29115=CARTESIAN_POINT('Ctrl Pts',(76.2387725079218,-20.1582439563016,-6.60379754098762));
#29116=CARTESIAN_POINT('Ctrl Pts',(76.3576273716655,-14.557574256196,-15.4286089178339));
#29117=CARTESIAN_POINT('Ctrl Pts',(76.4764822354091,-5.42254199321897,-20.5075834679736));
#29118=CARTESIAN_POINT('Ctrl Pts',(76.595337099153,5.02900283422426,-20.6076216933806));
#29119=CARTESIAN_POINT('Ctrl Pts',(76.7141919628966,14.2595805532021,-15.704435800463));
#29120=CARTESIAN_POINT('Ctrl Pts',(76.8330468266405,20.0281441493233,-6.98844641519513));
#29121=CARTESIAN_POINT('Ctrl Pts',(76.9519016903841,20.9341721581688,3.42423384369045));
#29122=CARTESIAN_POINT('Ctrl Pts',(77.0707565541279,16.7576944515415,13.0055610426041));
#29123=CARTESIAN_POINT('Ctrl Pts',(77.1896114178716,8.51269771370555,19.42933140896));
#29124=CARTESIAN_POINT('Ctrl Pts',(77.3084662816154,-1.79905544789076,21.1359490172441));
#29125=CARTESIAN_POINT('Ctrl Pts',(77.427321145359,-11.6740246981257,17.71107248903));
#29126=CARTESIAN_POINT('Ctrl Pts',(77.5461760091029,-18.7147143407172,9.98621091853553));
#29127=CARTESIAN_POINT('Ctrl Pts',(77.6650308728465,-21.2117496232761,-0.163154171175886));
#29128=CARTESIAN_POINT('Ctrl Pts',(77.7838857365904,-18.5588875093233,-10.2729078541768));
#29129=CARTESIAN_POINT('Ctrl Pts',(77.902740600334,-11.4002034729046,-17.88855226508));
#29130=CARTESIAN_POINT('Ctrl Pts',(78.0215954640778,-1.47371955069089,-21.1611221831461));
#29131=CARTESIAN_POINT('Ctrl Pts',(78.1404503278215,8.81056156468606,-19.29608629435));
#29132=CARTESIAN_POINT('Ctrl Pts',(78.2593051915654,16.955769342426,-12.7462475799967));
#29133=CARTESIAN_POINT('Ctrl Pts',(78.3781600553089,20.9843684507617,-3.10180948589734));
#29134=CARTESIAN_POINT('Ctrl Pts',(78.4970149190528,19.918274930186,7.29570182845017));
#29135=CARTESIAN_POINT('Ctrl Pts',(78.6158697827964,14.0163204350206,15.9219252236326));
#29136=CARTESIAN_POINT('Ctrl Pts',(78.7347246465403,4.71141175649178,20.6825419285183));
#29137=CARTESIAN_POINT('Ctrl Pts',(78.8535795102839,-5.73735763930797,20.4217449960281));
#29138=CARTESIAN_POINT('Ctrl Pts',(78.9724343740277,-14.7931819129804,15.2028520434027));
#29139=CARTESIAN_POINT('Ctrl Pts',(79.0912892377714,-20.2574415881256,6.29293267624914));
#29140=CARTESIAN_POINT('Ctrl Pts',(79.2101441015152,-20.8034956674346,-4.14481717077568));
#29141=CARTESIAN_POINT('Ctrl Pts',(79.3289989652588,-16.2987703401028,-13.5762670408589));
#29142=CARTESIAN_POINT('Ctrl Pts',(79.4478538290027,-7.83694593176299,-19.7116011482261));
#29143=CARTESIAN_POINT('Ctrl Pts',(79.5667086927464,2.5275724158971,-21.0612516020896));
#29144=CARTESIAN_POINT('Ctrl Pts',(79.6855635564901,12.2784337651812,-17.2975433411275));
#29145=CARTESIAN_POINT('Ctrl Pts',(79.8044184202338,19.0482739727128,-9.33424876594779));
#29146=CARTESIAN_POINT('Ctrl Pts',(79.9232732839776,21.1934765014896,0.895262612271957));
#29147=CARTESIAN_POINT('Ctrl Pts',(80.0421281477213,18.193218076009,10.9074175405044));
#29148=CARTESIAN_POINT('Ctrl Pts',(80.1609830114651,10.7759168290822,18.2714136797575));
#29149=CARTESIAN_POINT('Ctrl Pts',(80.2798378752087,0.742383210535154,21.1993822677181));
#29150=CARTESIAN_POINT('Ctrl Pts',(80.3986927389525,-9.47139001252587,18.9804560691979));
#29151=CARTESIAN_POINT('Ctrl Pts',(80.5175476026963,-17.3856505771247,12.1533573704655));
#29152=CARTESIAN_POINT('Ctrl Pts',(80.63640246644,-21.0789337007326,2.37560421877118));
#29153=CARTESIAN_POINT('Ctrl Pts',(80.7552573301837,-19.6545651588917,-7.9789103127562));
#29154=CARTESIAN_POINT('Ctrl Pts',(80.8741121939275,-13.4583604536502,-16.3962640642236));
#29155=CARTESIAN_POINT('Ctrl Pts',(80.9929670576711,-3.99466595183329,-20.8328487081673));
#29156=CARTESIAN_POINT('Ctrl Pts',(81.111821921415,6.43887404366729,-20.2115274636509));
#29157=CARTESIAN_POINT('Ctrl Pts',(81.2306767851586,15.3091511653896,-14.683147889992));
#29158=CARTESIAN_POINT('Ctrl Pts',(81.3495316489025,20.4625940263995,-5.58991834241638));
#29159=CARTESIAN_POINT('Ctrl Pts',(81.4683865126461,20.6480233301123,4.86046025837706));
#29160=CARTESIAN_POINT('Ctrl Pts',(81.5872413763899,15.8204195988616,14.130791381946));
#29161=CARTESIAN_POINT('Ctrl Pts',(81.7060962401336,7.15185323365191,19.9703764783849));
#29162=CARTESIAN_POINT('Ctrl Pts',(81.8249511038774,-3.25307675088904,20.961451119065));
#29163=CARTESIAN_POINT('Ctrl Pts',(81.943805967621,-12.8682080725383,16.8633971181961));
#29164=CARTESIAN_POINT('Ctrl Pts',(82.0626608313649,-19.3591298203665,8.67116105042012));
#29165=CARTESIAN_POINT('Ctrl Pts',(82.1815156951086,-21.1499427119579,-1.62630398297084));
#29166=CARTESIAN_POINT('Ctrl Pts',(82.3003705588523,-17.8058640060564,-11.5289265919231));
#29167=CARTESIAN_POINT('Ctrl Pts',(82.4192254225961,-10.1387862870605,-18.6324972558549));
#29168=CARTESIAN_POINT('Ctrl Pts',(82.5380802863397,-0.010162018117406,
-21.2123746454166));
#29169=CARTESIAN_POINT('Ctrl Pts',(82.6569351500835,10.1209294377187,-18.6422028923849));
#29170=CARTESIAN_POINT('Ctrl Pts',(82.7757900138273,17.794809721102,-11.5459814807533));
#29171=CARTESIAN_POINT('Ctrl Pts',(82.8946448775709,21.148374807404,-1.64656745069401));
#29172=CARTESIAN_POINT('Ctrl Pts',(83.0134997413148,19.3674289601245,8.6526086724557));
#29173=CARTESIAN_POINT('Ctrl Pts',(83.1323546050585,12.8843593488806,16.8510600714922));
#29174=CARTESIAN_POINT('Ctrl Pts',(83.2512094688022,3.27315887408406,20.9583246551133));
#29175=CARTESIAN_POINT('Ctrl Pts',(83.370064332546,-7.13271590450091,19.9772196561435));
#29176=CARTESIAN_POINT('Ctrl Pts',(83.4889191962896,-15.8068733227066,14.1459427796111));
#29177=CARTESIAN_POINT('Ctrl Pts',(83.6077740600334,-20.643356941375,4.880241341892));
#29178=CARTESIAN_POINT('Ctrl Pts',(83.7266289237771,-20.4679404548775,-5.57031012599066));
#29179=CARTESIAN_POINT('Ctrl Pts',(83.8454837875209,-15.323212377748,-14.6684731240356));
#29180=CARTESIAN_POINT('Ctrl Pts',(83.9643386512646,-6.45823618663142,-20.2053489631288));
#29181=CARTESIAN_POINT('Ctrl Pts',(84.0831935150084,3.9747037186663,-20.836666521134));
#29182=CARTESIAN_POINT('Ctrl Pts',(84.202048378752,13.4426446636611,-16.4091512824603));
#29183=CARTESIAN_POINT('Ctrl Pts',(84.3209032424958,19.646911372201,-7.99773811130408));
#29184=CARTESIAN_POINT('Ctrl Pts',(84.4397581062396,21.0812001429395,2.35540694943616));
#29185=CARTESIAN_POINT('Ctrl Pts',(84.5586129699833,17.3972869897626,12.136694227011));
#29186=CARTESIAN_POINT('Ctrl Pts',(84.677467833727,9.48957124763614,18.9713726150788));
#29187=CARTESIAN_POINT('Ctrl Pts',(84.7963226974708,-0.722071286488033,
21.2000838305266));
#29188=CARTESIAN_POINT('Ctrl Pts',(84.9151775612145,-10.7584056492251,18.2817299304756));
#29189=CARTESIAN_POINT('Ctrl Pts',(85.0340324249582,-18.1827590944255,10.9248438468571));
#29190=CARTESIAN_POINT('Ctrl Pts',(85.1528872887019,-21.1926090033863,0.91556812620056));
#29191=CARTESIAN_POINT('Ctrl Pts',(85.2717421524458,-19.0572085737298,-9.31599392128854));
#29192=CARTESIAN_POINT('Ctrl Pts',(85.3905970161894,-12.2950012770463,-17.2857711705771));
#29193=CARTESIAN_POINT('Ctrl Pts',(85.5094518799332,-2.54775049308316,-21.0588202136093));
#29194=CARTESIAN_POINT('Ctrl Pts',(85.6283067436769,7.81805622635515,-19.7191008467849));
#29195=CARTESIAN_POINT('Ctrl Pts',(85.7471616074207,16.2857551460622,-13.591877011165));
#29196=CARTESIAN_POINT('Ctrl Pts',(85.8660164711643,20.7995148803425,-4.16474754415393));
#29197=CARTESIAN_POINT('Ctrl Pts',(85.9848713349081,20.2634616838949,6.27352069809667));
#29198=CARTESIAN_POINT('Ctrl Pts',(86.1037261986518,14.8077413018752,15.1886714001213));
#29199=CARTESIAN_POINT('Ctrl Pts',(86.2225810623957,5.75692151819817,20.4162385369449));
#29200=CARTESIAN_POINT('Ctrl Pts',(86.3414359261392,-4.691593206492,20.6870465400193));
#29201=CARTESIAN_POINT('Ctrl Pts',(86.4602907898831,-14.0010588631557,15.9353472530277));
#29202=CARTESIAN_POINT('Ctrl Pts',(86.5791456536268,-19.9112756191699,7.31478260658337));
#29203=CARTESIAN_POINT('Ctrl Pts',(86.6980005173706,-20.9873307292317,-3.08170248823144));
#29204=CARTESIAN_POINT('Ctrl Pts',(86.8168553811143,-16.9679740132177,-12.7299960428468));
#29205=CARTESIAN_POINT('Ctrl Pts',(86.9357102448579,-8.8290455152107,-19.2876358492809));
#29206=CARTESIAN_POINT('Ctrl Pts',(87.0545651086018,1.45344394877011,-21.1625244725649));
#29207=CARTESIAN_POINT('Ctrl Pts',(87.1734199723454,11.3830588342422,-17.8994668339676));
#29208=CARTESIAN_POINT('Ctrl Pts',(87.2922748360893,18.5490362972512,-10.2906848075035));
#29209=CARTESIAN_POINT('Ctrl Pts',(87.4111296998329,21.211583565601,-0.183477529011579));
#29210=CARTESIAN_POINT('Ctrl Pts',(87.5299845635768,18.7242737537734,9.96827536527145));
#29211=CARTESIAN_POINT('Ctrl Pts',(87.6488394273203,11.6909886985687,17.699879225974));
#29212=CARTESIAN_POINT('Ctrl Pts',(87.7676942910643,1.81930542866218,21.1342156022259));
#29213=CARTESIAN_POINT('Ctrl Pts',(87.8865491548078,-8.49407814682619,19.4374786893705));
#29214=CARTESIAN_POINT('Ctrl Pts',(88.0054040185517,-16.7452258525253,13.0216109799074));
#29215=CARTESIAN_POINT('Ctrl Pts',(88.1242588822953,-20.9308817174528,3.44428975176641));
#29216=CARTESIAN_POINT('Ctrl Pts',(88.2431137460392,-20.0348307369856,-6.96925381260139));
#29217=CARTESIAN_POINT('Ctrl Pts',(88.3619686097828,-14.2746207651856,-15.6907661818753));
#29218=CARTESIAN_POINT('Ctrl Pts',(88.4808234735266,-5.04874513070288,-20.6027938389252));
#29219=CARTESIAN_POINT('Ctrl Pts',(88.5996783372703,5.40289074826908,-20.5127695089313));
#29220=CARTESIAN_POINT('Ctrl Pts',(88.7185332010141,14.5427850928398,-15.44254976056));
#29221=CARTESIAN_POINT('Ctrl Pts',(88.8373880647577,20.151907463494,-6.62310855619352));
#29222=CARTESIAN_POINT('Ctrl Pts',(88.9562429285016,20.8684463545089,3.80432492214186));
#29223=CARTESIAN_POINT('Ctrl Pts',(89.0750977922453,16.5184367778662,13.3081248783771));
#29224=CARTESIAN_POINT('Ctrl Pts',(89.1939526559889,8.15799637548015,19.5809100019827));
#29225=CARTESIAN_POINT('Ctrl Pts',(89.3128075197329,-2.18308424000846,21.0997413386136));
#29226=CARTESIAN_POINT('Ctrl Pts',(89.4316623834764,-11.9941444638625,17.495869225592));
#29227=CARTESIAN_POINT('Ctrl Pts',(89.5505172472203,-18.8932047609022,9.64426022093586));
#29228=CARTESIAN_POINT('Ctrl Pts',(89.6693721109639,-21.2052758782399,-0.548831754892572));
#29229=CARTESIAN_POINT('Ctrl Pts',(89.7882269747077,-18.3690213275962,-10.6086755482063));
#29230=CARTESIAN_POINT('Ctrl Pts',(89.9070818384514,-11.0730415411467,-18.09289065306));
#29231=CARTESIAN_POINT('Ctrl Pts',(90.0259367021953,-1.08869191919774,-21.1844209685031));
#29232=CARTESIAN_POINT('Ctrl Pts',(90.1447915659388,9.15997590841173,-19.132688828153));
#29233=CARTESIAN_POINT('Ctrl Pts',(90.2636464296828,17.1847377989099,-12.4358244362435));
#29234=CARTESIAN_POINT('Ctrl Pts',(90.3825012934262,21.0373008687106,-2.71972659361109));
#29235=CARTESIAN_POINT('Ctrl Pts',(90.5013561571702,19.7823201346039,7.6566800423115));
#29236=CARTESIAN_POINT('Ctrl Pts',(90.6202110209137,13.7244861716685,16.1741593677076));
#29237=CARTESIAN_POINT('Ctrl Pts',(90.7390658846577,4.33455115709318,20.7647918261493));
#29238=CARTESIAN_POINT('Ctrl Pts',(90.8579207484012,-6.10774864533687,20.3140444991141));
#29239=CARTESIAN_POINT('Ctrl Pts',(90.9767756121453,-15.067177463825,14.9313435218322));
#29240=CARTESIAN_POINT('Ctrl Pts',(91.0956304758887,-20.368520489837,5.92354558627522));
#29241=CARTESIAN_POINT('Ctrl Pts',(91.2144853396326,-20.7246879402021,-4.5224232036684));
#29242=CARTESIAN_POINT('Ctrl Pts',(91.3333402033763,-16.0492126196877,-13.8703715024302));
#29243=CARTESIAN_POINT('Ctrl Pts',(91.45219506712,-7.47722065097378,-19.8508851425969));
#29244=CARTESIAN_POINT('Ctrl Pts',(91.5710499308638,2.91011658725582,-21.0117313519411));
#29245=CARTESIAN_POINT('Ctrl Pts',(91.6899047946075,12.5909457871538,-17.0715713856038));
#29246=CARTESIAN_POINT('Ctrl Pts',(91.8087596583513,19.2148315676077,-8.98603862815482));
#29247=CARTESIAN_POINT('Ctrl Pts',(91.9276145220949,21.1737367581028,1.27988551323374));
#29248=CARTESIAN_POINT('Ctrl Pts',(92.0464693858387,17.9918043030239,11.2377002096187));
#29249=CARTESIAN_POINT('Ctrl Pts',(92.1257059616679,12.9584843859408,16.0530817204229));
#29250=CARTESIAN_POINT('Ctrl Pts',(92.1653242495824,10.0185191914685,17.7156819936512));
#29251=CARTESIAN_POINT('Ctrl Pts',(68.5596757504176,-8.87789851314185,18.6316073330471));
#29252=CARTESIAN_POINT('Ctrl Pts',(68.5992940383321,-11.9698639873395,17.1582961368962));
#29253=CARTESIAN_POINT('Ctrl Pts',(68.6785306141613,-17.4030844278904,12.6441725683155));
#29254=CARTESIAN_POINT('Ctrl Pts',(68.797385477905,-21.3282549068603,2.79670685859421));
#29255=CARTESIAN_POINT('Ctrl Pts',(68.9162403416488,-20.0748846690222,-7.72711152354461));
#29256=CARTESIAN_POINT('Ctrl Pts',(69.0350952053924,-13.9478180011767,-16.376195467809));
#29257=CARTESIAN_POINT('Ctrl Pts',(69.1539500691362,-4.43433290333388,-21.0487295098283));
#29258=CARTESIAN_POINT('Ctrl Pts',(69.27280493288,6.15569360820102,-20.611276820841));
#29259=CARTESIAN_POINT('Ctrl Pts',(69.3916597966237,15.2512340085775,-15.1695438678658));
#29260=CARTESIAN_POINT('Ctrl Pts',(69.5105146603674,20.6439889763955,-6.04495705340727));
#29261=CARTESIAN_POINT('Ctrl Pts',(69.6293695241112,21.024696797449,4.54729910049925));
#29262=CARTESIAN_POINT('Ctrl Pts',(69.7482243878549,16.3009176077266,14.0355164455145));
#29263=CARTESIAN_POINT('Ctrl Pts',(69.8670792515987,7.6195196700065,20.1161303953526));
#29264=CARTESIAN_POINT('Ctrl Pts',(69.9859341153423,-2.91178518690343,21.312841260998));
#29265=CARTESIAN_POINT('Ctrl Pts',(70.1047889790862,-12.7361514688866,17.3351141057232));
#29266=CARTESIAN_POINT('Ctrl Pts',(70.2236438428299,-19.4683697749204,9.1486775269705));
#29267=CARTESIAN_POINT('Ctrl Pts',(70.3424987065736,-21.4739572771565,-1.25892116139127));
#29268=CARTESIAN_POINT('Ctrl Pts',(70.4613535703174,-18.2659873199027,-11.3608728960612));
#29269=CARTESIAN_POINT('Ctrl Pts',(70.580208434061,-10.6233072221335,-18.7045734285684));
#29270=CARTESIAN_POINT('Ctrl Pts',(70.6990632978048,-0.401446110656565,
-21.507081763208));
#29271=CARTESIAN_POINT('Ctrl Pts',(70.8179181615486,9.91788015453811,-19.0879903986521));
#29272=CARTESIAN_POINT('Ctrl Pts',(70.9367730252922,17.8292925901796,-12.0346188234338));
#29273=CARTESIAN_POINT('Ctrl Pts',(71.055627889036,21.4120179027988,-2.05942073577562));
#29274=CARTESIAN_POINT('Ctrl Pts',(71.1744827527798,19.7962236575869,8.41577407693337));
#29275=CARTESIAN_POINT('Ctrl Pts',(71.2933376165234,13.3742006724056,16.8477440870536));
#29276=CARTESIAN_POINT('Ctrl Pts',(71.4121924802673,3.70512063385281,21.1893323517497));
#29277=CARTESIAN_POINT('Ctrl Pts',(71.531047344011,-6.86350760049681,20.3864658009993));
#29278=CARTESIAN_POINT('Ctrl Pts',(71.6499022077547,-15.7657782477023,14.6340684936305));
#29279=CARTESIAN_POINT('Ctrl Pts',(71.7687570714985,-20.8403523684772,5.32873696021297));
#29280=CARTESIAN_POINT('Ctrl Pts',(71.8876119352421,-20.8551988236627,-5.27033267062336));
#29281=CARTESIAN_POINT('Ctrl Pts',(72.006466798986,-15.8067131146762,-14.5898438971565));
#29282=CARTESIAN_POINT('Ctrl Pts',(72.1253216627296,-6.92059250228412,-20.3671579718622));
#29283=CARTESIAN_POINT('Ctrl Pts',(72.2441765264734,3.64574506263926,-21.1996289441932));
#29284=CARTESIAN_POINT('Ctrl Pts',(72.3630313902172,13.3269499374307,-16.8851452406709));
#29285=CARTESIAN_POINT('Ctrl Pts',(72.4818862539608,19.7725695349525,-8.47119934948849));
#29286=CARTESIAN_POINT('Ctrl Pts',(72.6007411177046,21.4177032612537,1.99942777968804));
#29287=CARTESIAN_POINT('Ctrl Pts',(72.7195959814483,17.8629371102081,11.9846235748171));
#29288=CARTESIAN_POINT('Ctrl Pts',(72.8384508451921,9.97131544503892,19.0601309735488));
#29289=CARTESIAN_POINT('Ctrl Pts',(72.9573057089358,-0.341193339873213,
21.5081219900329));
#29290=CARTESIAN_POINT('Ctrl Pts',(73.0761605726795,-10.5708654553014,18.7342608063202));
#29291=CARTESIAN_POINT('Ctrl Pts',(73.1950154364233,-18.2340886236142,11.4119996713763));
#29292=CARTESIAN_POINT('Ctrl Pts',(73.313870300167,-21.4703462092543,1.31907470905424));
#29293=CARTESIAN_POINT('Ctrl Pts',(73.4327251639108,-19.4939229925569,-9.0941019784017));
#29294=CARTESIAN_POINT('Ctrl Pts',(73.5515800276545,-12.7846651417468,-17.2993659319269));
#29295=CARTESIAN_POINT('Ctrl Pts',(73.6704348913983,-2.97148069845482,-21.3046010732898));
#29296=CARTESIAN_POINT('Ctrl Pts',(73.7892897551418,7.56313507344221,-20.1373958667494));
#29297=CARTESIAN_POINT('Ctrl Pts',(73.9081446188858,16.2615341109381,-14.081130380481));
#29298=CARTESIAN_POINT('Ctrl Pts',(74.0269994826293,21.0118744701763,-4.60617581979471));
#29299=CARTESIAN_POINT('Ctrl Pts',(74.1458543463733,20.6608441479951,5.98708973755754));
#29300=CARTESIAN_POINT('Ctrl Pts',(74.2647092101168,15.2936680869099,15.1267789327649));
#29301=CARTESIAN_POINT('Ctrl Pts',(74.3835640738608,6.21341682633891,20.5939111335238));
#29302=CARTESIAN_POINT('Ctrl Pts',(74.5024189376042,-4.37535964812074,21.0611479360197));
#29303=CARTESIAN_POINT('Ctrl Pts',(74.6212738013482,-13.9018638602333,16.4150511922701));
#29304=CARTESIAN_POINT('Ctrl Pts',(74.7401286650918,-20.0532022434075,7.78362410566604));
#29305=CARTESIAN_POINT('Ctrl Pts',(74.8589835288356,-21.3359213066685,-2.73755117376083));
#29306=CARTESIAN_POINT('Ctrl Pts',(74.9778383925793,-17.4385959350839,-12.5940897347202));
#29307=CARTESIAN_POINT('Ctrl Pts',(75.0966932563231,-9.30743877687657,-19.3929705782277));
#29308=CARTESIAN_POINT('Ctrl Pts',(75.2155481200667,1.08342611768035,-21.483526532691));
#29309=CARTESIAN_POINT('Ctrl Pts',(75.3344029838106,11.2112512610687,-18.3582016982736));
#29310=CARTESIAN_POINT('Ctrl Pts',(75.4532578475542,18.6171513060362,-10.7757784721784));
#29311=CARTESIAN_POINT('Ctrl Pts',(75.5721127112981,21.5030838450601,-0.577156465462027));
#29312=CARTESIAN_POINT('Ctrl Pts',(75.6909675750417,19.1683873705711,9.76159054893414));
#29313=CARTESIAN_POINT('Ctrl Pts',(75.8098224387856,12.1798914703757,17.7303685298185));
#29314=CARTESIAN_POINT('Ctrl Pts',(75.9286773025292,2.23429903231371,21.3944766766451));
#29315=CARTESIAN_POINT('Ctrl Pts',(76.047532166273,-8.25374798747288,19.8643240154957));
#29316=CARTESIAN_POINT('Ctrl Pts',(76.1663870300167,-16.7379077265277,13.5114088596102));
#29317=CARTESIAN_POINT('Ctrl Pts',(76.2852418937604,-21.1583523569849,3.87812454299523));
#29318=CARTESIAN_POINT('Ctrl Pts',(76.4040967575042,-20.4418636531854,-6.69671074617139));
#29319=CARTESIAN_POINT('Ctrl Pts',(76.5229516212479,-14.762394418451,-15.6456842441421));
#29320=CARTESIAN_POINT('Ctrl Pts',(76.6418064849916,-5.49883533106082,-20.7961182540201));
#29321=CARTESIAN_POINT('Ctrl Pts',(76.7606613487354,5.09975920876569,-20.8975639835345));
#29322=CARTESIAN_POINT('Ctrl Pts',(76.8795162124791,14.4602080445132,-15.9253919180253));
#29323=CARTESIAN_POINT('Ctrl Pts',(76.9983710762229,20.309933385781,-7.08677150036936));
#29324=CARTESIAN_POINT('Ctrl Pts',(77.1172259399665,21.2287089032783,3.4724116595216));
#29325=CARTESIAN_POINT('Ctrl Pts',(77.2360808037104,16.9934695632586,13.1885449021457));
#29326=CARTESIAN_POINT('Ctrl Pts',(77.354935667454,8.63246850080676,19.7026955520276));
#29327=CARTESIAN_POINT('Ctrl Pts',(77.4737905311979,-1.82436755155978,21.4333246947394));
#29328=CARTESIAN_POINT('Ctrl Pts',(77.5926453949414,-11.8382742901771,17.9602613083396));
#29329=CARTESIAN_POINT('Ctrl Pts',(77.7115002586854,-18.9780240625405,10.1267135396901));
#29330=CARTESIAN_POINT('Ctrl Pts',(77.830355122429,-21.510191789745,-0.165449695363124));
#29331=CARTESIAN_POINT('Ctrl Pts',(77.9492099861728,-18.82000480016,-10.4174442045669));
#29332=CARTESIAN_POINT('Ctrl Pts',(78.0680648499164,-11.5606004926255,-18.1402381650081));
#29333=CARTESIAN_POINT('Ctrl Pts',(78.1869197136603,-1.49445428796093,-21.4588520385995));
#29334=CARTESIAN_POINT('Ctrl Pts',(78.3057745774039,8.93452319575713,-19.5675757235736));
#29335=CARTESIAN_POINT('Ctrl Pts',(78.4246294411477,17.1943313010844,-12.9255829865371));
#29336=CARTESIAN_POINT('Ctrl Pts',(78.5434843048914,21.2796114407862,-3.14545089970743));
#29337=CARTESIAN_POINT('Ctrl Pts',(78.6623391686352,20.1985183437687,7.39834989370943));
#29338=CARTESIAN_POINT('Ctrl Pts',(78.7811940323789,14.2135253384747,16.1459413440607));
#29339=CARTESIAN_POINT('Ctrl Pts',(78.9000488961227,4.77769973163326,20.9735383211241));
#29340=CARTESIAN_POINT('Ctrl Pts',(79.0189037598663,-5.8180803271622,20.7090720637115));
#29341=CARTESIAN_POINT('Ctrl Pts',(79.1377586236102,-15.0013169955402,15.416751046593));
#29342=CARTESIAN_POINT('Ctrl Pts',(79.2566134873538,-20.5424569622484,6.38147211758228));
#29343=CARTESIAN_POINT('Ctrl Pts',(79.3754683510977,-21.096193838372,-4.2031333511018));
#29344=CARTESIAN_POINT('Ctrl Pts',(79.4943232148413,-16.5280885442806,-13.7672805414043));
#29345=CARTESIAN_POINT('Ctrl Pts',(79.6131780785851,-7.94720911909616,-19.9889367313688));
#29346=CARTESIAN_POINT('Ctrl Pts',(79.7320329423288,2.56313450771434,-21.357576312135));
#29347=CARTESIAN_POINT('Ctrl Pts',(79.8508878060726,12.4511871890527,-17.5409139447316));
#29348=CARTESIAN_POINT('Ctrl Pts',(79.9697426698162,19.3162767661114,-9.46557849939951));
#29349=CARTESIAN_POINT('Ctrl Pts',(80.08859753356,21.4916615712951,0.907858655423031));
#29350=CARTESIAN_POINT('Ctrl Pts',(80.2074523973037,18.4491905211904,11.0608812282804));
#29351=CARTESIAN_POINT('Ctrl Pts',(80.3263072610476,10.9275303461789,18.528486310723));
#29352=CARTESIAN_POINT('Ctrl Pts',(80.4451621247911,0.752828292041289,21.4976504296635));
#29353=CARTESIAN_POINT('Ctrl Pts',(80.5640169885351,-9.60464927708498,19.2475046875563));
#29354=CARTESIAN_POINT('Ctrl Pts',(80.6828718522786,-17.6302608198373,12.3243510116281));
#29355=CARTESIAN_POINT('Ctrl Pts',(80.8017267160225,-21.3755071919452,2.40902816928516));
#29356=CARTESIAN_POINT('Ctrl Pts',(80.9205815797661,-19.9310982648919,-8.09117089107204));
#29357=CARTESIAN_POINT('Ctrl Pts',(81.03943644351,-13.6477150482613,-16.6269539722335));
#29358=CARTESIAN_POINT('Ctrl Pts',(81.1582913072536,-4.05086955512668,-21.1259598664926));
#29359=CARTESIAN_POINT('Ctrl Pts',(81.2771461709974,6.5294668308414,-20.4958968415206));
#29360=CARTESIAN_POINT('Ctrl Pts',(81.3960010347411,15.5245457613914,-14.8897348309422));
#29361=CARTESIAN_POINT('Ctrl Pts',(81.5148558984849,20.7504958261696,-5.66856660906691));
#29362=CARTESIAN_POINT('Ctrl Pts',(81.6337107622285,20.9385340576752,4.92884529569403));
#29363=CARTESIAN_POINT('Ctrl Pts',(81.7525656259724,16.0430075693679,14.3296068530338));
#29364=CARTESIAN_POINT('Ctrl Pts',(81.8714204897161,7.25247739767545,20.2513529431867));
#29365=CARTESIAN_POINT('Ctrl Pts',(81.9902753534598,-3.29884644412353,21.2563716699582));
#29366=CARTESIAN_POINT('Ctrl Pts',(82.1091302172035,-13.0492594220944,17.1006594307994));
#29367=CARTESIAN_POINT('Ctrl Pts',(82.2279850809474,-19.6315062507484,8.79316136324904));
#29368=CARTESIAN_POINT('Ctrl Pts',(82.3468399446909,-21.4475152760204,-1.64918553176499));
#29369=CARTESIAN_POINT('Ctrl Pts',(82.4656948084348,-18.0563865100551,-11.6911347025345));
#29370=CARTESIAN_POINT('Ctrl Pts',(82.5845496721784,-10.2814355922152,-18.8946502110105));
#29371=CARTESIAN_POINT('Ctrl Pts',(82.7034045359223,-0.0103049942866093,
-21.5108256057363));
#29372=CARTESIAN_POINT('Ctrl Pts',(82.8222593996658,10.2633275030229,-18.9044924025747));
#29373=CARTESIAN_POINT('Ctrl Pts',(82.9411142634098,18.045176695038,-11.7084295479012));
#29374=CARTESIAN_POINT('Ctrl Pts',(83.0599691271533,21.445925311578,-1.66973409964801));
#29375=CARTESIAN_POINT('Ctrl Pts',(83.1788239908973,19.6399221566051,8.77434795958085));
#29376=CARTESIAN_POINT('Ctrl Pts',(83.2976788546409,13.0656379414501,17.0881488060073));
#29377=CARTESIAN_POINT('Ctrl Pts',(83.4165337183847,3.31921111602204,21.2532012177127));
#29378=CARTESIAN_POINT('Ctrl Pts',(83.5353885821283,-7.23307081275469,20.2582924021494));
#29379=CARTESIAN_POINT('Ctrl Pts',(83.6542434458721,-16.029270701674,14.3449714257563));
#29380=CARTESIAN_POINT('Ctrl Pts',(83.7730983096159,-20.9338020144214,4.94890469238559));
#29381=CARTESIAN_POINT('Ctrl Pts',(83.8919531733596,-20.7559174770939,-5.64868251164617));
#29382=CARTESIAN_POINT('Ctrl Pts',(84.0108080371033,-15.5388048102676,-14.8748535959758));
#29383=CARTESIAN_POINT('Ctrl Pts',(84.1296629008471,-6.54910139262988,-20.489631411579));
#29384=CARTESIAN_POINT('Ctrl Pts',(84.2485177645907,4.0306264600685,-21.1298313948007));
#29385=CARTESIAN_POINT('Ctrl Pts',(84.3673726283346,13.6317781424049,-16.6400225092864));
#29386=CARTESIAN_POINT('Ctrl Pts',(84.4862274920783,19.9233367920027,-8.11026359039845));
#29387=CARTESIAN_POINT('Ctrl Pts',(84.6050823558219,21.3778055222299,2.38854673117928));
#29388=CARTESIAN_POINT('Ctrl Pts',(84.7239372195658,17.6420609528783,12.3074534233625));
#29389=CARTESIAN_POINT('Ctrl Pts',(84.8427920833094,9.62308631604418,19.2382934322998));
#29390=CARTESIAN_POINT('Ctrl Pts',(84.9616469470533,-0.732230586070165,
21.4983618632242));
#29391=CARTESIAN_POINT('Ctrl Pts',(85.080501810797,-10.9097727899244,18.538947707611));
#29392=CARTESIAN_POINT('Ctrl Pts',(85.1993566745406,-18.4385843852619,11.0785527168889));
#29393=CARTESIAN_POINT('Ctrl Pts',(85.3182115382845,-21.4907818677859,0.92844986108743));
#29394=CARTESIAN_POINT('Ctrl Pts',(85.4370664020281,-19.3253370739528,-9.44706681522981));
#29395=CARTESIAN_POINT('Ctrl Pts',(85.555921265772,-12.4679878002247,-17.5289761437101));
#29396=CARTESIAN_POINT('Ctrl Pts',(85.6747761295156,-2.58359648364417,-21.3551107148385));
#29397=CARTESIAN_POINT('Ctrl Pts',(85.7936309932594,7.92805364190112,-19.9965419481581));
#29398=CARTESIAN_POINT('Ctrl Pts',(85.9124858570031,16.5148902308474,-13.7831101387303));
#29399=CARTESIAN_POINT('Ctrl Pts',(86.0313407207469,21.0921570429475,-4.22334413811475));
#29400=CARTESIAN_POINT('Ctrl Pts',(86.1501955844906,20.5485617587358,6.36178701944117));
#29401=CARTESIAN_POINT('Ctrl Pts',(86.2690504482343,15.0160812301286,15.402370886441));
#29402=CARTESIAN_POINT('Ctrl Pts',(86.3879053119781,5.83791946323322,20.7034881306052));
#29403=CARTESIAN_POINT('Ctrl Pts',(86.5067601757217,-4.75760234131602,20.9781063109904));
#29404=CARTESIAN_POINT('Ctrl Pts',(86.6256150394656,-14.1980490414384,16.1595522168846));
#29405=CARTESIAN_POINT('Ctrl Pts',(86.7444699032092,-20.1914205548062,7.41769913195866));
#29406=CARTESIAN_POINT('Ctrl Pts',(86.8633247669531,-21.2826153975157,-3.12506100336263));
#29407=CARTESIAN_POINT('Ctrl Pts',(86.9821796306967,-17.2067076874798,-12.9091027957381));
#29408=CARTESIAN_POINT('Ctrl Pts',(87.1010344944405,-8.95326720923453,-19.559006383591));
#29409=CARTESIAN_POINT('Ctrl Pts',(87.2198893581841,1.47389341515622,-21.4602740577577));
#29410=CARTESIAN_POINT('Ctrl Pts',(87.338744221928,11.5432146346768,-18.1513062982005));
#29411=CARTESIAN_POINT('Ctrl Pts',(87.4575990856716,18.810014984855,-10.435471273634));
#29412=CARTESIAN_POINT('Ctrl Pts',(87.5764539494155,21.5100233956944,-0.186058995992359));
#29413=CARTESIAN_POINT('Ctrl Pts',(87.6953088131591,18.9877179733158,10.1085256392378));
#29414=CARTESIAN_POINT('Ctrl Pts',(87.814163676903,11.8554769683876,17.9489105598457));
#29415=CARTESIAN_POINT('Ctrl Pts',(87.9330185406465,1.84490244273418,21.4315668911563));
#29416=CARTESIAN_POINT('Ctrl Pts',(88.0518734043905,-8.61358696289824,19.710957461927));
#29417=CARTESIAN_POINT('Ctrl Pts',(88.1707282681339,-16.9808255352575,13.2048206566564));
#29418=CARTESIAN_POINT('Ctrl Pts',(88.289583131878,-21.2253721671706,3.49274974746314));
#29419=CARTESIAN_POINT('Ctrl Pts',(88.4084379956215,-20.3167140514776,-7.06730886432714));
#29420=CARTESIAN_POINT('Ctrl Pts',(88.5272928593654,-14.475459867209,-15.9115299725123));
#29421=CARTESIAN_POINT('Ctrl Pts',(88.646147723109,-5.11977927270044,-20.8926682027945));
#29422=CARTESIAN_POINT('Ctrl Pts',(88.7650025868529,5.4789075997191,-20.8013772608259));
#29423=CARTESIAN_POINT('Ctrl Pts',(88.8838574505964,14.7473971765519,-15.6598212298257));
#29424=CARTESIAN_POINT('Ctrl Pts',(89.0027123143403,20.4354380080601,-6.71629346085131));
#29425=CARTESIAN_POINT('Ctrl Pts',(89.121567178084,21.1620583597178,3.85785049131365));
#29426=CARTESIAN_POINT('Ctrl Pts',(89.2404220418277,16.7508456147713,13.4953657090902));
#29427=CARTESIAN_POINT('Ctrl Pts',(89.3592769055715,8.27277663432653,19.8564068047553));
#29428=CARTESIAN_POINT('Ctrl Pts',(89.4781317693152,-2.21379949932195,21.3966075862766));
#29429=CARTESIAN_POINT('Ctrl Pts',(89.596986633059,-12.1628980331017,17.7420302075325));
#29430=CARTESIAN_POINT('Ctrl Pts',(89.7158414968027,-19.1590257827662,9.77995171105074));
#29431=CARTESIAN_POINT('Ctrl Pts',(89.8346963605465,-21.5036269612985,-0.556553632666229));
#29432=CARTESIAN_POINT('Ctrl Pts',(89.9535512242901,-18.627467265262,-10.7579360368601));
#29433=CARTESIAN_POINT('Ctrl Pts',(90.072406088034,-11.228835502778,-18.347451525222));
#29434=CARTESIAN_POINT('Ctrl Pts',(90.1912609517776,-1.10400944748999,-21.4824786300121));
#29435=CARTESIAN_POINT('Ctrl Pts',(90.3101158155213,9.28885368150731,-19.4018793101104));
#29436=CARTESIAN_POINT('Ctrl Pts',(90.4289706792652,17.426521266563,-12.6107922937986));
#29437=CARTESIAN_POINT('Ctrl Pts',(90.5478255430088,21.3332886000114,-2.75799222993136));
#29438=CARTESIAN_POINT('Ctrl Pts',(90.6666804067526,20.0606507100447,7.76440694934979));
#29439=CARTESIAN_POINT('Ctrl Pts',(90.7855352704963,13.917585065418,16.4017243375116));
#29440=CARTESIAN_POINT('Ctrl Pts',(90.90439013424,4.39553683064526,21.0569454470874));
#29441=CARTESIAN_POINT('Ctrl Pts',(91.0232449979838,-6.19368260978275,20.5998562571131));
#29442=CARTESIAN_POINT('Ctrl Pts',(91.1420998617275,-15.279167571418,15.1414224916527));
#29443=CARTESIAN_POINT('Ctrl Pts',(91.2609547254712,-20.6550987066608,6.00688787577717));
#29444=CARTESIAN_POINT('Ctrl Pts',(91.3798095892151,-21.0162773129844,-4.58605217358187));
#29445=CARTESIAN_POINT('Ctrl Pts',(91.4986644529586,-16.2750196308681,-14.0655229536038));
#29446=CARTESIAN_POINT('Ctrl Pts',(91.6175193167026,-7.58242262487387,-20.1301804045861));
#29447=CARTESIAN_POINT('Ctrl Pts',(91.7363741804461,2.95106094660392,-21.3073593287609));
#29448=CARTESIAN_POINT('Ctrl Pts',(91.85522904419,12.768096149823,-17.3117626399715));
#29449=CARTESIAN_POINT('Ctrl Pts',(91.9740839079336,19.4851777702179,-9.11246916235354));
#29450=CARTESIAN_POINT('Ctrl Pts',(92.0929387716774,21.4716440963733,1.29789307094044));
#29451=CARTESIAN_POINT('Ctrl Pts',(92.2117936354211,18.2449429243184,11.3958108632069));
#29452=CARTESIAN_POINT('Ctrl Pts',(92.2910302112503,13.1408058927933,16.2789431685464));
#29453=CARTESIAN_POINT('Ctrl Pts',(92.3306484991649,10.1594763791317,17.9649356671368));
#29454=CARTESIAN_POINT('Ctrl Pts',(68.725,-9.00107450765883,18.890110711893));
#29455=CARTESIAN_POINT('Ctrl Pts',(68.7646182879146,-12.1359393145907,17.3963581273268));
#29456=CARTESIAN_POINT('Ctrl Pts',(68.8438548637437,-17.6445427222035,12.8196035589538));
#29457=CARTESIAN_POINT('Ctrl Pts',(68.9627097274875,-21.6241727984171,2.8355096392489));
#29458=CARTESIAN_POINT('Ctrl Pts',(69.0815645912312,-20.353412732872,-7.83432097691324));
#29459=CARTESIAN_POINT('Ctrl Pts',(69.2004194549749,-14.1413363604027,-16.6034062384847));
#29460=CARTESIAN_POINT('Ctrl Pts',(69.3192743187187,-4.49585685121175,-21.3407691391228));
#29461=CARTESIAN_POINT('Ctrl Pts',(69.4381291824624,6.24110049599202,-20.897247032926));
#29462=CARTESIAN_POINT('Ctrl Pts',(69.5569840462062,15.4628365532379,-15.3800130064269));
#29463=CARTESIAN_POINT('Ctrl Pts',(69.6758389099499,20.9304130517779,-6.12882753196297));
#29464=CARTESIAN_POINT('Ctrl Pts',(69.7946937736936,21.3164029859812,4.61039039268297));
#29465=CARTESIAN_POINT('Ctrl Pts',(69.9135486374374,16.5270839391956,14.2302515727719));
#29466=CARTESIAN_POINT('Ctrl Pts',(70.0324035011811,7.72523634515273,20.395230721135));
#29467=CARTESIAN_POINT('Ctrl Pts',(70.1512583649248,-2.95218461653034,21.6085452966344));
#29468=CARTESIAN_POINT('Ctrl Pts',(70.2701132286686,-12.9128586165496,17.5756293489283));
#29469=CARTESIAN_POINT('Ctrl Pts',(70.3889680924123,-19.7384827757731,9.27561043245846));
#29470=CARTESIAN_POINT('Ctrl Pts',(70.507822956156,-21.7718967095473,-1.27638800513175));
#29471=CARTESIAN_POINT('Ctrl Pts',(70.6266778198999,-18.5194179206956,-11.5184988044314));
#29472=CARTESIAN_POINT('Ctrl Pts',(70.7455326836434,-10.7706998094906,-18.96408917215));
#29473=CARTESIAN_POINT('Ctrl Pts',(70.8643875473874,-0.40701595625145,-21.8054807797568));
#29474=CARTESIAN_POINT('Ctrl Pts',(70.9832424111309,10.0554853264971,-19.3528258433471));
#29475=CARTESIAN_POINT('Ctrl Pts',(71.1020972748748,18.0766642900339,-12.2015925886796));
#29476=CARTESIAN_POINT('Ctrl Pts',(71.2209521386185,21.7090979601895,-2.08799407403611));
#29477=CARTESIAN_POINT('Ctrl Pts',(71.3398070023622,20.0708854520526,8.53253834721895));
#29478=CARTESIAN_POINT('Ctrl Pts',(71.458661866106,13.5597604043912,17.0814973373548));
#29479=CARTESIAN_POINT('Ctrl Pts',(71.5775167298496,3.75652715964321,21.4833227687064));
#29480=CARTESIAN_POINT('Ctrl Pts',(71.6963715935935,-6.95873502096286,20.6693168829313));
#29481=CARTESIAN_POINT('Ctrl Pts',(71.8152264573371,-15.9845198127382,14.8371082037448));
#29482=CARTESIAN_POINT('Ctrl Pts',(71.934081321081,-21.1295008787099,5.40267027603342));
#29483=CARTESIAN_POINT('Ctrl Pts',(72.0529361848246,-21.1445533203548,-5.34345565881458));
#29484=CARTESIAN_POINT('Ctrl Pts',(72.1717910485684,-16.0260226286409,-14.7922700151415));
#29485=CARTESIAN_POINT('Ctrl Pts',(72.290645912312,-7.01661194459403,-20.6497411682071));
#29486=CARTESIAN_POINT('Ctrl Pts',(72.4095007760559,3.69632778479824,-21.4937622207481));
#29487=CARTESIAN_POINT('Ctrl Pts',(72.5283556397995,13.5118540912674,-17.1194174115574));
#29488=CARTESIAN_POINT('Ctrl Pts',(72.6472105035433,20.0469031413818,-8.58873261516847));
#29489=CARTESIAN_POINT('Ctrl Pts',(72.766065367287,21.7148621998888,2.02716874843905));
#29490=CARTESIAN_POINT('Ctrl Pts',(72.8849202310308,18.1107756094078,12.1509036832859));
#29491=CARTESIAN_POINT('Ctrl Pts',(73.0037750947745,10.1096620024779,19.3245798839318));
#29492=CARTESIAN_POINT('Ctrl Pts',(73.1226299585183,-0.345927211171586,
21.8065354391609));
#29493=CARTESIAN_POINT('Ctrl Pts',(73.2414848222619,-10.717530441777,18.9941884460587));
#29494=CARTESIAN_POINT('Ctrl Pts',(73.3603396860058,-18.4870766474128,11.5703349358388));
#29495=CARTESIAN_POINT('Ctrl Pts',(73.4791945497494,-21.7682355400497,1.33737615042459));
#29496=CARTESIAN_POINT('Ctrl Pts',(73.5980494134933,-19.7643905303522,-9.22027767795157));
#29497=CARTESIAN_POINT('Ctrl Pts',(73.7169042772369,-12.9620453901322,-17.5393851887391));
#29498=CARTESIAN_POINT('Ctrl Pts',(73.8357591409807,-3.01270837071065,-21.6001907808208));
#29499=CARTESIAN_POINT('Ctrl Pts',(73.9546140047244,7.66806944309719,-20.4167912393365));
#29500=CARTESIAN_POINT('Ctrl Pts',(74.0734688684682,16.4871540178927,-14.2764983761808));
#29501=CARTESIAN_POINT('Ctrl Pts',(74.1923237322118,21.3034027559186,-4.67008399431189));
#29502=CARTESIAN_POINT('Ctrl Pts',(74.3111785959557,20.9475020796805,6.07015733870148));
#29503=CARTESIAN_POINT('Ctrl Pts',(74.4300334596993,15.5058593812382,15.3366547312012));
#29504=CARTESIAN_POINT('Ctrl Pts',(74.5488883234433,6.29962459226462,20.879640406179));
#29505=CARTESIAN_POINT('Ctrl Pts',(74.6677431871866,-4.43606537428203,21.3533598641971));
#29506=CARTESIAN_POINT('Ctrl Pts',(74.7865980509307,-14.0947446308446,16.6428010649075));
#29507=CARTESIAN_POINT('Ctrl Pts',(74.9054529146743,-20.3314294754405,7.89161764025565));
#29508=CARTESIAN_POINT('Ctrl Pts',(75.0243077784181,-21.6319455653368,-2.77553320158754));
#29509=CARTESIAN_POINT('Ctrl Pts',(75.1431626421617,-17.68054693217,-12.7688258533877));
#29510=CARTESIAN_POINT('Ctrl Pts',(75.2620175059056,-9.43657440802294,-19.6620374563944));
#29511=CARTESIAN_POINT('Ctrl Pts',(75.3808723696492,1.09845806351002,-21.7815987332776));
#29512=CARTESIAN_POINT('Ctrl Pts',(75.4997272333931,11.3668012509472,-18.6129117232171));
#29513=CARTESIAN_POINT('Ctrl Pts',(75.6185820971367,18.8754541154003,-10.9252865148803));
#29514=CARTESIAN_POINT('Ctrl Pts',(75.7374369608804,21.8014273926774,-0.585164196291588));
#29515=CARTESIAN_POINT('Ctrl Pts',(75.8562918246243,19.4343382793545,9.89702728794988));
#29516=CARTESIAN_POINT('Ctrl Pts',(75.9751466883679,12.3488808142786,17.976367712348));
#29517=CARTESIAN_POINT('Ctrl Pts',(76.0940015521117,2.26529871145472,21.6913133591005));
#29518=CARTESIAN_POINT('Ctrl Pts',(76.2128564158553,-8.36826423423381,20.1399306652444));
#29519=CARTESIAN_POINT('Ctrl Pts',(76.3317112795992,-16.9701370572975,13.6988722802772));
#29520=CARTESIAN_POINT('Ctrl Pts',(76.4505661433428,-21.4519129434293,3.93193140356445));
#29521=CARTESIAN_POINT('Ctrl Pts',(76.5694210070867,-20.7254833500691,-6.78962395135514));
#29522=CARTESIAN_POINT('Ctrl Pts',(76.6882758708304,-14.967214580706,-15.8627595704502));
#29523=CARTESIAN_POINT('Ctrl Pts',(76.807130734574,-5.57512866890268,-21.0846530400666));
#29524=CARTESIAN_POINT('Ctrl Pts',(76.9259855983179,5.17051558330714,-21.1875062736884));
#29525=CARTESIAN_POINT('Ctrl Pts',(77.0448404620615,14.6608355358242,-16.1463480355876));
#29526=CARTESIAN_POINT('Ctrl Pts',(77.1636953258054,20.5917226222387,-7.1850965855436));
#29527=CARTESIAN_POINT('Ctrl Pts',(77.2825501895489,21.5232456483878,3.52058947535276));
#29528=CARTESIAN_POINT('Ctrl Pts',(77.4014050532929,17.2292446749756,13.3715287616874));
#29529=CARTESIAN_POINT('Ctrl Pts',(77.5202599170364,8.75223928790795,19.9760596950952));
#29530=CARTESIAN_POINT('Ctrl Pts',(77.6391147807804,-1.8496796552288,21.7307003722347));
#29531=CARTESIAN_POINT('Ctrl Pts',(77.7579696445239,-12.0025238822286,18.2094501276491));
#29532=CARTESIAN_POINT('Ctrl Pts',(77.8768245082678,-19.2413337843638,10.2672161608446));
#29533=CARTESIAN_POINT('Ctrl Pts',(77.9956793720115,-21.8086339562139,-0.167745219550351));
#29534=CARTESIAN_POINT('Ctrl Pts',(78.1145342357552,-19.0811220909967,-10.5619805549569));
#29535=CARTESIAN_POINT('Ctrl Pts',(78.2333890994989,-11.7209975123465,-18.3919240649361));
#29536=CARTESIAN_POINT('Ctrl Pts',(78.3522439632427,-1.51518902523096,-21.7565818940529));
#29537=CARTESIAN_POINT('Ctrl Pts',(78.4710988269864,9.05848482682818,-19.8390651527972));
#29538=CARTESIAN_POINT('Ctrl Pts',(78.5899536907302,17.4328932597428,-13.1049183930775));
#29539=CARTESIAN_POINT('Ctrl Pts',(78.7088085544739,21.5748544308107,-3.18909231351752));
#29540=CARTESIAN_POINT('Ctrl Pts',(78.8276634182175,20.4787617573513,7.5009979589687));
#29541=CARTESIAN_POINT('Ctrl Pts',(78.9465182819614,14.4107302419287,16.3699574644887));
#29542=CARTESIAN_POINT('Ctrl Pts',(79.0653731457051,4.84398770677473,21.2645347137299));
#29543=CARTESIAN_POINT('Ctrl Pts',(79.1842280094488,-5.89880301501642,20.9963991313949));
#29544=CARTESIAN_POINT('Ctrl Pts',(79.3030828731926,-15.2094520781,15.6306500497832));
#29545=CARTESIAN_POINT('Ctrl Pts',(79.4219377369363,-20.8274723363712,6.47001155891541));
#29546=CARTESIAN_POINT('Ctrl Pts',(79.54079260068,-21.3888920093095,-4.26144953142791));
#29547=CARTESIAN_POINT('Ctrl Pts',(79.6596474644238,-16.7574067484584,-13.9582940419497));
#29548=CARTESIAN_POINT('Ctrl Pts',(79.7785023281675,-8.05747230642932,-20.2662723145114));
#29549=CARTESIAN_POINT('Ctrl Pts',(79.8973571919112,2.59869659953155,-21.6539010221805));
#29550=CARTESIAN_POINT('Ctrl Pts',(80.0162120556551,12.6239406129242,-17.7842845483357));
#29551=CARTESIAN_POINT('Ctrl Pts',(80.1350669193986,19.58427955951,-9.59690823285125));
#29552=CARTESIAN_POINT('Ctrl Pts',(80.2539217831425,21.7898466411006,0.920454698574115));
#29553=CARTESIAN_POINT('Ctrl Pts',(80.3727766468862,18.7051629663718,11.2143449160563));
#29554=CARTESIAN_POINT('Ctrl Pts',(80.49163151063,11.0791438632757,18.7855589416884));
#29555=CARTESIAN_POINT('Ctrl Pts',(80.6104863743736,0.763273373547416,21.7959185916089));
#29556=CARTESIAN_POINT('Ctrl Pts',(80.7293412381174,-9.73790854164409,19.5145533059146));
#29557=CARTESIAN_POINT('Ctrl Pts',(80.8481961018611,-17.8748710625499,12.4953446527907));
#29558=CARTESIAN_POINT('Ctrl Pts',(80.9670509656049,-21.6720806831577,2.44245211979913));
#29559=CARTESIAN_POINT('Ctrl Pts',(81.0859058293486,-20.2076313708922,-8.20343146938788));
#29560=CARTESIAN_POINT('Ctrl Pts',(81.2047606930923,-13.8370696428724,-16.8576438802434));
#29561=CARTESIAN_POINT('Ctrl Pts',(81.3236155568361,-4.10707315842005,-21.4190710248179));
#29562=CARTESIAN_POINT('Ctrl Pts',(81.4424704205798,6.62005961801551,-20.7802662193902));
#29563=CARTESIAN_POINT('Ctrl Pts',(81.5613252843235,15.7399403573933,-15.0963217718923));
#29564=CARTESIAN_POINT('Ctrl Pts',(81.6801801480674,21.0383976259396,-5.74721487571741));
#29565=CARTESIAN_POINT('Ctrl Pts',(81.799035011811,21.2290447852381,4.99723033301097));
#29566=CARTESIAN_POINT('Ctrl Pts',(81.9178898755548,16.2655955398741,14.5284223241216));
#29567=CARTESIAN_POINT('Ctrl Pts',(82.0367447392985,7.35310156169902,20.5323294079885));
#29568=CARTESIAN_POINT('Ctrl Pts',(82.1555996030423,-3.34461613735804,21.5512922208515));
#29569=CARTESIAN_POINT('Ctrl Pts',(82.274454466786,-13.2303107716506,17.3379217434027));
#29570=CARTESIAN_POINT('Ctrl Pts',(82.3933093305297,-19.9038826811303,8.91516167607796));
#29571=CARTESIAN_POINT('Ctrl Pts',(82.5121641942735,-21.7450878400829,-1.67206708055913));
#29572=CARTESIAN_POINT('Ctrl Pts',(82.6310190580172,-18.3069090140539,-11.853342813146));
#29573=CARTESIAN_POINT('Ctrl Pts',(82.749873921761,-10.4240848973699,-19.1568031661661));
#29574=CARTESIAN_POINT('Ctrl Pts',(82.8687287855046,-0.0104479704558075,
-21.809276566056));
#29575=CARTESIAN_POINT('Ctrl Pts',(82.9875836492484,10.4057255683271,-19.1667819127644));
#29576=CARTESIAN_POINT('Ctrl Pts',(83.1064385129921,18.295543668974,-11.8708776150491));
#29577=CARTESIAN_POINT('Ctrl Pts',(83.225293376736,21.743475815752,-1.69290074860202));
#29578=CARTESIAN_POINT('Ctrl Pts',(83.3441482404795,19.9124153530857,8.89608724670601));
#29579=CARTESIAN_POINT('Ctrl Pts',(83.4630031042234,13.2469165340196,17.3252375405224));
#29580=CARTESIAN_POINT('Ctrl Pts',(83.5818579679671,3.36526335796003,21.5480777803121));
#29581=CARTESIAN_POINT('Ctrl Pts',(83.7007128317108,-7.33342572100848,20.5393651481553));
#29582=CARTESIAN_POINT('Ctrl Pts',(83.8195676954546,-16.2516680806413,14.5440000719016));
#29583=CARTESIAN_POINT('Ctrl Pts',(83.9384225591982,-21.2242470874678,5.0175680428792));
#29584=CARTESIAN_POINT('Ctrl Pts',(84.0572774229421,-21.0438944993103,-5.72705489730169));
#29585=CARTESIAN_POINT('Ctrl Pts',(84.1761322866856,-15.7543972427872,-15.0812340679159));
#29586=CARTESIAN_POINT('Ctrl Pts',(84.2949871504297,-6.63996659862833,-20.7739138600291));
#29587=CARTESIAN_POINT('Ctrl Pts',(84.4138420141732,4.08654920147068,-21.4229962684674));
#29588=CARTESIAN_POINT('Ctrl Pts',(84.532696877917,13.8209116211488,-16.8708937361125));
#29589=CARTESIAN_POINT('Ctrl Pts',(84.6515517416606,20.1997622118043,-8.22278906949283));
#29590=CARTESIAN_POINT('Ctrl Pts',(84.7704066054046,21.6744109015202,2.42168651292241));
#29591=CARTESIAN_POINT('Ctrl Pts',(84.8892614691481,17.8868349159939,12.4782126197139));
#29592=CARTESIAN_POINT('Ctrl Pts',(85.008116332892,9.75660138445222,19.5052142495209));
#29593=CARTESIAN_POINT('Ctrl Pts',(85.1269711966357,-0.742389885652297,
21.7966398959218));
#29594=CARTESIAN_POINT('Ctrl Pts',(85.2458260603794,-11.0611399306238,18.7961654847464));
#29595=CARTESIAN_POINT('Ctrl Pts',(85.3646809241231,-18.6944096760982,11.2322615869207));
#29596=CARTESIAN_POINT('Ctrl Pts',(85.4835357878669,-21.7889547321855,0.9413315959743));
#29597=CARTESIAN_POINT('Ctrl Pts',(85.6023906516106,-19.5934655741757,-9.57813970917106));
#29598=CARTESIAN_POINT('Ctrl Pts',(85.7212455153544,-12.640974323403,-17.7721811168431));
#29599=CARTESIAN_POINT('Ctrl Pts',(85.8401003790981,-2.61944247420519,-21.6514012160677));
#29600=CARTESIAN_POINT('Ctrl Pts',(85.9589552428418,8.03805105744712,-20.2739830495313));
#29601=CARTESIAN_POINT('Ctrl Pts',(86.0778101065855,16.7440253156326,-13.9743432662956));
#29602=CARTESIAN_POINT('Ctrl Pts',(86.1966649703293,21.3847992055526,-4.28194073207559));
#29603=CARTESIAN_POINT('Ctrl Pts',(86.3155198340729,20.8336618335766,6.45005334078568));
#29604=CARTESIAN_POINT('Ctrl Pts',(86.4343746978168,15.2244211583821,15.6160703727607));
#29605=CARTESIAN_POINT('Ctrl Pts',(86.5532295615605,5.91891740826824,20.9907377242656));
#29606=CARTESIAN_POINT('Ctrl Pts',(86.6720844253043,-4.82361147614002,21.2691660819614));
#29607=CARTESIAN_POINT('Ctrl Pts',(86.7909392890479,-14.3950392197212,16.3837571807414));
#29608=CARTESIAN_POINT('Ctrl Pts',(86.9097941527918,-20.4715654904424,7.52061565733396));
#29609=CARTESIAN_POINT('Ctrl Pts',(87.0286490165353,-21.5779000657997,-3.16841951849384));
#29610=CARTESIAN_POINT('Ctrl Pts',(87.1475038802793,-17.445441361742,-13.0882095486293));
#29611=CARTESIAN_POINT('Ctrl Pts',(87.2663587440229,-9.07748890325836,-19.8303769179012));
#29612=CARTESIAN_POINT('Ctrl Pts',(87.3852136077667,1.49434288154233,-21.7580236429505));
#29613=CARTESIAN_POINT('Ctrl Pts',(87.5040684715103,11.7033704351114,-18.4031457624334));
#29614=CARTESIAN_POINT('Ctrl Pts',(87.6229233352542,19.0709936724587,-10.5802577397646));
#29615=CARTESIAN_POINT('Ctrl Pts',(87.7417781989977,21.8084632257878,-0.188640462973126));
#29616=CARTESIAN_POINT('Ctrl Pts',(87.8606330627418,19.2511621928582,10.2487759132041));
#29617=CARTESIAN_POINT('Ctrl Pts',(87.9794879264852,12.0199652382065,18.1979418937174));
#29618=CARTESIAN_POINT('Ctrl Pts',(88.0983427902292,1.87049945680621,21.7289181800866));
#29619=CARTESIAN_POINT('Ctrl Pts',(88.2171976539727,-8.73309577897031,19.9844362344835));
#29620=CARTESIAN_POINT('Ctrl Pts',(88.3360525177166,-17.2164252179897,13.3880303334053));
#29621=CARTESIAN_POINT('Ctrl Pts',(88.4549073814603,-21.5198626168885,3.54120974315988));
#29622=CARTESIAN_POINT('Ctrl Pts',(88.5737622452041,-20.5985973659696,-7.16536391605289));
#29623=CARTESIAN_POINT('Ctrl Pts',(88.6926171089477,-14.6762989692325,-16.1322937631492));
#29624=CARTESIAN_POINT('Ctrl Pts',(88.8114719726916,-5.19081341469801,-21.1825425666637));
#29625=CARTESIAN_POINT('Ctrl Pts',(88.9303268364351,5.55492445116913,-21.0899850127204));
#29626=CARTESIAN_POINT('Ctrl Pts',(89.0491817001791,14.9520092602641,-15.8770926990914));
#29627=CARTESIAN_POINT('Ctrl Pts',(89.1680365639226,20.7189685526261,-6.80947836550907));
#29628=CARTESIAN_POINT('Ctrl Pts',(89.2868914276666,21.4556703649268,3.91137606048543));
#29629=CARTESIAN_POINT('Ctrl Pts',(89.4057462914101,16.9832544516763,13.6826065398033));
#29630=CARTESIAN_POINT('Ctrl Pts',(89.524601155154,8.3875568931729,20.1319036075278));
#29631=CARTESIAN_POINT('Ctrl Pts',(89.6434560188976,-2.24451475863544,21.6934738339396));
#29632=CARTESIAN_POINT('Ctrl Pts',(89.7623108826415,-12.3316516023409,17.9881911894731));
#29633=CARTESIAN_POINT('Ctrl Pts',(89.881165746385,-19.4248468046303,9.91564320116563));
#29634=CARTESIAN_POINT('Ctrl Pts',(90.000020610129,-21.8019780443571,-0.564275510439895));
#29635=CARTESIAN_POINT('Ctrl Pts',(90.1188754738725,-18.8859132029279,-10.9071965255139));
#29636=CARTESIAN_POINT('Ctrl Pts',(90.2377303376164,-11.3846294644092,-18.6020123973841));
#29637=CARTESIAN_POINT('Ctrl Pts',(90.35658520136,-1.11932697578227,-21.7805362915212));
#29638=CARTESIAN_POINT('Ctrl Pts',(90.4754400651038,9.4177314546029,-19.6710697920678));
#29639=CARTESIAN_POINT('Ctrl Pts',(90.5942949288476,17.6683047342162,-12.7857601513537));
#29640=CARTESIAN_POINT('Ctrl Pts',(90.7131497925913,21.6292763313123,-2.79625786625162));
#29641=CARTESIAN_POINT('Ctrl Pts',(90.832004656335,20.3389812854855,7.87213385638809));
#29642=CARTESIAN_POINT('Ctrl Pts',(90.9508595200787,14.1106839591675,16.6292893073156));
#29643=CARTESIAN_POINT('Ctrl Pts',(91.0697143838226,4.45652250419733,21.3490990680254));
#29644=CARTESIAN_POINT('Ctrl Pts',(91.1885692475662,-6.27961657422861,20.885668015112));
#29645=CARTESIAN_POINT('Ctrl Pts',(91.30742411131,-15.4911576790111,15.3515014614732));
#29646=CARTESIAN_POINT('Ctrl Pts',(91.4262789750536,-20.9416769234847,6.0902301652791));
#29647=CARTESIAN_POINT('Ctrl Pts',(91.5451338387976,-21.3078666857667,-4.64968114349535));
#29648=CARTESIAN_POINT('Ctrl Pts',(91.6639887025411,-16.5008266420486,-14.2606744047774));
#29649=CARTESIAN_POINT('Ctrl Pts',(91.7828435662849,-7.68762459877395,-20.4094756665753));
#29650=CARTESIAN_POINT('Ctrl Pts',(91.9016984300287,2.99200530595202,-21.6029873055806));
#29651=CARTESIAN_POINT('Ctrl Pts',(92.0205532937724,12.9452465124921,-17.5519538943392));
#29652=CARTESIAN_POINT('Ctrl Pts',(92.1394081575161,19.7555239728282,-9.23889969655227));
#29653=CARTESIAN_POINT('Ctrl Pts',(92.2582630212599,21.7695514346438,1.31590062864715));
#29654=CARTESIAN_POINT('Ctrl Pts',(92.3771178850036,18.4980815456128,11.5539215167952));
#29655=CARTESIAN_POINT('Ctrl Pts',(92.4563544608328,13.3231273996458,16.5048046166698));
#29656=CARTESIAN_POINT('Ctrl Pts',(92.4959727487473,10.3004335667949,18.2141893406225));
#29657=CARTESIAN_POINT('',(92.,10.9270703901696,-17.8460909879584));
#29658=CARTESIAN_POINT('Ctrl Pts',(92.,10.9270703901696,-17.8460909879584));
#29659=CARTESIAN_POINT('Ctrl Pts',(92.,11.2921794592486,-17.6130173722224));
#29660=CARTESIAN_POINT('Ctrl Pts',(92.,11.6496215836174,-17.368828590994));
#29661=CARTESIAN_POINT('Ctrl Pts',(92.,11.99882582637,-17.1137755643941));
#29662=CARTESIAN_POINT('Ctrl Pts',(92.,12.1338901895175,-17.0151267784142));
#29663=CARTESIAN_POINT('Ctrl Pts',(92.,12.2677219209951,-16.9148522548055));
#29664=CARTESIAN_POINT('Ctrl Pts',(92.,12.4002868707347,-16.81296473787));
#29665=CARTESIAN_POINT('Ctrl Pts',(92.,12.7431657755325,-16.5494329348703));
#29666=CARTESIAN_POINT('Ctrl Pts',(92.,13.0775724354481,-16.2751130739695));
#29667=CARTESIAN_POINT('Ctrl Pts',(92.,13.4031395125407,-15.9905322322926));
#29668=CARTESIAN_POINT('Ctrl Pts',(92.,13.7291901755177,-15.7055286842437));
#29669=CARTESIAN_POINT('Ctrl Pts',(92.,14.0463753218874,-15.4102332180127));
#29670=CARTESIAN_POINT('Ctrl Pts',(92.,14.3542883269116,-15.1051388266276));
#29671=CARTESIAN_POINT('Ctrl Pts',(92.,14.5837985359634,-14.8777295376245));
#29672=CARTESIAN_POINT('Ctrl Pts',(92.,14.8081565673134,-14.6448753583735));
#29673=CARTESIAN_POINT('Ctrl Pts',(92.,15.0271787147356,-14.4067694678288));
#29674=CARTESIAN_POINT('Ctrl Pts',(92.,15.0614652272146,-14.3694955177577));
#29675=CARTESIAN_POINT('Ctrl Pts',(92.,15.0956222772878,-14.3320913486537));
#29676=CARTESIAN_POINT('Ctrl Pts',(92.,15.1296372996932,-14.2945708579953));
#29677=CARTESIAN_POINT('Ctrl Pts',(92.,15.419454141796,-13.9748865142016));
#29678=CARTESIAN_POINT('Ctrl Pts',(92.,15.6991446771822,-13.6465657021793));
#29679=CARTESIAN_POINT('Ctrl Pts',(92.,15.9683573898317,-13.3101384802151));
#29680=CARTESIAN_POINT('Ctrl Pts',(92.,16.24637517215,-12.9627078212336));
#29681=CARTESIAN_POINT('Ctrl Pts',(92.,16.5132191271701,-12.6066315155433));
#29682=CARTESIAN_POINT('Ctrl Pts',(92.,16.7684581893239,-12.2424555046393));
#29683=CARTESIAN_POINT('Ctrl Pts',(92.,17.0147113551117,-11.8911006029549));
#29684=CARTESIAN_POINT('Ctrl Pts',(92.,17.2501624348741,-11.5322056524719));
#29685=CARTESIAN_POINT('Ctrl Pts',(92.,17.4743799650063,-11.1662337083294));
#29686=CARTESIAN_POINT('Ctrl Pts',(92.,17.6967831806401,-10.8032231214182));
#29687=CARTESIAN_POINT('Ctrl Pts',(92.,17.9081341661192,-10.4332491691195));
#29688=CARTESIAN_POINT('Ctrl Pts',(92.,18.1079647220086,-10.0567440255743));
#29689=CARTESIAN_POINT('Ctrl Pts',(92.,18.1292790880992,-10.0165851598352));
#29690=CARTESIAN_POINT('Ctrl Pts',(92.,18.150463115333,-9.97635049241957));
#29691=CARTESIAN_POINT('Ctrl Pts',(92.,18.1715137789144,-9.93604517955553));
#29692=CARTESIAN_POINT('Ctrl Pts',(92.,18.3728227038647,-9.55060273632429));
#29693=CARTESIAN_POINT('Ctrl Pts',(92.,18.5615730281604,-9.15940492952969));
#29694=CARTESIAN_POINT('Ctrl Pts',(92.,18.7374063270933,-8.76297535539794));
#29695=CARTESIAN_POINT('Ctrl Pts',(92.,18.910632580253,-8.37242356466628));
#29696=CARTESIAN_POINT('Ctrl Pts',(92.,19.0713223953422,-7.97679356884877));
#29697=CARTESIAN_POINT('Ctrl Pts',(92.,19.219457689155,-7.57672924718513));
#29698=CARTESIAN_POINT('Ctrl Pts',(92.,19.3682726495474,-7.17482937139957));
#29699=CARTESIAN_POINT('Ctrl Pts',(92.,19.504417731036,-6.7684538540207));
#29700=CARTESIAN_POINT('Ctrl Pts',(92.,19.6278254352608,-6.35823462134573));
#29701=CARTESIAN_POINT('Ctrl Pts',(92.,19.7514283151323,-5.94736660580445));
#29702=CARTESIAN_POINT('Ctrl Pts',(92.,19.8622535912408,-5.53264216214906));
#29703=CARTESIAN_POINT('Ctrl Pts',(92.,19.9601827265672,-5.11468346047855));
#29704=CARTESIAN_POINT('Ctrl Pts',(92.,20.0577509900072,-4.6982649495247));
#29705=CARTESIAN_POINT('Ctrl Pts',(92.,20.1425180399432,-4.2786354299643));
#29706=CARTESIAN_POINT('Ctrl Pts',(92.,20.214315269712,-3.85640572218818));
#29707=CARTESIAN_POINT('Ctrl Pts',(92.,20.2856986963168,-3.4366095343343));
#29708=CARTESIAN_POINT('Ctrl Pts',(92.,20.3442614197365,-3.01424251934551));
#29709=CARTESIAN_POINT('Ctrl Pts',(92.,20.3897861214498,-2.58990850333));
#29710=CARTESIAN_POINT('Ctrl Pts',(92.,20.3963829166491,-2.52842002576895));
#29711=CARTESIAN_POINT('Ctrl Pts',(92.,20.402705853733,-2.46689025967155));
#29712=CARTESIAN_POINT('Ctrl Pts',(92.,20.4087541799555,-2.40532105860444));
#29713=CARTESIAN_POINT('Ctrl Pts',(92.,20.4124617649804,-2.36757953483858));
#29714=CARTESIAN_POINT('Ctrl Pts',(92.,20.416066161468,-2.3298231930452));
#29715=CARTESIAN_POINT('Ctrl Pts',(92.,20.4195671916806,-2.29205246118946));
#29716=CARTESIAN_POINT('Ctrl Pts',(92.,20.4231789043748,-2.25308763557207));
#29717=CARTESIAN_POINT('Ctrl Pts',(92.,20.4266797049764,-2.21411724628959));
#29718=CARTESIAN_POINT('Ctrl Pts',(92.,20.4300694323654,-2.17514335803996));
#29719=CARTESIAN_POINT('Ctrl Pts',(92.,20.4671268176833,-1.74907063051458));
#29720=CARTESIAN_POINT('Ctrl Pts',(92.,20.4909193423328,-1.32251843100026));
#29721=CARTESIAN_POINT('Ctrl Pts',(92.,20.5014010397203,-0.896104986036221));
#29722=CARTESIAN_POINT('Ctrl Pts',(92.,20.5118795350299,-0.469821807097898));
#29723=CARTESIAN_POINT('Ctrl Pts',(92.,20.509055396132,-0.0436767532038229));
#29724=CARTESIAN_POINT('Ctrl Pts',(92.,20.4928314192176,0.381720490806974));
#29725=CARTESIAN_POINT('Ctrl Pts',(92.,20.4819546873464,0.666911463789854));
#29726=CARTESIAN_POINT('Ctrl Pts',(92.,20.4650543294267,0.951766487557669));
#29727=CARTESIAN_POINT('Ctrl Pts',(92.,20.4420879241197,1.23610201945244));
#29728=CARTESIAN_POINT('Ctrl Pts',(92.,20.4077857600276,1.66077988879583));
#29729=CARTESIAN_POINT('Ctrl Pts',(92.,20.3599539272904,2.08429948485678));
#29730=CARTESIAN_POINT('Ctrl Pts',(92.,20.2988198171285,2.50606443235308));
#29731=CARTESIAN_POINT('Ctrl Pts',(92.,20.2376806168394,2.92786449669744));
#29732=CARTESIAN_POINT('Ctrl Pts',(92.,20.1632367394275,3.34791014691897));
#29733=CARTESIAN_POINT('Ctrl Pts',(92.,20.0756652657719,3.76559140238497));
#29734=CARTESIAN_POINT('Ctrl Pts',(92.,20.0107921805636,4.07501033237003));
#29735=CARTESIAN_POINT('Ctrl Pts',(92.,19.9387137896103,4.38313147665421));
#29736=CARTESIAN_POINT('Ctrl Pts',(92.,19.8594851502963,4.68969950654939));
#29737=CARTESIAN_POINT('Ctrl Pts',(92.,19.7901600908965,4.95794653270768));
#29738=CARTESIAN_POINT('Ctrl Pts',(92.,19.7153603920804,5.22500440903414));
#29739=CARTESIAN_POINT('Ctrl Pts',(92.,19.6351142811139,5.49069696494022));
#29740=CARTESIAN_POINT('Ctrl Pts',(92.,19.6247466371941,5.52502393454163));
#29741=CARTESIAN_POINT('Ctrl Pts',(92.,19.6142877564505,5.55932912547967));
#29742=CARTESIAN_POINT('Ctrl Pts',(92.,19.6037386647578,5.59360898626946));
#29743=CARTESIAN_POINT('Ctrl Pts',(92.,19.4792224942109,5.99823121506005));
#29744=CARTESIAN_POINT('Ctrl Pts',(92.,19.34242773395,6.39839984507992));
#29745=CARTESIAN_POINT('Ctrl Pts',(92.,19.1936344458134,6.79355365066581));
#29746=CARTESIAN_POINT('Ctrl Pts',(92.,19.0438980499274,7.19121208949771));
#29747=CARTESIAN_POINT('Ctrl Pts',(92.,18.8820103888085,7.58379245980847));
#29748=CARTESIAN_POINT('Ctrl Pts',(92.,18.7082055767162,7.9707113061041));
#29749=CARTESIAN_POINT('Ctrl Pts',(92.,18.5346901736901,8.35698587897231));
#29750=CARTESIAN_POINT('Ctrl Pts',(92.,18.349297063112,8.73761827716024));
#29751=CARTESIAN_POINT('Ctrl Pts',(92.,18.1522110520214,9.11200875632698));
#29752=CARTESIAN_POINT('Ctrl Pts',(92.,17.956955229384,9.4829225547889));
#29753=CARTESIAN_POINT('Ctrl Pts',(92.,17.7502224133289,9.84771028195912));
#29754=CARTESIAN_POINT('Ctrl Pts',(92.,17.5321485463934,10.2057627247099));
#29755=CARTESIAN_POINT('Ctrl Pts',(92.,17.4227884407154,10.3853195580332));
#29756=CARTESIAN_POINT('Ctrl Pts',(92.,17.3105755743928,10.5631821215417));
#29757=CARTESIAN_POINT('Ctrl Pts',(92.,17.1955231821568,10.7392705347842));
#29758=CARTESIAN_POINT('Ctrl Pts',(92.,16.9668897465601,11.0891954525194));
#29759=CARTESIAN_POINT('Ctrl Pts',(92.,16.7270449335161,11.4321165235876));
#29760=CARTESIAN_POINT('Ctrl Pts',(92.,16.4764020151916,11.767600152219));
#29761=CARTESIAN_POINT('Ctrl Pts',(92.,16.3667457384246,11.9143742397452));
#29762=CARTESIAN_POINT('Ctrl Pts',(92.,16.2550222124525,12.0597242811191));
#29763=CARTESIAN_POINT('Ctrl Pts',(92.,16.1412641903407,12.2036116409786));
#29764=CARTESIAN_POINT('Ctrl Pts',(92.,16.0850347937596,12.2747336530385));
#29765=CARTESIAN_POINT('Ctrl Pts',(92.,16.0283083085223,12.3454982768305));
#29766=CARTESIAN_POINT('Ctrl Pts',(92.,15.9710885983828,12.4159007092191));
#29767=CARTESIAN_POINT('Ctrl Pts',(92.,15.9463460917906,12.4463435870882));
#29768=CARTESIAN_POINT('Ctrl Pts',(92.,15.9215113610675,12.476718741088));
#29769=CARTESIAN_POINT('Ctrl Pts',(92.,15.8965847152718,12.5070257774445));
#29770=CARTESIAN_POINT('Ctrl Pts',(92.,15.8714065760418,12.5376385918313));
#29771=CARTESIAN_POINT('Ctrl Pts',(92.,15.8461408680008,12.5681743492675));
#29772=CARTESIAN_POINT('Ctrl Pts',(92.,15.8207895134622,12.5986310019053));
#29773=CARTESIAN_POINT('Ctrl Pts',(92.,15.5526633401512,12.9207528716145));
#29774=CARTESIAN_POINT('Ctrl Pts',(92.,15.2749071405144,13.2340931711695));
#29775=CARTESIAN_POINT('Ctrl Pts',(92.,14.9880458141498,13.5383111481772));
#29776=CARTESIAN_POINT('Ctrl Pts',(92.,14.699003791787,13.8448417650009));
#29777=CARTESIAN_POINT('Ctrl Pts',(92.,14.4007173132838,14.1421112257004));
#29778=CARTESIAN_POINT('Ctrl Pts',(92.,14.0936803430808,14.4297399483924));
#29779=CARTESIAN_POINT('Ctrl Pts',(92.,13.7770001609194,14.7264023217761));
#29780=CARTESIAN_POINT('Ctrl Pts',(92.,13.4510109375165,15.0128094692374));
#29781=CARTESIAN_POINT('Ctrl Pts',(92.,13.1162136914518,15.2885042773823));
#29782=CARTESIAN_POINT('Ctrl Pts',(92.,12.7926192649061,15.5549739224943));
#29783=CARTESIAN_POINT('Ctrl Pts',(92.,12.4607958105108,15.8114362654091));
#29784=CARTESIAN_POINT('Ctrl Pts',(92.,12.1211651035996,16.0574364911078));
#29785=CARTESIAN_POINT('Ctrl Pts',(92.,11.7842321306937,16.3014827027533));
#29786=CARTESIAN_POINT('Ctrl Pts',(92.,11.4396150210109,16.5352326307995));
#29787=CARTESIAN_POINT('Ctrl Pts',(92.,11.0877022244914,16.7581967512111));
#29788=CARTESIAN_POINT('Ctrl Pts',(92.,10.7411333572112,16.9777750769198));
#29789=CARTESIAN_POINT('Ctrl Pts',(92.,10.3874882912748,17.186892894028));
#29790=CARTESIAN_POINT('Ctrl Pts',(92.,10.0271214322955,17.3850347542793));
#29791=CARTESIAN_POINT('Ctrl Pts',(92.,9.97739598921864,17.4123754809515));
#29792=CARTESIAN_POINT('Ctrl Pts',(92.,9.92754254225955,17.4395071465117));
#29793=CARTESIAN_POINT('Ctrl Pts',(92.,9.87756200380534,17.4664283201656));
#29794=CARTESIAN_POINT('Ctrl Pts',(91.4938431528482,-20.9233577741311,-0.000216749186123405));
#29795=CARTESIAN_POINT('Ctrl Pts',(91.5109400481646,-20.9238979401944,-1.49907582982062));
#29796=CARTESIAN_POINT('Ctrl Pts',(91.5280369434811,-20.7650628346641,-2.99782158597188));
#29797=CARTESIAN_POINT('Ctrl Pts',(91.5451338387975,-20.4456617181001,-4.46152813557956));
#29798=CARTESIAN_POINT('Ctrl Pts',(91.5847521267121,-19.7055200045274,-7.85334556392255));
#29799=CARTESIAN_POINT('Ctrl Pts',(91.6243704146266,-18.1031733232879,-11.0570099843501));
#29800=CARTESIAN_POINT('Ctrl Pts',(91.6639887025412,-15.8331329754556,-13.6836424048636));
#29801=CARTESIAN_POINT('Ctrl Pts',(91.7036069904557,-13.5630926276235,-16.3102748253768));
#29802=CARTESIAN_POINT('Ctrl Pts',(91.7432252783703,-10.6253586131987,-18.3598752459761));
#29803=CARTESIAN_POINT('Ctrl Pts',(91.7828435662849,-7.37655328853197,-19.5835940627766));
#29804=CARTESIAN_POINT('Ctrl Pts',(91.8224618541995,-4.12774796386517,-20.8073128795771));
#29805=CARTESIAN_POINT('Ctrl Pts',(91.8620801421141,-0.567871328956467,
-21.2051500925789));
#29806=CARTESIAN_POINT('Ctrl Pts',(91.9016984300287,2.87094052292124,-20.7288964638728));
#29807=CARTESIAN_POINT('Ctrl Pts',(91.9344656200191,5.71508667923201,-20.3350002619699));
#29808=CARTESIAN_POINT('Ctrl Pts',(91.9672328100095,8.47641863398564,-19.343183398648));
#29809=CARTESIAN_POINT('Ctrl Pts',(92.,10.9270703901696,-17.8460909879584));
#29810=CARTESIAN_POINT('',(68.725,-11.6499306790267,-16.3385250883756));
#29811=CARTESIAN_POINT('Ctrl Pts',(68.725,-11.6499306790269,-16.3385250883755));
#29812=CARTESIAN_POINT('Ctrl Pts',(68.725,-11.9987892920946,-16.100985275945));
#29813=CARTESIAN_POINT('Ctrl Pts',(68.725,-12.3397428201089,-15.852668582927));
#29814=CARTESIAN_POINT('Ctrl Pts',(68.725,-12.6722355485707,-15.5938760861607));
#29815=CARTESIAN_POINT('Ctrl Pts',(68.725,-12.7943494799348,-15.4988298897105));
#29816=CARTESIAN_POINT('Ctrl Pts',(68.725,-12.9153219620097,-15.4023701941502));
#29817=CARTESIAN_POINT('Ctrl Pts',(68.725,-13.0351246648751,-15.3045103400552));
#29818=CARTESIAN_POINT('Ctrl Pts',(68.725,-13.3598924567193,-15.0392264360661));
#29819=CARTESIAN_POINT('Ctrl Pts',(68.725,-13.676066145712,-14.7636562391713));
#29820=CARTESIAN_POINT('Ctrl Pts',(68.725,-13.9833264286331,-14.4783477229447));
#29821=CARTESIAN_POINT('Ctrl Pts',(68.725,-14.2918745628573,-14.1918433640893));
#29822=CARTESIAN_POINT('Ctrl Pts',(68.725,-14.5914347756753,-13.8955184759107));
#29823=CARTESIAN_POINT('Ctrl Pts',(68.725,-14.8816491181147,-13.58988796133));
#29824=CARTESIAN_POINT('Ctrl Pts',(68.725,-15.1025513098886,-13.3572514555793));
#29825=CARTESIAN_POINT('Ctrl Pts',(68.725,-15.3180380420484,-13.1192226084338));
#29826=CARTESIAN_POINT('Ctrl Pts',(68.725,-15.5279361392978,-12.8760152733416));
#29827=CARTESIAN_POINT('Ctrl Pts',(68.725,-15.5573089156157,-12.8419812599506));
#29828=CARTESIAN_POINT('Ctrl Pts',(68.725,-15.5865695773343,-12.8078488654536));
#29829=CARTESIAN_POINT('Ctrl Pts',(68.725,-15.615712402069,-12.7736250045455));
#29830=CARTESIAN_POINT('Ctrl Pts',(68.725,-15.8891395467608,-12.4525259809051));
#29831=CARTESIAN_POINT('Ctrl Pts',(68.725,-16.1523380967823,-12.1232148948141));
#29832=CARTESIAN_POINT('Ctrl Pts',(68.725,-16.4049974667961,-11.78624941686));
#29833=CARTESIAN_POINT('Ctrl Pts',(68.725,-16.6638480447255,-11.4410268798691));
#29834=CARTESIAN_POINT('Ctrl Pts',(68.725,-16.9116371170591,-11.0877699117912));
#29835=CARTESIAN_POINT('Ctrl Pts',(68.725,-17.147991537967,-10.7270379841369));
#29836=CARTESIAN_POINT('Ctrl Pts',(68.725,-17.3793535036121,-10.3739257066834));
#29837=CARTESIAN_POINT('Ctrl Pts',(68.725,-17.5997589757048,-10.0136503549057));
#29838=CARTESIAN_POINT('Ctrl Pts',(68.725,-17.8088160791237,-9.64670563770897));
#29839=CARTESIAN_POINT('Ctrl Pts',(68.725,-18.0246399056295,-9.26788371926525));
#29840=CARTESIAN_POINT('Ctrl Pts',(68.725,-18.2283694893187,-8.88195335649133));
#29841=CARTESIAN_POINT('Ctrl Pts',(68.725,-18.4195215195112,-8.48943084625261));
#29842=CARTESIAN_POINT('Ctrl Pts',(68.725,-18.4372721406238,-8.45298070575238));
#29843=CARTESIAN_POINT('Ctrl Pts',(68.725,-18.4549124068542,-8.41647747693315));
#29844=CARTESIAN_POINT('Ctrl Pts',(68.725,-18.4724385493003,-8.37992885242366));
#29845=CARTESIAN_POINT('Ctrl Pts',(68.725,-18.6436470820391,-8.02289441685841));
#29846=CARTESIAN_POINT('Ctrl Pts',(68.725,-18.8040682762284,-7.66132317967038));
#29847=CARTESIAN_POINT('Ctrl Pts',(68.725,-18.9534486909712,-7.29565499339187));
#29848=CARTESIAN_POINT('Ctrl Pts',(68.725,-19.1136552191723,-6.90348557347062));
#29849=CARTESIAN_POINT('Ctrl Pts',(68.725,-19.2611637358523,-6.50660390994598));
#29850=CARTESIAN_POINT('Ctrl Pts',(68.725,-19.3960048313395,-6.10566837001001));
#29851=CARTESIAN_POINT('Ctrl Pts',(68.725,-19.5308721958782,-5.7046547218663));
#29852=CARTESIAN_POINT('Ctrl Pts',(68.725,-19.653067281878,-5.29958508272568));
#29853=CARTESIAN_POINT('Ctrl Pts',(68.725,-19.7625728366385,-4.89109319987111));
#29854=CARTESIAN_POINT('Ctrl Pts',(68.725,-19.8725372525205,-4.48088961349667));
#29855=CARTESIAN_POINT('Ctrl Pts',(68.725,-19.9697056892801,-4.06723451410488));
#29856=CARTESIAN_POINT('Ctrl Pts',(68.725,-20.0540108703053,-3.65075241347895));
#29857=CARTESIAN_POINT('Ctrl Pts',(68.725,-20.1382310371142,-3.23469029770981));
#29858=CARTESIAN_POINT('Ctrl Pts',(68.725,-20.2096139643298,-2.81580633501393));
#29859=CARTESIAN_POINT('Ctrl Pts',(68.725,-20.2680414869829,-2.39471406072667));
#29860=CARTESIAN_POINT('Ctrl Pts',(68.725,-20.326156800138,-1.97587190764284));
#29861=CARTESIAN_POINT('Ctrl Pts',(68.725,-20.3714548499849,-1.5548444432437));
#29862=CARTESIAN_POINT('Ctrl Pts',(68.725,-20.4037677778091,-1.13223450157562));
#29863=CARTESIAN_POINT('Ctrl Pts',(68.725,-20.4091213406707,-1.06221704908848));
#29864=CARTESIAN_POINT('Ctrl Pts',(68.725,-20.4141183529857,-0.992156166950641));
#29865=CARTESIAN_POINT('Ctrl Pts',(68.725,-20.4187579119077,-0.922054610248633));
#29866=CARTESIAN_POINT('Ctrl Pts',(68.725,-20.422098764979,-0.871575889111893));
#29867=CARTESIAN_POINT('Ctrl Pts',(68.725,-20.4252544645954,-0.821072156902455));
#29868=CARTESIAN_POINT('Ctrl Pts',(68.725,-20.4282231742031,-0.770571679141828));
#29869=CARTESIAN_POINT('Ctrl Pts',(68.725,-20.4533182195221,-0.343681903620332));
#29870=CARTESIAN_POINT('Ctrl Pts',(68.725,-20.4650818340108,0.0833365859073504));
#29871=CARTESIAN_POINT('Ctrl Pts',(68.725,-20.463517702269,0.509847184542638));
#29872=CARTESIAN_POINT('Ctrl Pts',(68.725,-20.461948035478,0.937867091567226));
#29873=CARTESIAN_POINT('Ctrl Pts',(68.725,-20.4469562296846,1.36537605047279));
#29874=CARTESIAN_POINT('Ctrl Pts',(68.725,-20.4184952559188,1.79174359745879));
#29875=CARTESIAN_POINT('Ctrl Pts',(68.725,-20.3989647374653,2.0843259705317));
#29876=CARTESIAN_POINT('Ctrl Pts',(68.725,-20.373090542812,2.37637112215609));
#29877=CARTESIAN_POINT('Ctrl Pts',(68.725,-20.3408433469955,2.66767680784106));
#29878=CARTESIAN_POINT('Ctrl Pts',(68.725,-20.2938522813738,3.09217153506962));
#29879=CARTESIAN_POINT('Ctrl Pts',(68.725,-20.2333307283686,3.51509643752233));
#29880=CARTESIAN_POINT('Ctrl Pts',(68.725,-20.1595547533075,3.935873610376));
#29881=CARTESIAN_POINT('Ctrl Pts',(68.725,-20.0857891749123,4.35659148642359));
#29882=CARTESIAN_POINT('Ctrl Pts',(68.725,-19.9987727312683,4.77516275868168));
#29883=CARTESIAN_POINT('Ctrl Pts',(68.725,-19.8987294279677,5.19100075672885));
#29884=CARTESIAN_POINT('Ctrl Pts',(68.725,-19.8236846127296,5.50293053816237));
#29885=CARTESIAN_POINT('Ctrl Pts',(68.725,-19.7413086989252,5.81332221201406));
#29886=CARTESIAN_POINT('Ctrl Pts',(68.725,-19.651677945131,6.12192214555817));
#29887=CARTESIAN_POINT('Ctrl Pts',(68.725,-19.5732510355612,6.39194708740926));
#29888=CARTESIAN_POINT('Ctrl Pts',(68.725,-19.4892693892593,6.66060020105372));
#29889=CARTESIAN_POINT('Ctrl Pts',(68.725,-19.3997746480287,6.92770707799559));
#29890=CARTESIAN_POINT('Ctrl Pts',(68.725,-19.3874363192146,6.96453217443008));
#29891=CARTESIAN_POINT('Ctrl Pts',(68.725,-19.3749922652267,7.00133057306016));
#29892=CARTESIAN_POINT('Ctrl Pts',(68.725,-19.3624457063944,7.03809267495641));
#29893=CARTESIAN_POINT('Ctrl Pts',(68.725,-19.2244394670901,7.44245848548721));
#29894=CARTESIAN_POINT('Ctrl Pts',(68.725,-19.0741889509375,7.84199020533157));
#29895=CARTESIAN_POINT('Ctrl Pts',(68.725,-18.9120227648927,8.23613571192123));
#29896=CARTESIAN_POINT('Ctrl Pts',(68.725,-18.7482047332631,8.63429603522855));
#29897=CARTESIAN_POINT('Ctrl Pts',(68.725,-18.5722269355258,9.02696038238803));
#29898=CARTESIAN_POINT('Ctrl Pts',(68.725,-18.3843755501797,9.41355256367695));
#29899=CARTESIAN_POINT('Ctrl Pts',(68.725,-18.1963904566248,9.80041991221034));
#29900=CARTESIAN_POINT('Ctrl Pts',(68.725,-17.996514678722,10.1812069718227));
#29901=CARTESIAN_POINT('Ctrl Pts',(68.725,-17.7849850009624,10.5553214340206));
#29902=CARTESIAN_POINT('Ctrl Pts',(68.725,-17.5747675470806,10.9271150779981));
#29903=CARTESIAN_POINT('Ctrl Pts',(68.725,-17.3530401041389,11.2923191462909));
#29904=CARTESIAN_POINT('Ctrl Pts',(68.725,-17.119988918834,11.6503300347784));
#29905=CARTESIAN_POINT('Ctrl Pts',(68.725,-17.0041505504421,11.8282797720202));
#29906=CARTESIAN_POINT('Ctrl Pts',(68.725,-16.8855138433729,12.0044519712643));
#29907=CARTESIAN_POINT('Ctrl Pts',(68.725,-16.7640976485875,12.1787698690955));
#29908=CARTESIAN_POINT('Ctrl Pts',(68.725,-16.5175195192571,12.5327834439073));
#29909=CARTESIAN_POINT('Ctrl Pts',(68.725,-16.2594801824049,12.8791515357829));
#29910=CARTESIAN_POINT('Ctrl Pts',(68.725,-15.9904435978116,13.2174610733958));
#29911=CARTESIAN_POINT('Ctrl Pts',(68.725,-15.8727400920521,13.3654714961014));
#29912=CARTESIAN_POINT('Ctrl Pts',(68.725,-15.7529311424556,13.5119389942562));
#29913=CARTESIAN_POINT('Ctrl Pts',(68.725,-15.6310533922898,13.6568266706687));
#29914=CARTESIAN_POINT('Ctrl Pts',(68.725,-15.5693617221597,13.7301654279644));
#29915=CARTESIAN_POINT('Ctrl Pts',(68.725,-15.5071399745656,13.8030993881211));
#29916=CARTESIAN_POINT('Ctrl Pts',(68.725,-15.4443927821345,13.8756236175601));
#29917=CARTESIAN_POINT('Ctrl Pts',(68.725,-15.4207447743093,13.902956371088));
#29918=CARTESIAN_POINT('Ctrl Pts',(68.725,-15.3970214238862,13.9302317377608));
#29919=CARTESIAN_POINT('Ctrl Pts',(68.725,-15.3732251808066,13.9574469290418));
#29920=CARTESIAN_POINT('Ctrl Pts',(68.725,-15.0919796997952,14.2791006260988));
#29921=CARTESIAN_POINT('Ctrl Pts',(68.725,-14.8011916071194,14.5916249436891));
#29922=CARTESIAN_POINT('Ctrl Pts',(68.725,-14.5014254406708,14.8947134294339));
#29923=CARTESIAN_POINT('Ctrl Pts',(68.725,-14.198654557309,15.2008399334786));
#29924=CARTESIAN_POINT('Ctrl Pts',(68.725,-13.886724384795,15.4973408812269));
#29925=CARTESIAN_POINT('Ctrl Pts',(68.725,-13.5661704902236,15.7838736081083));
#29926=CARTESIAN_POINT('Ctrl Pts',(68.725,-13.2438021970466,16.0720281670401));
#29927=CARTESIAN_POINT('Ctrl Pts',(68.725,-12.9127119086089,16.350101727454));
#29928=CARTESIAN_POINT('Ctrl Pts',(68.725,-12.5734032896817,16.6177129020166));
#29929=CARTESIAN_POINT('Ctrl Pts',(68.725,-12.2344059655302,16.8850785597962));
#29930=CARTESIAN_POINT('Ctrl Pts',(68.725,-11.8872049704363,17.142001376928));
#29931=CARTESIAN_POINT('Ctrl Pts',(68.725,-11.5322676984425,17.3880627724302));
#29932=CARTESIAN_POINT('Ctrl Pts',(68.725,-11.179301167814,17.6327579451973));
#29933=CARTESIAN_POINT('Ctrl Pts',(68.725,-10.818683608423,17.8667122980006));
#29934=CARTESIAN_POINT('Ctrl Pts',(68.725,-10.4508464323994,18.0894713180186));
#29935=CARTESIAN_POINT('Ctrl Pts',(68.725,-10.0879532382318,18.3092363052824));
#29936=CARTESIAN_POINT('Ctrl Pts',(68.725,-9.71803277350823,18.5181051321412));
#29937=CARTESIAN_POINT('Ctrl Pts',(68.725,-9.3414780335832,18.7155953847213));
#29938=CARTESIAN_POINT('Ctrl Pts',(68.725,-9.22860300304108,18.7747945287718));
#29939=CARTESIAN_POINT('Ctrl Pts',(68.725,-9.11513173031872,18.8329709265167));
#29940=CARTESIAN_POINT('Ctrl Pts',(68.725,-9.0010745076591,18.8901107118929));
#29941=CARTESIAN_POINT('Ctrl Pts',(68.725,-11.6499306790267,-16.3385250883756));
#29942=CARTESIAN_POINT('Ctrl Pts',(68.7577671899904,-9.40607008510334,-17.9350305838001));
#29943=CARTESIAN_POINT('Ctrl Pts',(68.8301526678954,-3.71778776782437,-20.4401340743294));
#29944=CARTESIAN_POINT('Ctrl Pts',(68.9421564337151,5.98487983261901,-20.039336396671));
#29945=CARTESIAN_POINT('Ctrl Pts',(69.0610112974588,14.8280289192567,-14.7486055907437));
#29946=CARTESIAN_POINT('Ctrl Pts',(69.1798661612025,20.0711408256307,-5.87721609629587));
#29947=CARTESIAN_POINT('Ctrl Pts',(69.2987210249463,20.4412844203846,4.42111651613181));
#29948=CARTESIAN_POINT('Ctrl Pts',(69.4175758886899,15.8485849447886,13.6460461909995));
#29949=CARTESIAN_POINT('Ctrl Pts',(69.5364307524338,7.40808631971404,19.5579297437878));
#29950=CARTESIAN_POINT('Ctrl Pts',(69.6552856161775,-2.83098632764961,20.7214331897253));
#29951=CARTESIAN_POINT('Ctrl Pts',(69.7741404799212,-12.3827371735606,16.8540836193131));
#29952=CARTESIAN_POINT('Ctrl Pts',(69.8883354092291,-18.6715184686174,9.20687033992677));
#29953=CARTESIAN_POINT('Ctrl Pts',(69.9629120506222,-20.0646021687516,2.93742032732148));
#29954=CARTESIAN_POINT('Ctrl Pts',(69.9978704041008,-20.0670795681067,-0.000365800382557055));
#29955=CARTESIAN_POINT('Origin',(68.725,-1.75604157117454E-15,0.));
#29956=CARTESIAN_POINT('',(68.725,-20.925,-2.56257342721584E-15));
#29957=CARTESIAN_POINT('Origin',(68.725,0.,0.));
#29958=CARTESIAN_POINT('Origin',(68.725,0.,0.));
#29959=CARTESIAN_POINT('',(68.725,11.6491905967232,-16.3382590211967));
#29960=CARTESIAN_POINT('Ctrl Pts',(68.725,9.00178625489518,18.890518144815));
#29961=CARTESIAN_POINT('Ctrl Pts',(68.725,9.38925803975212,18.6968856239625));
#29962=CARTESIAN_POINT('Ctrl Pts',(68.725,9.77026673223583,18.4913974126918));
#29963=CARTESIAN_POINT('Ctrl Pts',(68.725,10.1442182949888,18.2742433770339));
#29964=CARTESIAN_POINT('Ctrl Pts',(68.725,10.2888543730052,18.1902530660648));
#29965=CARTESIAN_POINT('Ctrl Pts',(68.725,10.4324345077463,18.1045170779589));
#29966=CARTESIAN_POINT('Ctrl Pts',(68.725,10.5749234040853,18.0170445175294));
#29967=CARTESIAN_POINT('Ctrl Pts',(68.725,10.9434705568083,17.7907969718192));
#29968=CARTESIAN_POINT('Ctrl Pts',(68.725,11.3047195365857,17.5529348738655));
#29969=CARTESIAN_POINT('Ctrl Pts',(68.725,11.6582499229056,17.3039440167568));
#29970=CARTESIAN_POINT('Ctrl Pts',(68.725,12.0123054338337,17.0545833152689));
#29971=CARTESIAN_POINT('Ctrl Pts',(68.725,12.3586197932977,16.794060375687));
#29972=CARTESIAN_POINT('Ctrl Pts',(68.725,12.6967370719532,16.5228229871426));
#29973=CARTESIAN_POINT('Ctrl Pts',(68.725,12.9487607468455,16.3206498130859));
#29974=CARTESIAN_POINT('Ctrl Pts',(68.725,13.1962296143473,16.1125230269113));
#29975=CARTESIAN_POINT('Ctrl Pts',(68.725,13.4389407817561,15.8986155470502));
#29976=CARTESIAN_POINT('Ctrl Pts',(68.725,13.476935663215,15.8651296987176));
#29977=CARTESIAN_POINT('Ctrl Pts',(68.725,13.5148154030423,15.8315008121615));
#29978=CARTESIAN_POINT('Ctrl Pts',(68.725,13.5525660521234,15.7977413953055));
#29979=CARTESIAN_POINT('Ctrl Pts',(68.725,13.8742113629858,15.5101024170764));
#29980=CARTESIAN_POINT('Ctrl Pts',(68.725,14.1866885968815,15.2128157948926));
#29981=CARTESIAN_POINT('Ctrl Pts',(68.725,14.4895927569317,14.906371940508));
#29982=CARTESIAN_POINT('Ctrl Pts',(68.725,14.8024039249045,14.5899053063349));
#29983=CARTESIAN_POINT('Ctrl Pts',(68.725,15.1050061927679,14.2636724048909));
#29984=CARTESIAN_POINT('Ctrl Pts',(68.725,15.396913789591,13.9281711290047));
#29985=CARTESIAN_POINT('Ctrl Pts',(68.725,15.6785445458156,13.6044814440822));
#29986=CARTESIAN_POINT('Ctrl Pts',(68.725,15.9502205399353,13.2721638912857));
#29987=CARTESIAN_POINT('Ctrl Pts',(68.725,16.2114642691751,12.9316338894825));
#29988=CARTESIAN_POINT('Ctrl Pts',(68.725,16.4705940747135,12.5938593775202));
#29989=CARTESIAN_POINT('Ctrl Pts',(68.725,16.7194600643542,12.248004375501));
#29990=CARTESIAN_POINT('Ctrl Pts',(68.725,16.9575514286903,11.8944497505135));
#29991=CARTESIAN_POINT('Ctrl Pts',(68.725,16.9829467777613,11.8567388358725));
#29992=CARTESIAN_POINT('Ctrl Pts',(68.725,17.008220425394,11.8189389107047));
#29993=CARTESIAN_POINT('Ctrl Pts',(68.725,17.0333688243885,11.7810547868178));
#29994=CARTESIAN_POINT('Ctrl Pts',(68.725,17.2738646611779,11.4187663533783));
#29995=CARTESIAN_POINT('Ctrl Pts',(68.725,17.5024722926295,11.0494413563035));
#29996=CARTESIAN_POINT('Ctrl Pts',(68.725,17.7187805264893,10.6735630585382));
#29997=CARTESIAN_POINT('Ctrl Pts',(68.725,17.9318816017938,10.3032578324811));
#29998=CARTESIAN_POINT('Ctrl Pts',(68.725,18.1330457301988,9.92659180879433));
#29999=CARTESIAN_POINT('Ctrl Pts',(68.725,18.322187624511,9.5442034481681));
#30000=CARTESIAN_POINT('Ctrl Pts',(68.725,18.5121973296755,9.16006063345676));
#30001=CARTESIAN_POINT('Ctrl Pts',(68.725,18.69007439373,8.77014233425846));
#30002=CARTESIAN_POINT('Ctrl Pts',(68.725,18.8556856344539,8.37506995850641));
#30003=CARTESIAN_POINT('Ctrl Pts',(68.725,19.0215588002192,7.97937274987526));
#30004=CARTESIAN_POINT('Ctrl Pts',(68.725,19.1751274650245,7.57850461655889));
#30005=CARTESIAN_POINT('Ctrl Pts',(68.725,19.3162087073801,7.17307192876857));
#30006=CARTESIAN_POINT('Ctrl Pts',(68.725,19.4567700648238,6.76913326196687));
#30007=CARTESIAN_POINT('Ctrl Pts',(68.725,19.584935976176,6.36066308509569));
#30008=CARTESIAN_POINT('Ctrl Pts',(68.725,19.7004749109341,5.94825124717928));
#30009=CARTESIAN_POINT('Ctrl Pts',(68.725,19.8153479310481,5.53821636628431));
#30010=CARTESIAN_POINT('Ctrl Pts',(68.725,19.9177392069654,5.12428461199538));
#30011=CARTESIAN_POINT('Ctrl Pts',(68.725,20.0073694943154,4.70703378549649));
#30012=CARTESIAN_POINT('Ctrl Pts',(68.725,20.0203574504677,4.64657168502481));
#30013=CARTESIAN_POINT('Ctrl Pts',(68.725,20.0330773644314,4.58603989614209));
#30014=CARTESIAN_POINT('Ctrl Pts',(68.725,20.0455282938352,4.52544018357549));
#30015=CARTESIAN_POINT('Ctrl Pts',(68.725,20.0531606330853,4.48829295144747));
#30016=CARTESIAN_POINT('Ctrl Pts',(68.725,20.0606918979433,4.45112019629494));
#30017=CARTESIAN_POINT('Ctrl Pts',(68.725,20.0681218669106,4.41392232515951));
#30018=CARTESIAN_POINT('Ctrl Pts',(68.725,20.0757867204331,4.37554851298652));
#30019=CARTESIAN_POINT('Ctrl Pts',(68.725,20.0833418512032,4.33715757420951));
#30020=CARTESIAN_POINT('Ctrl Pts',(68.725,20.0907868831788,4.29875154530138));
#30021=CARTESIAN_POINT('Ctrl Pts',(68.725,20.1721779867712,3.87888644764823));
#30022=CARTESIAN_POINT('Ctrl Pts',(68.725,20.2404270161492,3.45715794634081));
#30023=CARTESIAN_POINT('Ctrl Pts',(68.725,20.2954236349033,3.03417607531588));
#30024=CARTESIAN_POINT('Ctrl Pts',(68.725,20.3504034542094,2.6113234097238));
#30025=CARTESIAN_POINT('Ctrl Pts',(68.725,20.3921390760943,2.18721760469451));
#30026=CARTESIAN_POINT('Ctrl Pts',(68.725,20.420470100454,1.76245484355877));
#30027=CARTESIAN_POINT('Ctrl Pts',(68.725,20.4394635270914,1.47768927209487));
#30028=CARTESIAN_POINT('Ctrl Pts',(68.725,20.4524312120413,1.19262816696663));
#30029=CARTESIAN_POINT('Ctrl Pts',(68.725,20.4593117811368,0.907449630746225));
#30030=CARTESIAN_POINT('Ctrl Pts',(68.725,20.4695884628776,0.481512616615602));
#30031=CARTESIAN_POINT('Ctrl Pts',(68.725,20.4662885233733,0.055313289463583));
#30032=CARTESIAN_POINT('Ctrl Pts',(68.725,20.4495757689587,-0.370531471920013));
#30033=CARTESIAN_POINT('Ctrl Pts',(68.725,20.4328616239798,-0.796411665197902));
#30034=CARTESIAN_POINT('Ctrl Pts',(68.725,20.4027323035974,-1.22193777674415));
#30035=CARTESIAN_POINT('Ctrl Pts',(68.725,20.359300157245,-1.64648465592586));
#30036=CARTESIAN_POINT('Ctrl Pts',(68.725,20.3271255537314,-1.96098966334021));
#30037=CARTESIAN_POINT('Ctrl Pts',(68.725,20.287649461122,-2.27495715534068));
#30038=CARTESIAN_POINT('Ctrl Pts',(68.725,20.2408999456565,-2.58812744623019));
#30039=CARTESIAN_POINT('Ctrl Pts',(68.725,20.1999941196242,-2.86215145075851));
#30040=CARTESIAN_POINT('Ctrl Pts',(68.725,20.1535193450914,-3.1355650759092));
#30041=CARTESIAN_POINT('Ctrl Pts',(68.725,20.1014852795674,-3.4081901651746));
#30042=CARTESIAN_POINT('Ctrl Pts',(68.725,20.094762577507,-3.44341280693583));
#30043=CARTESIAN_POINT('Ctrl Pts',(68.725,20.0879468619263,-3.4786233261834));
#30044=CARTESIAN_POINT('Ctrl Pts',(68.725,20.0810387818474,-3.51381808365658));
#30045=CARTESIAN_POINT('Ctrl Pts',(68.725,19.9994992812284,-3.9292392883932));
#30046=CARTESIAN_POINT('Ctrl Pts',(68.725,19.9052829250088,-4.34151475336195));
#30047=CARTESIAN_POINT('Ctrl Pts',(68.725,19.7986095757904,-4.75005705124187));
#30048=CARTESIAN_POINT('Ctrl Pts',(68.725,19.6912600984964,-5.16118881424805));
#30049=CARTESIAN_POINT('Ctrl Pts',(68.725,19.5712951185248,-5.56854047845237));
#30050=CARTESIAN_POINT('Ctrl Pts',(68.725,19.4388864788952,-5.97150731141695));
#30051=CARTESIAN_POINT('Ctrl Pts',(68.725,19.3066983254461,-6.3738031260997));
#30052=CARTESIAN_POINT('Ctrl Pts',(68.725,19.162107763649,-6.77172923042562));
#30053=CARTESIAN_POINT('Ctrl Pts',(68.725,19.005235896752,-7.16466984645415));
#30054=CARTESIAN_POINT('Ctrl Pts',(68.725,18.8498207943706,-7.55396148476931));
#30055=CARTESIAN_POINT('Ctrl Pts',(68.725,18.6823512228577,-7.9383602804339));
#30056=CARTESIAN_POINT('Ctrl Pts',(68.725,18.5028986988963,-8.31724614652518));
#30057=CARTESIAN_POINT('Ctrl Pts',(68.725,18.4129064453031,-8.50725067915277));
#30058=CARTESIAN_POINT('Ctrl Pts',(68.725,18.3198999557319,-8.69586841528021));
#30059=CARTESIAN_POINT('Ctrl Pts',(68.725,18.22388404251,-8.88301852833684));
#30060=CARTESIAN_POINT('Ctrl Pts',(68.725,18.0330801990091,-9.25492522259813));
#30061=CARTESIAN_POINT('Ctrl Pts',(68.725,17.8303942892476,-9.62103833894468));
#30062=CARTESIAN_POINT('Ctrl Pts',(68.725,17.6161919994574,-9.98088345991726));
#30063=CARTESIAN_POINT('Ctrl Pts',(68.725,17.5224784976742,-10.1383157003428));
#30064=CARTESIAN_POINT('Ctrl Pts',(68.725,17.4265602172733,-10.2945477810432));
#30065=CARTESIAN_POINT('Ctrl Pts',(68.725,17.3284656934938,-10.4495378548228));
#30066=CARTESIAN_POINT('Ctrl Pts',(68.725,17.2799785994724,-10.5261478223335));
#30067=CARTESIAN_POINT('Ctrl Pts',(68.725,17.2309597825059,-10.6024543190805));
#30068=CARTESIAN_POINT('Ctrl Pts',(68.725,17.1814125831296,-10.6784521643853));
#30069=CARTESIAN_POINT('Ctrl Pts',(68.725,17.1599877734037,-10.7113145541013));
#30070=CARTESIAN_POINT('Ctrl Pts',(68.725,17.1384641657444,-10.7441192310031));
#30071=CARTESIAN_POINT('Ctrl Pts',(68.725,17.1168420263571,-10.7768657711699));
#30072=CARTESIAN_POINT('Ctrl Pts',(68.725,17.0950017185671,-10.8099427254663));
#30073=CARTESIAN_POINT('Ctrl Pts',(68.725,17.0730662669445,-10.8429521983094));
#30074=CARTESIAN_POINT('Ctrl Pts',(68.725,17.0510373692289,-10.8758919521138));
#30075=CARTESIAN_POINT('Ctrl Pts',(68.725,16.818050944262,-11.2242759510445));
#30076=CARTESIAN_POINT('Ctrl Pts',(68.725,16.5745693237755,-11.564933096434));
#30077=CARTESIAN_POINT('Ctrl Pts',(68.725,16.3210789145324,-11.8974696375785));
#30078=CARTESIAN_POINT('Ctrl Pts',(68.725,16.0656614747229,-12.232534116885));
#30079=CARTESIAN_POINT('Ctrl Pts',(68.725,15.8000821665744,-12.5593544816777));
#30080=CARTESIAN_POINT('Ctrl Pts',(68.725,15.5247925724923,-12.8775015980273));
#30081=CARTESIAN_POINT('Ctrl Pts',(68.725,15.2408568295324,-13.2056409094765));
#30082=CARTESIAN_POINT('Ctrl Pts',(68.725,14.9465910767754,-13.5245542327704));
#30083=CARTESIAN_POINT('Ctrl Pts',(68.725,14.6424458081594,-13.8337345898222));
#30084=CARTESIAN_POINT('Ctrl Pts',(68.725,14.3484776729286,-14.1325693322663));
#30085=CARTESIAN_POINT('Ctrl Pts',(68.725,14.0452795397488,-14.4223117602991));
#30086=CARTESIAN_POINT('Ctrl Pts',(68.725,13.7332233336194,-14.702465464485));
#30087=CARTESIAN_POINT('Ctrl Pts',(68.725,13.4236458124489,-14.9803938875865));
#30088=CARTESIAN_POINT('Ctrl Pts',(68.725,13.1053499927846,-15.2488856416173));
#30089=CARTESIAN_POINT('Ctrl Pts',(68.725,12.7786710287523,-15.5074132815735));
#30090=CARTESIAN_POINT('Ctrl Pts',(68.725,12.4569527845981,-15.7620151003297));
#30091=CARTESIAN_POINT('Ctrl Pts',(68.725,12.1271036836736,-16.0069533777913));
#30092=CARTESIAN_POINT('Ctrl Pts',(68.725,11.7894223124711,-16.2416784451644));
#30093=CARTESIAN_POINT('Ctrl Pts',(68.725,11.7428273090342,-16.274067010995));
#30094=CARTESIAN_POINT('Ctrl Pts',(68.725,11.6960831511765,-16.3062610424414));
#30095=CARTESIAN_POINT('Ctrl Pts',(68.725,11.6491905967231,-16.3382590211968));
#30096=CARTESIAN_POINT('Origin',(68.725,0.,0.));
#30097=CARTESIAN_POINT('Origin',(65.9521295958992,0.,0.));
#30098=CARTESIAN_POINT('Ctrl Pts',(68.725,11.6491905967231,-16.3382590211968));
#30099=CARTESIAN_POINT('Ctrl Pts',(68.7646182879146,14.3605687349063,-14.4050444314105));
#30100=CARTESIAN_POINT('Ctrl Pts',(68.8438548637438,18.799624465765,-9.16469984651376));
#30101=CARTESIAN_POINT('Ctrl Pts',(68.9627097274874,20.8933712948219,0.927153582356417));
#30102=CARTESIAN_POINT('Ctrl Pts',(69.0815645912312,17.9146243999094,10.7913118927399));
#30103=CARTESIAN_POINT('Ctrl Pts',(69.200419454975,10.5864329691218,18.0367711701248));
#30104=CARTESIAN_POINT('Ctrl Pts',(69.3192743187187,0.688032188973571,20.9025284426369));
#30105=CARTESIAN_POINT('Ctrl Pts',(69.4381291824624,-9.37742221120445,18.6937889137184));
#30106=CARTESIAN_POINT('Ctrl Pts',(69.5569840462062,-17.1661730459504,11.9463094506391));
#30107=CARTESIAN_POINT('Ctrl Pts',(69.6449841840185,-19.847207074249,4.80309241700195));
#30108=CARTESIAN_POINT('Ctrl Pts',(69.6933660339161,-20.0668056364202,0.737086159903154));
#30109=CARTESIAN_POINT('Ctrl Pts',(69.7021295958992,-20.0660502412321,0.000515820514980642));
#30110=CARTESIAN_POINT('Ctrl Pts',(68.2290272512527,12.1479079354045,-17.0377216139053));
#30111=CARTESIAN_POINT('Ctrl Pts',(68.2686455391672,14.9753637768416,-15.0217435370499));
#30112=CARTESIAN_POINT('Ctrl Pts',(68.3478821149964,19.6044613858867,-9.55705283269926));
#30113=CARTESIAN_POINT('Ctrl Pts',(68.4667369787401,21.787844300626,0.966846259998003));
#30114=CARTESIAN_POINT('Ctrl Pts',(68.5855918424839,18.6815732904799,11.2533023034334));
#30115=CARTESIAN_POINT('Ctrl Pts',(68.7044467062276,11.0396522406801,18.8089493263395));
#30116=CARTESIAN_POINT('Ctrl Pts',(68.8233015699713,0.717487761819058,21.7973934781148));
#30117=CARTESIAN_POINT('Ctrl Pts',(68.9421564337151,-9.7788821246665,19.4940948731338));
#30118=CARTESIAN_POINT('Ctrl Pts',(69.0610112974588,-17.9010797388866,12.457746842518));
#30119=CARTESIAN_POINT('Ctrl Pts',(69.1798661612025,-21.6771639701384,2.39693115856188));
#30120=CARTESIAN_POINT('Ctrl Pts',(69.2987210249463,-20.1903538023596,-8.24586855545789));
#30121=CARTESIAN_POINT('Ctrl Pts',(69.41757588869,-13.8016266268924,-16.8866712137983));
#30122=CARTESIAN_POINT('Ctrl Pts',(69.5364307524337,-4.062069390721,-21.4276527915994));
#30123=CARTESIAN_POINT('Ctrl Pts',(69.6552856161776,6.66369771808618,-20.7663129975645));
#30124=CARTESIAN_POINT('Ctrl Pts',(69.7741404799212,15.7716181964099,-15.0632241959129));
#30125=CARTESIAN_POINT('Ctrl Pts',(69.892995343665,21.0504242506639,-5.70300701887552));
#30126=CARTESIAN_POINT('Ctrl Pts',(70.0118502074087,21.2185003328937,5.04181468411517));
#30127=CARTESIAN_POINT('Ctrl Pts',(70.1307050711524,16.2350400350607,14.5625591469258));
#30128=CARTESIAN_POINT('Ctrl Pts',(70.2495599348962,7.30995343255451,20.5477305886088));
#30129=CARTESIAN_POINT('Ctrl Pts',(70.3684147986399,-3.38988116968799,21.5442186838522));
#30130=CARTESIAN_POINT('Ctrl Pts',(70.4872696623837,-13.2667030288609,17.3100907863903));
#30131=CARTESIAN_POINT('Ctrl Pts',(70.6061245261274,-19.9225666650911,8.87333026802901));
#30132=CARTESIAN_POINT('Ctrl Pts',(70.7249793898711,-21.741527356917,-1.71774290924665));
#30133=CARTESIAN_POINT('Ctrl Pts',(70.8438342536149,-18.2819684963326,-11.8917736436063));
#30134=CARTESIAN_POINT('Ctrl Pts',(70.9626891173586,-10.3838195318354,-19.1786585677004));
#30135=CARTESIAN_POINT('Ctrl Pts',(71.0815439811023,0.0353664108211744,
-21.8092503703829));
#30136=CARTESIAN_POINT('Ctrl Pts',(71.2003988448461,10.4459659148443,-19.144880480705));
#30137=CARTESIAN_POINT('Ctrl Pts',(71.3192537085898,18.3204402229448,-11.8324182881816));
#30138=CARTESIAN_POINT('Ctrl Pts',(71.4381085723336,21.7469840640831,-1.64722087984511));
#30139=CARTESIAN_POINT('Ctrl Pts',(71.5569634360772,19.8936835452454,8.93789726458204));
#30140=CARTESIAN_POINT('Ctrl Pts',(71.675818299821,13.2104924744173,17.3530268568187));
#30141=CARTESIAN_POINT('Ctrl Pts',(71.7946731635647,3.31999026665197,21.555099562281));
#30142=CARTESIAN_POINT('Ctrl Pts',(71.9135280273085,-7.37655621064897,20.5239146115309));
#30143=CARTESIAN_POINT('Ctrl Pts',(72.0323828910521,-16.2821845270664,14.5098283772393));
#30144=CARTESIAN_POINT('Ctrl Pts',(72.151237754796,-21.2347405512553,4.97297156951684));
#30145=CARTESIAN_POINT('Ctrl Pts',(72.2700926185397,-21.031817323487,-5.77124878876516));
#30146=CARTESIAN_POINT('Ctrl Pts',(72.3889474822835,-15.7226815860593,-15.1142957577833));
#30147=CARTESIAN_POINT('Ctrl Pts',(72.5078023460271,-6.59631255084762,-20.7878164616172));
#30148=CARTESIAN_POINT('Ctrl Pts',(72.626657209771,4.13154308662491,-21.4143644368381));
#30149=CARTESIAN_POINT('Ctrl Pts',(72.7455120735146,13.8563214974062,-16.8418231516327));
#30150=CARTESIAN_POINT('Ctrl Pts',(72.8643669372584,20.2169910877431,-8.18033763780386));
#30151=CARTESIAN_POINT('Ctrl Pts',(72.983221801002,21.6692758622504,2.46721221544587));
#30152=CARTESIAN_POINT('Ctrl Pts',(73.102076664746,17.8605826726939,12.515759629452));
#30153=CARTESIAN_POINT('Ctrl Pts',(73.2209315284895,9.71560559143255,19.5256667108214));
#30154=CARTESIAN_POINT('Ctrl Pts',(73.3397863922334,-0.788176059440954,
21.7950322553025));
#30155=CARTESIAN_POINT('Ctrl Pts',(73.458641255977,-11.1006002830113,18.7728880534446));
#30156=CARTESIAN_POINT('Ctrl Pts',(73.5774961197208,-18.717963820288,11.1929657791286));
#30157=CARTESIAN_POINT('Ctrl Pts',(73.6963509834645,-21.790884072211,0.895557849507379));
#30158=CARTESIAN_POINT('Ctrl Pts',(73.8152058472083,-19.5733016949674,-9.61927820931176));
#30159=CARTESIAN_POINT('Ctrl Pts',(73.934060710952,-12.6036127150021,-17.79869655454));
#30160=CARTESIAN_POINT('Ctrl Pts',(74.0529155746958,-2.57395397957607,-21.656856037324));
#30161=CARTESIAN_POINT('Ctrl Pts',(74.1717704384395,8.08062250820797,-20.2570529048575));
#30162=CARTESIAN_POINT('Ctrl Pts',(74.2906253021832,16.7733440073046,-13.9391385430726));
#30163=CARTESIAN_POINT('Ctrl Pts',(74.409480165927,21.3937469957573,-4.23700861361877));
#30164=CARTESIAN_POINT('Ctrl Pts',(74.5283350296706,20.8200663319033,6.49380400424132));
#30165=CARTESIAN_POINT('Ctrl Pts',(74.6471898934145,15.1915831504761,15.6480175706868));
#30166=CARTESIAN_POINT('Ctrl Pts',(74.7660447571581,5.87480947415842,21.0031251520504));
#30167=CARTESIAN_POINT('Ctrl Pts',(74.8848996209019,-4.86828058592294,21.2589862563359));
#30168=CARTESIAN_POINT('Ctrl Pts',(75.0037544846456,-14.4294245095375,16.3534816119967));
#30169=CARTESIAN_POINT('Ctrl Pts',(75.1226093483894,-20.4873187232229,7.47759480337299));
#30170=CARTESIAN_POINT('Ctrl Pts',(75.2414642121331,-21.571196590871,-3.21374083403576));
#30171=CARTESIAN_POINT('Ctrl Pts',(75.3603190758769,-17.4179086831383,-13.1248279842522));
#30172=CARTESIAN_POINT('Ctrl Pts',(75.4791739396206,-9.03581154594236,-19.8494020619405));
#30173=CARTESIAN_POINT('Ctrl Pts',(75.5980288033643,1.54004627494346,-21.7548364733313));
#30174=CARTESIAN_POINT('Ctrl Pts',(75.7168836671081,11.7420037602749,-18.3785200765471));
#30175=CARTESIAN_POINT('Ctrl Pts',(75.8357385308518,19.0931773325003,-10.5401722879682));
#30176=CARTESIAN_POINT('Ctrl Pts',(75.9545933945955,21.8088113579133,-0.142827396904615));
#30177=CARTESIAN_POINT('Ctrl Pts',(76.0734482583393,19.2295902757642,10.289193862329));
#30178=CARTESIAN_POINT('Ctrl Pts',(76.1923031220829,11.9817106125957,18.2231518488533));
#30179=CARTESIAN_POINT('Ctrl Pts',(76.3111579858268,1.82484977694283,21.7327995389905));
#30180=CARTESIAN_POINT('Ctrl Pts',(76.4300128495704,-8.77505744961176,19.9660466609283));
#30181=CARTESIAN_POINT('Ctrl Pts',(76.5488677133143,-17.2445112097343,13.3518345424028));
#30182=CARTESIAN_POINT('Ctrl Pts',(76.6677225770579,-21.5272540685705,3.49599553454599));
#30183=CARTESIAN_POINT('Ctrl Pts',(76.7865774408017,-20.5834997430292,-7.20861920474871));
#30184=CARTESIAN_POINT('Ctrl Pts',(76.9054323045454,-14.6423777500227,-16.1630883910221));
#30185=CARTESIAN_POINT('Ctrl Pts',(77.0242871682892,-5.14630416684486,-21.1934000559766));
#30186=CARTESIAN_POINT('Ctrl Pts',(77.1431420320329,5.59921554412473,-21.0782693265074));
#30187=CARTESIAN_POINT('Ctrl Pts',(77.2619968957766,14.9853289795481,-15.8456482317723));
#30188=CARTESIAN_POINT('Ctrl Pts',(77.3808517595204,20.733227365848,-6.76593936614905));
#30189=CARTESIAN_POINT('Ctrl Pts',(77.4997066232641,21.4474064442648,3.95643897019295));
#30190=CARTESIAN_POINT('Ctrl Pts',(77.6185614870079,16.9544741541765,13.7182527555704));
#30191=CARTESIAN_POINT('Ctrl Pts',(77.7374163507515,8.34524764713181,20.1494787579826));
#30192=CARTESIAN_POINT('Ctrl Pts',(77.8562712144953,-2.29008089743881,21.6887109343442));
#30193=CARTESIAN_POINT('Ctrl Pts',(77.9751260782391,-12.3694118528912,17.9622466001307));
#30194=CARTESIAN_POINT('Ctrl Pts',(78.0939809419827,-19.4456335397104,9.87481588434143));
#30195=CARTESIAN_POINT('Ctrl Pts',(78.2128358057266,-21.8007445535193,-0.610073292771518));
#30196=CARTESIAN_POINT('Ctrl Pts',(78.3316906694703,-18.8629589599221,-10.9468457459968));
#30197=CARTESIAN_POINT('Ctrl Pts',(78.450545533214,-11.3455274171,-18.6258868282341));
#30198=CARTESIAN_POINT('Ctrl Pts',(78.5694003969577,-1.07357052181668,-21.7828395496326));
#30199=CARTESIAN_POINT('Ctrl Pts',(78.6882552607015,9.45903333250906,-19.651242732327));
#30200=CARTESIAN_POINT('Ctrl Pts',(78.8071101244452,17.6951245465407,-12.7486163873874));
#30201=CARTESIAN_POINT('Ctrl Pts',(78.925964988189,21.6351026415876,-2.75081555149077));
#30202=CARTESIAN_POINT('Ctrl Pts',(79.0448198519327,20.3223995224024,7.91484239654908));
#30203=CARTESIAN_POINT('Ctrl Pts',(79.1636747156765,14.0757199868426,16.6588943019143));
#30204=CARTESIAN_POINT('Ctrl Pts',(79.2825295794201,4.41166493998945,21.3584143832734));
#30205=CARTESIAN_POINT('Ctrl Pts',(79.4013844431639,-6.32347675422834,20.8724290452522));
#30206=CARTESIAN_POINT('Ctrl Pts',(79.5202393069077,-15.5233723206223,15.3189283014737));
#30207=CARTESIAN_POINT('Ctrl Pts',(79.6390941706513,-20.9544239152145,6.04621955372461));
#30208=CARTESIAN_POINT('Ctrl Pts',(79.7579490343952,-21.2980529688603,-4.694421396293));
#30209=CARTESIAN_POINT('Ctrl Pts',(79.8768038981389,-16.4708314569902,-14.2953266358547));
#30210=CARTESIAN_POINT('Ctrl Pts',(79.9956587618826,-7.64473698342631,-20.4255391352245));
#30211=CARTESIAN_POINT('Ctrl Pts',(80.1145136256263,3.03738595488812,-21.5967344538799));
#30212=CARTESIAN_POINT('Ctrl Pts',(80.23336848937,12.9820767483259,-17.5245637837559));
#30213=CARTESIAN_POINT('Ctrl Pts',(80.3522233531138,19.7749123466527,-9.19768961166646));
#30214=CARTESIAN_POINT('Ctrl Pts',(80.4710782168576,21.7666932739152,1.36224683139497));
#30215=CARTESIAN_POINT('Ctrl Pts',(80.5899330806012,18.4738447381279,11.591449999974));
#30216=CARTESIAN_POINT('Ctrl Pts',(80.7087879443451,10.6958214001617,19.0064214697612));
#30217=CARTESIAN_POINT('Ctrl Pts',(80.8276428080887,0.321011669723394,21.8069164261767));
#30218=CARTESIAN_POINT('Ctrl Pts',(80.9464976718325,-10.1317349207816,19.3130163362787));
#30219=CARTESIAN_POINT('Ctrl Pts',(81.0653525355763,-18.12464692822,12.1302030583876));
#30220=CARTESIAN_POINT('Ctrl Pts',(81.1842073993199,-21.7171641692642,2.00235685020962));
#30221=CARTESIAN_POINT('Ctrl Pts',(81.3030622630637,-20.0370768773855,-8.61163182678505));
#30222=CARTESIAN_POINT('Ctrl Pts',(81.4219171268075,-13.4922852646845,-17.1348443484828));
#30223=CARTESIAN_POINT('Ctrl Pts',(81.5407719905511,-3.67176741574004,-21.4979714520943));
#30224=CARTESIAN_POINT('Ctrl Pts',(81.6596268542949,7.04020096372379,-20.6417107551854));
#30225=CARTESIAN_POINT('Ctrl Pts',(81.7784817180386,16.042913234761,-14.7739496226393));
#30226=CARTESIAN_POINT('Ctrl Pts',(81.8973365817824,21.150644725453,-5.31929320568268));
#30227=CARTESIAN_POINT('Ctrl Pts',(82.0161914455261,21.1233141802142,5.42680850540308));
#30228=CARTESIAN_POINT('Ctrl Pts',(82.1350463092699,15.9675570490321,14.8553618063061));
#30229=CARTESIAN_POINT('Ctrl Pts',(82.2539011730136,6.935114498877,20.6772541551778));
#30230=CARTESIAN_POINT('Ctrl Pts',(82.3727560367573,-3.78107072864253,21.4790166594134));
#30231=CARTESIAN_POINT('Ctrl Pts',(82.491610900501,-13.5792682065756,17.0659933049395));
#30232=CARTESIAN_POINT('Ctrl Pts',(82.6104657642449,-20.0806212833829,8.50960054195855));
#30233=CARTESIAN_POINT('Ctrl Pts',(82.7293206279884,-21.7066981050834,-2.11279669753649));
#30234=CARTESIAN_POINT('Ctrl Pts',(82.8481754917323,-18.0627113986171,-12.2222383154895));
#30235=CARTESIAN_POINT('Ctrl Pts',(82.9670303554759,-10.0333669513822,-19.3643022112666));
#30236=CARTESIAN_POINT('Ctrl Pts',(83.0858852192198,0.431929798649459,-21.8050014712082));
#30237=CARTESIAN_POINT('Ctrl Pts',(83.2047400829634,10.7923604162288,-18.9517706074279));
#30238=CARTESIAN_POINT('Ctrl Pts',(83.3235949467072,18.5325664037399,-11.4973316470095));
#30239=CARTESIAN_POINT('Ctrl Pts',(83.442449810451,21.773340841834,-1.25151152438869));
#30240=CARTESIAN_POINT('Ctrl Pts',(83.5613046741946,19.7278718862347,9.29815698677236));
#30241=CARTESIAN_POINT('Ctrl Pts',(83.6801595379384,12.892768983884,17.5903712422038));
#30242=CARTESIAN_POINT('Ctrl Pts',(83.7990144016822,2.92749348365049,21.6119049232949));
#30243=CARTESIAN_POINT('Ctrl Pts',(83.9178692654259,-7.74853390350953,20.3863894512127));
#30244=CARTESIAN_POINT('Ctrl Pts',(84.0367241291696,-16.5433324771502,14.2113617595507));
#30245=CARTESIAN_POINT('Ctrl Pts',(84.1555789929134,-21.3216559194696,4.58602675113233));
#30246=CARTESIAN_POINT('Ctrl Pts',(84.2744338566571,-20.9233983508335,-6.15272735969124));
#30247=CARTESIAN_POINT('Ctrl Pts',(84.3932887204009,-15.4452507869423,-15.397690756695));
#30248=CARTESIAN_POINT('Ctrl Pts',(84.5121435841446,-6.21722599798435,-20.9043237967732));
#30249=CARTESIAN_POINT('Ctrl Pts',(84.6309984478883,4.52024881509651,-21.3356978596898));
#30250=CARTESIAN_POINT('Ctrl Pts',(84.7498533116321,14.1602744305448,-16.5870817373646));
#30251=CARTESIAN_POINT('Ctrl Pts',(84.8687081753757,20.3623959730666,-7.81136881387576));
#30252=CARTESIAN_POINT('Ctrl Pts',(84.9875630391196,21.6208305557273,2.86082830503407));
#30253=CARTESIAN_POINT('Ctrl Pts',(85.1064179028633,17.6300489743814,12.8384588510953));
#30254=CARTESIAN_POINT('Ctrl Pts',(85.225272766607,9.35895365531763,19.6991024919404));
#30255=CARTESIAN_POINT('Ctrl Pts',(85.3441276303508,-1.18435644657133,21.7770969671767));
#30256=CARTESIAN_POINT('Ctrl Pts',(85.4629824940945,-11.4401224142391,18.5679361173389));
#30257=CARTESIAN_POINT('Ctrl Pts',(85.5818373578382,-18.9183967707379,10.8507564775589));
#30258=CARTESIAN_POINT('Ctrl Pts',(85.700692221582,-21.8035657018886,0.499174512350522));
#30259=CARTESIAN_POINT('Ctrl Pts',(85.8195470853257,-19.3951530927588,-9.97359960188911));
#30260=CARTESIAN_POINT('Ctrl Pts',(85.9384019490694,-12.2778857125101,-18.0249320370673));
#30261=CARTESIAN_POINT('Ctrl Pts',(86.0572568128131,-2.17973024954803,-21.7000789986939));
#30262=CARTESIAN_POINT('Ctrl Pts',(86.1761116765569,8.44763130610374,-20.1067694527612));
#30263=CARTESIAN_POINT('Ctrl Pts',(86.2949665403006,17.0240335942439,-13.6318352650114));
#30264=CARTESIAN_POINT('Ctrl Pts',(86.4138214040445,21.4672536677061,-3.84729417600341));
#30265=CARTESIAN_POINT('Ctrl Pts',(86.532676267788,20.6985437619337,6.87131273088848));
#30266=CARTESIAN_POINT('Ctrl Pts',(86.651531131532,14.9045352115744,15.9216670809716));
#30267=CARTESIAN_POINT('Ctrl Pts',(86.7703859952754,5.49192713757767,21.1064774139573));
#30268=CARTESIAN_POINT('Ctrl Pts',(86.8892408590194,-5.25403918220026,21.1669488774896));
#30269=CARTESIAN_POINT('Ctrl Pts',(87.008095722763,-14.7244029144438,16.0883998994143));
#30270=CARTESIAN_POINT('Ctrl Pts',(87.1269505865068,-20.6199005662829,7.10382665518801));
#30271=CARTESIAN_POINT('Ctrl Pts',(87.2458054502505,-21.5091929720396,-3.60545006925838));
#30272=CARTESIAN_POINT('Ctrl Pts',(87.3646603139942,-17.1763731590936,-13.439377128793));
#30273=CARTESIAN_POINT('Ctrl Pts',(87.483515177738,-8.67338535036549,-20.0104232607513));
#30274=CARTESIAN_POINT('Ctrl Pts',(87.6023700414818,1.93537145092961,-21.7232361736755));
#30275=CARTESIAN_POINT('Ctrl Pts',(87.7212249052254,12.0742488423013,-18.1619703612943));
#30276=CARTESIAN_POINT('Ctrl Pts',(87.8400797689693,19.2816781550306,-10.1912482079563));
#30277=CARTESIAN_POINT('Ctrl Pts',(87.9589346327128,21.8078027241847,0.253757469630748));
#30278=CARTESIAN_POINT('Ctrl Pts',(88.0777894964568,19.0393170670483,10.6371546068841));
#30279=CARTESIAN_POINT('Ctrl Pts',(88.1966443602003,11.6483683346654,18.4380087767184));
#30280=CARTESIAN_POINT('Ctrl Pts',(88.3154992239443,1.4293689781864,21.7623885829307));
#30281=CARTESIAN_POINT('Ctrl Pts',(88.4343540876878,-9.13665991193285,19.8031840410625));
#30282=CARTESIAN_POINT('Ctrl Pts',(88.5532089514317,-17.4844436346792,13.0360608811034));
#30283=CARTESIAN_POINT('Ctrl Pts',(88.6720638151753,-21.5872644310895,3.10397598135163));
#30284=CARTESIAN_POINT('Ctrl Pts',(88.7909186789191,-20.4490184194228,-7.58170813158806));
#30285=CARTESIAN_POINT('Ctrl Pts',(88.9097735426628,-14.3460548059972,-16.4266662476692));
#30286=CARTESIAN_POINT('Ctrl Pts',(89.0286284064066,-4.7600824069233,-21.2834740583831));
#30287=CARTESIAN_POINT('Ctrl Pts',(89.1474832701503,5.98156721951559,-20.9729708458168));
#30288=CARTESIAN_POINT('Ctrl Pts',(89.266338133894,15.2709812692953,-15.5705421742144));
#30289=CARTESIAN_POINT('Ctrl Pts',(89.3851929976378,20.8528281411215,-6.38781739004154));
#30290=CARTESIAN_POINT('Ctrl Pts',(89.5040478613815,21.371918416116,4.3457744682298));
#30291=CARTESIAN_POINT('Ctrl Pts',(89.6229027251252,16.7022246916625,14.0242769125449));
#30292=CARTESIAN_POINT('Ctrl Pts',(89.741757588869,7.97747917221166,20.2978934460202));
#30293=CARTESIAN_POINT('Ctrl Pts',(89.8606124526128,-2.68407967420241,21.643483299709));
#30294=CARTESIAN_POINT('Ctrl Pts',(89.9794673163564,-12.6939838742683,17.7343571895906));
#30295=CARTESIAN_POINT('Ctrl Pts',(90.0983221801002,-19.6219775704911,9.5195929572056));
#30296=CARTESIAN_POINT('Ctrl Pts',(90.2171770438439,-21.7860468354839,-1.00638708659696));
#30297=CARTESIAN_POINT('Ctrl Pts',(90.3360319075877,-18.6607879782059,-11.2880309276121));
#30298=CARTESIAN_POINT('Ctrl Pts',(90.4548867713314,-11.004967087704,-18.829109461369));
#30299=CARTESIAN_POINT('Ctrl Pts',(90.5737416350751,-0.677304206385872,
-21.7987587216074));
#30300=CARTESIAN_POINT('Ctrl Pts',(90.692596498819,9.81479880737376,-19.4759964125881));
#30301=CARTESIAN_POINT('Ctrl Pts',(90.8114513625626,17.9240131542646,-12.4247460608585));
#30302=CARTESIAN_POINT('Ctrl Pts',(90.9303062263064,21.6815465004587,-2.35696335287487));
#30303=CARTESIAN_POINT('Ctrl Pts',(91.0491610900501,20.1751171149987,8.28307709509201));
#30304=CARTESIAN_POINT('Ctrl Pts',(91.1680159537938,13.77048037642,16.912066178113));
#30305=CARTESIAN_POINT('Ctrl Pts',(91.2868708175375,4.02255397575585,21.4351424078077));
#30306=CARTESIAN_POINT('Ctrl Pts',(91.4057256812813,-6.70194588462795,20.753917039625));
#30307=CARTESIAN_POINT('Ctrl Pts',(91.5245805450251,-15.7993971343879,15.0342790497535));
#30308=CARTESIAN_POINT('Ctrl Pts',(91.6434354087688,-21.0608241866243,5.6638924707422));
#30309=CARTESIAN_POINT('Ctrl Pts',(91.7622902725125,-21.2093216757592,-5.08031741261938));
#30310=CARTESIAN_POINT('Ctrl Pts',(91.8811451362563,-16.2078709329371,-14.5937344397854));
#30311=CARTESIAN_POINT('Ctrl Pts',(91.9603817120854,-10.2510427877187,-18.5696101441575));
#30312=CARTESIAN_POINT('Ctrl Pts',(92.,-6.97721143603873,-19.7274971949513));
#30313=CARTESIAN_POINT('Ctrl Pts',(68.3943515008351,11.9816688225107,-16.8045674163358));
#30314=CARTESIAN_POINT('Ctrl Pts',(68.4339697887497,14.7704320961965,-14.8161771685034));
#30315=CARTESIAN_POINT('Ctrl Pts',(68.5132063645788,19.3361824125128,-9.42626850397076));
#30316=CARTESIAN_POINT('Ctrl Pts',(68.6320612283226,21.4896866320246,0.953615367450808));
#30317=CARTESIAN_POINT('Ctrl Pts',(68.7509160920663,18.4259236602897,11.0993054998689));
#30318=CARTESIAN_POINT('Ctrl Pts',(68.86977095581,10.8885791501607,18.5515566076013));
#30319=CARTESIAN_POINT('Ctrl Pts',(68.9886258195538,0.707669237537231,21.4991051329555));
#30320=CARTESIAN_POINT('Ctrl Pts',(69.1074806832975,-9.64506215351249,19.2273262199953));
#30321=CARTESIAN_POINT('Ctrl Pts',(69.2263355470413,-17.6561108412412,12.2872677118917));
#30322=CARTESIAN_POINT('Ctrl Pts',(69.345190410785,-21.3805209162388,2.36413014363932));
#30323=CARTESIAN_POINT('Ctrl Pts',(69.4640452745287,-19.9140571327632,-8.13302724311118));
#30324=CARTESIAN_POINT('Ctrl Pts',(69.5829001382725,-13.6127570553459,-16.6555840786934));
#30325=CARTESIAN_POINT('Ctrl Pts',(69.7017550020162,-4.00648164543864,-21.134424195333));
#30326=CARTESIAN_POINT('Ctrl Pts',(69.82060986576,6.57250776149964,-20.4821345637842));
#30327=CARTESIAN_POINT('Ctrl Pts',(69.9394647295037,15.5557901022382,-14.8570901816477));
#30328=CARTESIAN_POINT('Ctrl Pts',(70.0583195932474,20.7623578714917,-5.62496371852402));
#30329=CARTESIAN_POINT('Ctrl Pts',(70.1771744569912,20.9281339018149,4.97281952833043));
#30330=CARTESIAN_POINT('Ctrl Pts',(70.2960293207349,16.0128702040433,14.3632765274886));
#30331=CARTESIAN_POINT('Ctrl Pts',(70.4148841844786,7.20991973289324,20.2665433649984));
#30332=CARTESIAN_POINT('Ctrl Pts',(70.5337390482224,-3.34349204314369,21.2493949313972));
#30333=CARTESIAN_POINT('Ctrl Pts',(70.6525939119661,-13.0851536662652,17.0732093289622));
#30334=CARTESIAN_POINT('Ctrl Pts',(70.7714487757099,-19.64993455209,8.75190240077688));
#30335=CARTESIAN_POINT('Ctrl Pts',(70.8903036394536,-21.4440035165991,-1.69423630556385));
#30336=CARTESIAN_POINT('Ctrl Pts',(71.0091585031973,-18.0317872930387,-11.7290396229207));
#30337=CARTESIAN_POINT('Ctrl Pts',(71.1280133669411,-10.2417212416112,-18.9162065303833));
#30338=CARTESIAN_POINT('Ctrl Pts',(71.2468682306848,0.0348824360666644,
-21.5107997685402));
#30339=CARTESIAN_POINT('Ctrl Pts',(71.3657230944286,10.3030171769846,-18.8828906825855));
#30340=CARTESIAN_POINT('Ctrl Pts',(71.4845779581722,18.0697325499298,-11.6704965210695));
#30341=CARTESIAN_POINT('Ctrl Pts',(71.603432821916,21.4493855509768,-1.62467934106641));
#30342=CARTESIAN_POINT('Ctrl Pts',(71.7222876856598,19.6214466858341,8.81558582459576));
#30343=CARTESIAN_POINT('Ctrl Pts',(71.8411425494034,13.02971233009,17.1155578369645));
#30344=CARTESIAN_POINT('Ctrl Pts',(71.9599974131473,3.27455756830758,21.2601269094897));
#30345=CARTESIAN_POINT('Ctrl Pts',(72.0788522768909,-7.27561107942226,20.2430532997501));
#30346=CARTESIAN_POINT('Ctrl Pts',(72.1977071406346,-16.0593695431082,14.3112673566504));
#30347=CARTESIAN_POINT('Ctrl Pts',(72.3165620043785,-20.9441518794822,4.90491850337913));
#30348=CARTESIAN_POINT('Ctrl Pts',(72.4354168681221,-20.7440055724437,-5.69227162792107));
#30349=CARTESIAN_POINT('Ctrl Pts',(72.554271731866,-15.5075231692293,-14.907462850245));
#30350=CARTESIAN_POINT('Ctrl Pts',(72.6731265956095,-6.50604473249943,-20.5033437617947));
#30351=CARTESIAN_POINT('Ctrl Pts',(72.7919814593534,4.07500462245026,-21.1213176862293));
#30352=CARTESIAN_POINT('Ctrl Pts',(72.910836323097,13.6667034491012,-16.6113497437727));
#30353=CARTESIAN_POINT('Ctrl Pts',(73.0296911868409,19.9403298978757,-8.06839308905427));
#30354=CARTESIAN_POINT('Ctrl Pts',(73.1485460505845,21.3727407538559,2.43344943322881));
#30355=CARTESIAN_POINT('Ctrl Pts',(73.2674009143284,17.616167960707,12.3444866177486));
#30356=CARTESIAN_POINT('Ctrl Pts',(73.386255778072,9.58265153355406,19.2584660100977));
#30357=CARTESIAN_POINT('Ctrl Pts',(73.5051106418158,-0.777390194942946,
21.4967762225042));
#30358=CARTESIAN_POINT('Ctrl Pts',(73.6239655055596,-10.9486931436546,18.5159888183619));
#30359=CARTESIAN_POINT('Ctrl Pts',(73.7428203693032,-18.4618162006971,11.0397946560292));
#30360=CARTESIAN_POINT('Ctrl Pts',(73.861675233047,-21.4926848055884,0.883302509473593));
#30361=CARTESIAN_POINT('Ctrl Pts',(73.9805300967907,-19.3054491291201,-9.48764235195281));
#30362=CARTESIAN_POINT('Ctrl Pts',(74.0993849605345,-12.4311374700347,-17.5551287285714));
#30363=CARTESIAN_POINT('Ctrl Pts',(74.2182398242782,-2.53873048031433,-21.3604908891143));
#30364=CARTESIAN_POINT('Ctrl Pts',(74.3370946880219,7.97004251990571,-19.9798434855358));
#30365=CARTESIAN_POINT('Ctrl Pts',(74.4559495517657,16.5438077083086,-13.7483871776337));
#30366=CARTESIAN_POINT('Ctrl Pts',(74.5748044155094,21.1009823863315,-4.17902689717862));
#30367=CARTESIAN_POINT('Ctrl Pts',(74.6936592792532,20.535152305899,6.40493897310086));
#30368=CARTESIAN_POINT('Ctrl Pts',(74.8125141429969,14.9836925968255,15.4338809001317));
#30369=CARTESIAN_POINT('Ctrl Pts',(74.9313690067407,5.79441512802099,20.7157060415467));
#30370=CARTESIAN_POINT('Ctrl Pts',(75.0502238704844,-4.80166017274356,20.9680657920826));
#30371=CARTESIAN_POINT('Ctrl Pts',(75.1690787342281,-14.2319637827367,16.1296909568189));
#30372=CARTESIAN_POINT('Ctrl Pts',(75.2879335979719,-20.2069582110894,7.37526700065154));
#30373=CARTESIAN_POINT('Ctrl Pts',(75.4067884617155,-21.2760036568783,-3.16976211538219));
#30374=CARTESIAN_POINT('Ctrl Pts',(75.5256433254593,-17.1795517822342,-12.9452201231631));
#30375=CARTESIAN_POINT('Ctrl Pts',(75.644498189203,-8.91216018937456,-19.577771176376));
#30376=CARTESIAN_POINT('Ctrl Pts',(75.7633530529468,1.51897137645698,-21.457130503241));
#30377=CARTESIAN_POINT('Ctrl Pts',(75.8822079166905,11.5813192787095,-18.1270176046752));
#30378=CARTESIAN_POINT('Ctrl Pts',(76.0010627804343,18.8318950706527,-10.3959343747228));
#30379=CARTESIAN_POINT('Ctrl Pts',(76.119917644178,21.5103667637752,-0.140872862849453));
#30380=CARTESIAN_POINT('Ctrl Pts',(76.2387725079217,18.9664412590155,10.1483904853886));
#30381=CARTESIAN_POINT('Ctrl Pts',(76.3576273716655,11.8177458415602,17.9737755271368));
#30382=CARTESIAN_POINT('Ctrl Pts',(76.4764822354092,1.79987745992357,21.4353951352633));
#30383=CARTESIAN_POINT('Ctrl Pts',(76.595337099153,-8.65497440537299,19.692819542106));
#30384=CARTESIAN_POINT('Ctrl Pts',(76.7141919628966,-17.0085271817818,13.1691201901343));
#30385=CARTESIAN_POINT('Ctrl Pts',(76.8330468266405,-21.2326624698831,3.44815427665745));
#30386=CARTESIAN_POINT('Ctrl Pts',(76.9519016903841,-20.301823033284,-7.10997222222639));
#30387=CARTESIAN_POINT('Ctrl Pts',(77.0707565541279,-14.4420028459023,-15.9419031885959));
#30388=CARTESIAN_POINT('Ctrl Pts',(77.1896114178716,-5.07587911555805,-20.9033771118414));
#30389=CARTESIAN_POINT('Ctrl Pts',(77.3084662816153,5.52259258732379,-20.7898218989497));
#30390=CARTESIAN_POINT('Ctrl Pts',(77.4273211453592,14.7802609292115,-15.6288070670808));
#30391=CARTESIAN_POINT('Ctrl Pts',(77.5461760091027,20.4495016953003,-6.67335027475135));
#30392=CARTESIAN_POINT('Ctrl Pts',(77.6650308728467,21.1539075274039,3.90229673367615));
#30393=CARTESIAN_POINT('Ctrl Pts',(77.7838857365902,16.7224591637799,13.5305241210874));
#30394=CARTESIAN_POINT('Ctrl Pts',(77.9027406003341,8.23104637287821,19.8737414465204));
#30395=CARTESIAN_POINT('Ctrl Pts',(78.0215954640777,-2.25874208429753,21.3919098649989));
#30396=CARTESIAN_POINT('Ctrl Pts',(78.1404503278216,-12.2001415501875,17.7164406592014));
#30397=CARTESIAN_POINT('Ctrl Pts',(78.2593051915652,-19.1795280599448,9.73968309922879));
#30398=CARTESIAN_POINT('Ctrl Pts',(78.378160055309,-21.5024103502743,-0.601724691223848));
#30399=CARTESIAN_POINT('Ctrl Pts',(78.4970149190527,-18.6048271416103,-10.7970426741036));
#30400=CARTESIAN_POINT('Ctrl Pts',(78.6158697827966,-11.1902685508688,-18.3709992443266));
#30401=CARTESIAN_POINT('Ctrl Pts',(78.7347246465401,-1.05887915173673,-21.4847503689857));
#30402=CARTESIAN_POINT('Ctrl Pts',(78.8535795102839,9.32959036023836,-19.3823235755097));
#30403=CARTESIAN_POINT('Ctrl Pts',(78.9724343740277,17.4529740608107,-12.5741568269321));
#30404=CARTESIAN_POINT('Ctrl Pts',(79.0912892377714,21.3390351796321,-2.7131717745173));
#30405=CARTESIAN_POINT('Ctrl Pts',(79.2101441015152,20.0442958615546,7.80653104074255));
#30406=CARTESIAN_POINT('Ctrl Pts',(79.3289989652589,13.8830995606427,16.430924199962));
#30407=CARTESIAN_POINT('Ctrl Pts',(79.4478538290026,4.35129312371388,21.0661332860859));
#30408=CARTESIAN_POINT('Ctrl Pts',(79.5667086927464,-6.23694258129774,20.5867984570989));
#30409=CARTESIAN_POINT('Ctrl Pts',(79.6855635564901,-15.3109413689372,15.1092950819216));
#30410=CARTESIAN_POINT('Ctrl Pts',(79.8044184202338,-20.6676712610629,5.96347953130122));
#30411=CARTESIAN_POINT('Ctrl Pts',(79.9232732839776,-21.0065978927488,-4.63018017446131));
#30412=CARTESIAN_POINT('Ctrl Pts',(80.0421281477213,-16.2454349175536,-14.099700983182));
#30413=CARTESIAN_POINT('Ctrl Pts',(80.160983011465,-7.54012190886456,-20.1460240512879));
#30414=CARTESIAN_POINT('Ctrl Pts',(80.2798378752088,2.99582058006459,-21.3011920447583));
#30415=CARTESIAN_POINT('Ctrl Pts',(80.3986927389524,12.8044223790604,-17.2847473517617));
#30416=CARTESIAN_POINT('Ctrl Pts',(80.5175476026964,19.5043008221382,-9.07182302049318));
#30417=CARTESIAN_POINT('Ctrl Pts',(80.6364024664399,21.4688250483962,1.34360504500695));
#30418=CARTESIAN_POINT('Ctrl Pts',(80.7552573301838,18.2210377875538,11.4328257845622));
#30419=CARTESIAN_POINT('Ctrl Pts',(80.8741121939274,10.5494534929724,18.7463264261355));
#30420=CARTESIAN_POINT('Ctrl Pts',(80.9929670576712,0.316618757339831,21.5084977633984));
#30421=CARTESIAN_POINT('Ctrl Pts',(81.111821921415,-9.99308630455384,19.048725668279));
#30422=CARTESIAN_POINT('Ctrl Pts',(81.2306767851586,-17.87661860574,11.964206229438));
#30423=CARTESIAN_POINT('Ctrl Pts',(81.3495316489024,-21.4199737291271,1.9749554220587));
#30424=CARTESIAN_POINT('Ctrl Pts',(81.4683865126461,-19.7628777393287,-8.49378519483287));
#30425=CARTESIAN_POINT('Ctrl Pts',(81.5872413763899,-13.3076489021735,-16.9003610663233));
#30426=CARTESIAN_POINT('Ctrl Pts',(81.7060962401336,-3.62152079210815,-21.2037805739435));
#30427=CARTESIAN_POINT('Ctrl Pts',(81.8249511038774,6.94385871541021,-20.3592374517327));
#30428=CARTESIAN_POINT('Ctrl Pts',(81.943805967621,15.8233725798136,-14.5717742116742));
#30429=CARTESIAN_POINT('Ctrl Pts',(82.0626608313649,20.8612068703929,-5.24650087070311));
#30430=CARTESIAN_POINT('Ctrl Pts',(82.1815156951085,20.8342503324003,5.35254486786322));
#30431=CARTESIAN_POINT('Ctrl Pts',(82.3003705588522,15.7490476124256,14.6520723031646));
#30432=CARTESIAN_POINT('Ctrl Pts',(82.4192254225961,6.84021031551958,20.3942944549468));
#30433=CARTESIAN_POINT('Ctrl Pts',(82.5380802863397,-3.72932833422693,21.1850851697874));
#30434=CARTESIAN_POINT('Ctrl Pts',(82.6569351500835,-13.3934415183581,16.8324522209313));
#30435=CARTESIAN_POINT('Ctrl Pts',(82.7757900138273,-19.8058262580784,8.39315016608327));
#30436=CARTESIAN_POINT('Ctrl Pts',(82.8946448775708,-21.4096508887207,-2.08388394559674));
#30437=CARTESIAN_POINT('Ctrl Pts',(83.0134997413149,-17.8155306383307,-12.0549820219822));
#30438=CARTESIAN_POINT('Ctrl Pts',(83.1323546050583,-9.89606446026975,-19.099309717207));
#30439=CARTESIAN_POINT('Ctrl Pts',(83.2512094688023,0.42601901739055,-21.5066090137993));
#30440=CARTESIAN_POINT('Ctrl Pts',(83.3700643325459,10.6446714123967,-18.692423438327));
#30441=CARTESIAN_POINT('Ctrl Pts',(83.4889191962897,18.2789558713762,-11.3399954024637));
#30442=CARTESIAN_POINT('Ctrl Pts',(83.6077740600334,21.475381647088,-1.23438510503342));
#30443=CARTESIAN_POINT('Ctrl Pts',(83.726628923777,19.4579040910317,9.17091554098207));
#30444=CARTESIAN_POINT('Ctrl Pts',(83.8454837875209,12.7163367545633,17.3496542622657));
#30445=CARTESIAN_POINT('Ctrl Pts',(83.9643386512646,2.88743194199966,21.3161549125525));
#30446=CARTESIAN_POINT('Ctrl Pts',(84.0831935150084,-7.64249841088016,20.1074101145649));
#30447=CARTESIAN_POINT('Ctrl Pts',(84.202048378752,-16.3169437911367,14.016885131601));
#30448=CARTESIAN_POINT('Ctrl Pts',(84.3209032424959,-21.0298778467078,4.52326886534082));
#30449=CARTESIAN_POINT('Ctrl Pts',(84.4397581062395,-20.6370702687422,-6.0685298218443));
#30450=CARTESIAN_POINT('Ctrl Pts',(84.5586129699834,-15.233888896245,-15.1869797054081));
#30451=CARTESIAN_POINT('Ctrl Pts',(84.677467833727,-6.13214582285781,-20.618256742092));
#30452=CARTESIAN_POINT('Ctrl Pts',(84.7963226974707,4.45839107324696,-21.043727628764));
#30453=CARTESIAN_POINT('Ctrl Pts',(84.9151775612146,13.966496911635,-16.360094360758));
#30454=CARTESIAN_POINT('Ctrl Pts',(85.0340324249581,20.0837449772775,-7.70447345139769));
#30455=CARTESIAN_POINT('Ctrl Pts',(85.1528872887021,21.324958401384,2.82167904887415));
#30456=CARTESIAN_POINT('Ctrl Pts',(85.2717421524456,17.388789021033,12.662769833556));
#30457=CARTESIAN_POINT('Ctrl Pts',(85.3905970161895,9.23088023217779,19.4295283940399));
#30458=CARTESIAN_POINT('Ctrl Pts',(85.5094518799331,-1.1681490167756,21.4790863714037));
#30459=CARTESIAN_POINT('Ctrl Pts',(85.628306743677,-11.2835690544629,18.3138415650235));
#30460=CARTESIAN_POINT('Ctrl Pts',(85.7471616074206,-18.6595063088358,10.7022683476975));
#30461=CARTESIAN_POINT('Ctrl Pts',(85.8660164711644,-21.5051928923911,0.492343514901928));
#30462=CARTESIAN_POINT('Ctrl Pts',(85.9848713349081,-19.1297384171023,-9.83711500231921));
#30463=CARTESIAN_POINT('Ctrl Pts',(86.1037261986519,-12.1098679073116,-17.7782682717715));
#30464=CARTESIAN_POINT('Ctrl Pts',(86.2225810623956,-2.14990153953807,-21.4031223620739));
#30465=CARTESIAN_POINT('Ctrl Pts',(86.3414359261394,8.33202895367829,-19.8316166005366));
#30466=CARTESIAN_POINT('Ctrl Pts',(86.4602907898831,16.7910667115815,-13.4452892182666));
#30467=CARTESIAN_POINT('Ctrl Pts',(86.5791456536268,21.1734831497732,-3.79464554100704));
#30468=CARTESIAN_POINT('Ctrl Pts',(86.6980005173705,20.4152927222094,6.77728164842781));
#30469=CARTESIAN_POINT('Ctrl Pts',(86.8168553811144,14.7005727906504,15.7037856296628));
#30470=CARTESIAN_POINT('Ctrl Pts',(86.9357102448579,5.41677237839747,20.8176439703498));
#30471=CARTESIAN_POINT('Ctrl Pts',(87.0545651086018,-5.18213982163527,20.8772879068292));
#30472=CARTESIAN_POINT('Ctrl Pts',(87.1734199723454,-14.522905529758,15.8682367782101));
#30473=CARTESIAN_POINT('Ctrl Pts',(87.2922748360894,-20.3377257262755,7.00661371551234));
#30474=CARTESIAN_POINT('Ctrl Pts',(87.4111296998329,-21.2148485320136,-3.55611097117801));
#30475=CARTESIAN_POINT('Ctrl Pts',(87.5299845635768,-16.9413215722784,-13.2554647923137));
#30476=CARTESIAN_POINT('Ctrl Pts',(87.6488394273203,-8.55469364689703,-19.7365888664518));
#30477=CARTESIAN_POINT('Ctrl Pts',(87.7676942910644,1.9088866903574,-21.4259626406608));
#30478=CARTESIAN_POINT('Ctrl Pts',(87.8865491548077,11.9090177237354,-17.9134312830168));
#30479=CARTESIAN_POINT('Ctrl Pts',(88.0054040185518,19.0178163371241,-10.0517851769242));
#30480=CARTESIAN_POINT('Ctrl Pts',(88.1242588822953,21.5093719327835,0.250284903254255));
#30481=CARTESIAN_POINT('Ctrl Pts',(88.2431137460391,18.7787718607328,10.4915895305791));
#30482=CARTESIAN_POINT('Ctrl Pts',(88.3619686097829,11.4889652153043,18.1856922265052));
#30483=CARTESIAN_POINT('Ctrl Pts',(88.4808234735266,1.40980865288631,21.4645792653335));
#30484=CARTESIAN_POINT('Ctrl Pts',(88.5996783372704,-9.01162848704484,19.5321856300632));
#30485=CARTESIAN_POINT('Ctrl Pts',(88.718533201014,-17.2451762303881,12.8576677612322));
#30486=CARTESIAN_POINT('Ctrl Pts',(88.8373880647578,-21.2918516153265,3.06149934946342));
#30487=CARTESIAN_POINT('Ctrl Pts',(88.9562429285016,-20.1691820311599,-7.47795558088412));
#30488=CARTESIAN_POINT('Ctrl Pts',(89.0750977922452,-14.1497349592255,-16.2018740909179));
#30489=CARTESIAN_POINT('Ctrl Pts',(89.193952655989,-4.69494264122567,-20.9922184886523));
#30490=CARTESIAN_POINT('Ctrl Pts',(89.3128075197327,5.89971193763708,-20.6859643845647));
#30491=CARTESIAN_POINT('Ctrl Pts',(89.4316623834766,15.0620041851155,-15.3574657225257));
#30492=CARTESIAN_POINT('Ctrl Pts',(89.5505172472201,20.567465783262,-6.30040274203012));
#30493=CARTESIAN_POINT('Ctrl Pts',(89.669372110964,21.0794525218052,4.28630433590113));
#30494=CARTESIAN_POINT('Ctrl Pts',(89.7882269747077,16.4736616311866,13.8323604636127));
#30495=CARTESIAN_POINT('Ctrl Pts',(89.9070818384515,7.86831065794818,20.0201251407266));
#30496=CARTESIAN_POINT('Ctrl Pts',(90.0259367021951,-2.64734915020205,21.3473011519015));
#30497=CARTESIAN_POINT('Ctrl Pts',(90.1447915659389,-12.5202719372362,17.4916698213115));
#30498=CARTESIAN_POINT('Ctrl Pts',(90.2636464296827,-19.3534588953509,9.3893212514328));
#30499=CARTESIAN_POINT('Ctrl Pts',(90.3825012934263,-21.4879137644521,-0.992615094135966));
#30500=CARTESIAN_POINT('Ctrl Pts',(90.5013561571702,-18.4054227864468,-11.1335588771404));
#30501=CARTESIAN_POINT('Ctrl Pts',(90.6202110209139,-10.8543686492063,-18.5714408594927));
#30502=CARTESIAN_POINT('Ctrl Pts',(90.7390658846576,-0.668035577497034,
-21.5004516936536));
#30503=CARTESIAN_POINT('Ctrl Pts',(90.8579207484013,9.68048733122125,-19.2094754294223));
#30504=CARTESIAN_POINT('Ctrl Pts',(90.976775612145,17.6787304222826,-12.2547185323268));
#30505=CARTESIAN_POINT('Ctrl Pts',(91.0956304758889,21.3848434734381,-2.32470928089896));
#30506=CARTESIAN_POINT('Ctrl Pts',(91.2144853396325,19.8990289531884,8.16972659921727));
#30507=CARTESIAN_POINT('Ctrl Pts',(91.3333402033763,13.5820370284732,16.6806315233889));
#30508=CARTESIAN_POINT('Ctrl Pts',(91.45219506712,3.96750698263957,21.1418113192306));
#30509=CARTESIAN_POINT('Ctrl Pts',(91.5710499308638,-6.61023251764766,20.4699082394197));
#30510=CARTESIAN_POINT('Ctrl Pts',(91.6899047946075,-15.5831888969001,14.8285411378826));
#30511=CARTESIAN_POINT('Ctrl Pts',(91.8087596583512,-20.7726154886153,5.58638443685941));
#30512=CARTESIAN_POINT('Ctrl Pts',(91.927614522095,-20.91908085082,-5.01079536286535));
#30513=CARTESIAN_POINT('Ctrl Pts',(92.0464693858386,-15.9860728998834,-14.3940251993155));
#30514=CARTESIAN_POINT('Ctrl Pts',(92.1257059616679,-10.110761492509,-18.3154926834751));
#30515=CARTESIAN_POINT('Ctrl Pts',(92.1653242495824,-6.88173117344805,-19.457534527244));
#30516=CARTESIAN_POINT('Ctrl Pts',(68.5596757504176,11.8154297096169,-16.5714132187663));
#30517=CARTESIAN_POINT('Ctrl Pts',(68.5992940383321,14.5655004155514,-14.610610799957));
#30518=CARTESIAN_POINT('Ctrl Pts',(68.6785306141613,19.0679034391389,-9.29548417524227));
#30519=CARTESIAN_POINT('Ctrl Pts',(68.797385477905,21.1915289634232,0.940384474903618));
#30520=CARTESIAN_POINT('Ctrl Pts',(68.9162403416488,18.1702740300995,10.9453086963044));
#30521=CARTESIAN_POINT('Ctrl Pts',(69.0350952053925,10.7375060596412,18.2941638888631));
#30522=CARTESIAN_POINT('Ctrl Pts',(69.1539500691362,0.6978507132554,21.2008167877962));
#30523=CARTESIAN_POINT('Ctrl Pts',(69.27280493288,-9.51124218235847,18.9605575668569));
#30524=CARTESIAN_POINT('Ctrl Pts',(69.3916597966237,-17.4111419435958,12.1167885812654));
#30525=CARTESIAN_POINT('Ctrl Pts',(69.5105146603675,-21.0838778623392,2.33132912871676));
#30526=CARTESIAN_POINT('Ctrl Pts',(69.6293695241111,-19.6377604631667,-8.02018593076447));
#30527=CARTESIAN_POINT('Ctrl Pts',(69.748224387855,-13.4238874837994,-16.4244969435884));
#30528=CARTESIAN_POINT('Ctrl Pts',(69.8670792515985,-3.95089390015628,-20.8411955990666));
#30529=CARTESIAN_POINT('Ctrl Pts',(69.9859341153425,6.48131780491308,-20.1979561300039));
#30530=CARTESIAN_POINT('Ctrl Pts',(70.1047889790861,15.3399620080666,-14.6509561673825));
#30531=CARTESIAN_POINT('Ctrl Pts',(70.2236438428299,20.4742914923196,-5.5469204181725));
#30532=CARTESIAN_POINT('Ctrl Pts',(70.3424987065737,20.637767470736,4.90382437254567));
#30533=CARTESIAN_POINT('Ctrl Pts',(70.4613535703173,15.7907003730259,14.1639939080515));
#30534=CARTESIAN_POINT('Ctrl Pts',(70.5802084340611,7.10988603323194,19.985356141388));
#30535=CARTESIAN_POINT('Ctrl Pts',(70.6990632978048,-3.29710291659937,20.9545711789422));
#30536=CARTESIAN_POINT('Ctrl Pts',(70.8179181615486,-12.9036043036696,16.8363278715341));
#30537=CARTESIAN_POINT('Ctrl Pts',(70.9367730252922,-19.3773024390889,8.63047453352477));
#30538=CARTESIAN_POINT('Ctrl Pts',(71.0556278890361,-21.1464796762811,-1.67072970188107));
#30539=CARTESIAN_POINT('Ctrl Pts',(71.1744827527797,-17.7816060897448,-11.5663056022351));
#30540=CARTESIAN_POINT('Ctrl Pts',(71.2933376165235,-10.099622951387,-18.6537544930662));
#30541=CARTESIAN_POINT('Ctrl Pts',(71.4121924802672,0.0343984613121467,
-21.2123491666975));
#30542=CARTESIAN_POINT('Ctrl Pts',(71.531047344011,10.1600684391248,-18.6209008844661));
#30543=CARTESIAN_POINT('Ctrl Pts',(71.6499022077547,17.8190248769147,-11.5085747539573));
#30544=CARTESIAN_POINT('Ctrl Pts',(71.7687570714985,21.1517870378704,-1.60213780228773));
#30545=CARTESIAN_POINT('Ctrl Pts',(71.8876119352421,19.3492098264228,8.6932743846095));
#30546=CARTESIAN_POINT('Ctrl Pts',(72.006466798986,12.8489321857626,16.8780888171102));
#30547=CARTESIAN_POINT('Ctrl Pts',(72.1253216627296,3.2291248699632,20.9651542566983));
#30548=CARTESIAN_POINT('Ctrl Pts',(72.2441765264735,-7.17466594819554,19.9621919879694));
#30549=CARTESIAN_POINT('Ctrl Pts',(72.3630313902171,-15.8365545591501,14.1127063360615));
#30550=CARTESIAN_POINT('Ctrl Pts',(72.4818862539609,-20.6535632077091,4.83686543724142));
#30551=CARTESIAN_POINT('Ctrl Pts',(72.6007411177046,-20.4561938214004,-5.61329446707699));
#30552=CARTESIAN_POINT('Ctrl Pts',(72.7195959814484,-15.2923647523993,-14.7006299427066));
#30553=CARTESIAN_POINT('Ctrl Pts',(72.838450845192,-6.41577691415126,-20.2188710619723));
#30554=CARTESIAN_POINT('Ctrl Pts',(72.9573057089359,4.01846615827561,-20.8282709356206));
#30555=CARTESIAN_POINT('Ctrl Pts',(73.0761605726795,13.4770854007962,-16.3808763359127));
#30556=CARTESIAN_POINT('Ctrl Pts',(73.1950154364233,19.6636687080083,-7.95644854030465));
#30557=CARTESIAN_POINT('Ctrl Pts',(73.3138703001669,21.0762056454613,2.39968665101172));
#30558=CARTESIAN_POINT('Ctrl Pts',(73.4327251639109,17.37175324872,12.1732136060453));
#30559=CARTESIAN_POINT('Ctrl Pts',(73.5515800276544,9.44969747567559,18.991265309374));
#30560=CARTESIAN_POINT('Ctrl Pts',(73.6704348913983,-0.766604330444966,
21.1985201897058));
#30561=CARTESIAN_POINT('Ctrl Pts',(73.7892897551419,-10.7967860042978,18.2590895832793));
#30562=CARTESIAN_POINT('Ctrl Pts',(73.9081446188858,-18.2056685811062,10.8866235329299));
#30563=CARTESIAN_POINT('Ctrl Pts',(74.0269994826294,-21.1944855389658,0.871047169439829));
#30564=CARTESIAN_POINT('Ctrl Pts',(74.1458543463732,-19.0375965632729,-9.35600649459388));
#30565=CARTESIAN_POINT('Ctrl Pts',(74.2647092101169,-12.2586622250674,-17.3115609026028));
#30566=CARTESIAN_POINT('Ctrl Pts',(74.3835640738607,-2.50350698105258,-21.0641257409046));
#30567=CARTESIAN_POINT('Ctrl Pts',(74.5024189376044,7.85946253160344,-19.7026340662141));
#30568=CARTESIAN_POINT('Ctrl Pts',(74.6212738013481,16.3142714093126,-13.5576358121948));
#30569=CARTESIAN_POINT('Ctrl Pts',(74.7401286650918,20.8082177769057,-4.12104518073847));
#30570=CARTESIAN_POINT('Ctrl Pts',(74.8589835288356,20.2502382798946,6.31607394196041));
#30571=CARTESIAN_POINT('Ctrl Pts',(74.9778383925794,14.7758020431749,15.2197442295766));
#30572=CARTESIAN_POINT('Ctrl Pts',(75.096693256323,5.71402078188356,20.428286931043));
#30573=CARTESIAN_POINT('Ctrl Pts',(75.2155481200669,-4.73503975956417,20.6771453278292));
#30574=CARTESIAN_POINT('Ctrl Pts',(75.3344029838105,-14.034503055936,15.9059003016411));
#30575=CARTESIAN_POINT('Ctrl Pts',(75.4532578475543,-19.9265976989558,7.2729391979301));
#30576=CARTESIAN_POINT('Ctrl Pts',(75.5721127112981,-20.9808107228857,-3.12578339672864));
#30577=CARTESIAN_POINT('Ctrl Pts',(75.6909675750417,-16.9411948813302,-12.7656122620739));
#30578=CARTESIAN_POINT('Ctrl Pts',(75.8098224387856,-8.78850883280678,-19.3061402908116));
#30579=CARTESIAN_POINT('Ctrl Pts',(75.9286773025292,1.49789647797051,-21.1594245331508));
#30580=CARTESIAN_POINT('Ctrl Pts',(76.0475321662729,11.4206347971442,-17.8755151328033));
#30581=CARTESIAN_POINT('Ctrl Pts',(76.1663870300168,18.570612808805,-10.2516964614774));
#30582=CARTESIAN_POINT('Ctrl Pts',(76.2852418937604,21.2119221696372,-0.138918328794305));
#30583=CARTESIAN_POINT('Ctrl Pts',(76.4040967575042,18.7032922422669,10.0075871084483));
#30584=CARTESIAN_POINT('Ctrl Pts',(76.5229516212479,11.6537810705247,17.7243992054202));
#30585=CARTESIAN_POINT('Ctrl Pts',(76.6418064849917,1.7749051429043,21.1379907315363));
#30586=CARTESIAN_POINT('Ctrl Pts',(76.7606613487353,-8.53489136113423,19.4195924232837));
#30587=CARTESIAN_POINT('Ctrl Pts',(76.8795162124791,-16.7725431538293,12.9864058378659));
#30588=CARTESIAN_POINT('Ctrl Pts',(76.9983710762229,-20.9380708711956,3.4003130187689));
#30589=CARTESIAN_POINT('Ctrl Pts',(77.1172259399666,-20.0201463235389,-7.01132523970409));
#30590=CARTESIAN_POINT('Ctrl Pts',(77.2360808037103,-14.2416279417819,-15.7207179861697));
#30591=CARTESIAN_POINT('Ctrl Pts',(77.3549356674541,-5.00545406427125,-20.6133541677062));
#30592=CARTESIAN_POINT('Ctrl Pts',(77.4737905311978,5.44596963052285,-20.501374471392));
#30593=CARTESIAN_POINT('Ctrl Pts',(77.5926453949415,14.5751928788749,-15.4119659023894));
#30594=CARTESIAN_POINT('Ctrl Pts',(77.7115002586853,20.1657760247526,-6.58076118335362));
#30595=CARTESIAN_POINT('Ctrl Pts',(77.8303551224291,20.8604086105429,3.84815449715933));
#30596=CARTESIAN_POINT('Ctrl Pts',(77.9492099861727,16.4904441733833,13.3427954866044));
#30597=CARTESIAN_POINT('Ctrl Pts',(78.0680648499165,8.11684509862461,19.5980041350581));
#30598=CARTESIAN_POINT('Ctrl Pts',(78.1869197136602,-2.22740327115626,21.0951087956537));
#30599=CARTESIAN_POINT('Ctrl Pts',(78.305774577404,-12.0308712474838,17.4706347182719));
#30600=CARTESIAN_POINT('Ctrl Pts',(78.4246294411476,-18.9134225801791,9.60455031411619));
#30601=CARTESIAN_POINT('Ctrl Pts',(78.5434843048915,-21.2040761470294,-0.593376089676207));
#30602=CARTESIAN_POINT('Ctrl Pts',(78.6623391686352,-18.3466953232985,-10.6472396022104));
#30603=CARTESIAN_POINT('Ctrl Pts',(78.7811940323789,-11.0350096846377,-18.1161116604191));
#30604=CARTESIAN_POINT('Ctrl Pts',(78.9000488961227,-1.04418778165678,-21.1866611883387));
#30605=CARTESIAN_POINT('Ctrl Pts',(79.0189037598663,9.2001473879677,-19.1134044186924));
#30606=CARTESIAN_POINT('Ctrl Pts',(79.1377586236102,17.2108235750806,-12.3996972664767));
#30607=CARTESIAN_POINT('Ctrl Pts',(79.2566134873538,21.0429677176766,-2.67552799754383));
#30608=CARTESIAN_POINT('Ctrl Pts',(79.3754683510976,19.7661922007068,7.69821968493602));
#30609=CARTESIAN_POINT('Ctrl Pts',(79.4943232148413,13.6904791344428,16.2029540980096));
#30610=CARTESIAN_POINT('Ctrl Pts',(79.6131780785851,4.29092130743831,20.7738521888983));
#30611=CARTESIAN_POINT('Ctrl Pts',(79.7320329423288,-6.15040840836714,20.3011678689456));
#30612=CARTESIAN_POINT('Ctrl Pts',(79.8508878060725,-15.0985104172522,14.8996618623695));
#30613=CARTESIAN_POINT('Ctrl Pts',(79.9697426698163,-20.3809186069113,5.88073950887784));
#30614=CARTESIAN_POINT('Ctrl Pts',(80.08859753356,-20.7151428166373,-4.56593895262964));
#30615=CARTESIAN_POINT('Ctrl Pts',(80.2074523973038,-16.0200383781171,-13.9040753305092));
#30616=CARTESIAN_POINT('Ctrl Pts',(80.3263072610475,-7.43550683430282,-19.8665089673515));
#30617=CARTESIAN_POINT('Ctrl Pts',(80.4451621247912,2.9542552052411,-21.0056496356368));
#30618=CARTESIAN_POINT('Ctrl Pts',(80.564016988535,12.6267680097947,-17.0449309197675));
#30619=CARTESIAN_POINT('Ctrl Pts',(80.6828718522787,19.2336892976239,-8.94595642931989));
#30620=CARTESIAN_POINT('Ctrl Pts',(80.8017267160225,21.1709568228772,1.32496325861892));
#30621=CARTESIAN_POINT('Ctrl Pts',(80.9205815797661,17.9682308369797,11.2742015691503));
#30622=CARTESIAN_POINT('Ctrl Pts',(81.03943644351,10.403085585783,18.4862313825099));
#30623=CARTESIAN_POINT('Ctrl Pts',(81.1582913072536,0.312225844956285,21.2100791006201));
#30624=CARTESIAN_POINT('Ctrl Pts',(81.2771461709974,-9.85443768832609,18.7844350002794));
#30625=CARTESIAN_POINT('Ctrl Pts',(81.3960010347411,-17.6285902832599,11.7982094004884));
#30626=CARTESIAN_POINT('Ctrl Pts',(81.5148558984849,-21.12278328899,1.9475539939078));
#30627=CARTESIAN_POINT('Ctrl Pts',(81.6337107622286,-19.4886786012718,-8.37593856288069));
#30628=CARTESIAN_POINT('Ctrl Pts',(81.7525656259724,-13.1230125396625,-16.6658777841638));
#30629=CARTESIAN_POINT('Ctrl Pts',(81.871420489716,-3.57127416847624,-20.9095896957926));
#30630=CARTESIAN_POINT('Ctrl Pts',(81.9902753534598,6.8475164670966,-20.07676414828));
#30631=CARTESIAN_POINT('Ctrl Pts',(82.1091302172036,15.6038319248663,-14.3695988007092));
#30632=CARTESIAN_POINT('Ctrl Pts',(82.2279850809473,20.5717690153327,-5.17370853572354));
#30633=CARTESIAN_POINT('Ctrl Pts',(82.346839944691,20.5451864845865,5.27828123032336));
#30634=CARTESIAN_POINT('Ctrl Pts',(82.4656948084347,15.5305381758191,14.4487828000231));
#30635=CARTESIAN_POINT('Ctrl Pts',(82.5845496721784,6.74530613216218,20.1113347547157));
#30636=CARTESIAN_POINT('Ctrl Pts',(82.7034045359223,-3.67758593981133,20.8911536801614));
#30637=CARTESIAN_POINT('Ctrl Pts',(82.8222593996659,-13.2076148301405,16.5989111369232));
#30638=CARTESIAN_POINT('Ctrl Pts',(82.9411142634097,-19.5310312327739,8.27669979020799));
#30639=CARTESIAN_POINT('Ctrl Pts',(83.0599691271534,-21.1126036723579,-2.05497119365699));
#30640=CARTESIAN_POINT('Ctrl Pts',(83.1788239908972,-17.5683498780442,-11.887725728475));
#30641=CARTESIAN_POINT('Ctrl Pts',(83.2976788546409,-9.75876196915726,-18.8343172231475));
#30642=CARTESIAN_POINT('Ctrl Pts',(83.4165337183847,0.420108236131625,-21.2082165563905));
#30643=CARTESIAN_POINT('Ctrl Pts',(83.5353885821283,10.4969824085646,-18.4330762692261));
#30644=CARTESIAN_POINT('Ctrl Pts',(83.6542434458721,18.0253453390124,-11.1826591579179));
#30645=CARTESIAN_POINT('Ctrl Pts',(83.7730983096158,21.1774224523421,-1.21725868567815));
#30646=CARTESIAN_POINT('Ctrl Pts',(83.8919531733597,19.1879362958286,9.04367409519178));
#30647=CARTESIAN_POINT('Ctrl Pts',(84.0108080371033,12.5399045252426,17.1089372823276));
#30648=CARTESIAN_POINT('Ctrl Pts',(84.1296629008471,2.84737040034882,21.02040490181));
#30649=CARTESIAN_POINT('Ctrl Pts',(84.2485177645907,-7.5364629182508,19.8284307779171));
#30650=CARTESIAN_POINT('Ctrl Pts',(84.3673726283346,-16.0905551051233,13.8224085036513));
#30651=CARTESIAN_POINT('Ctrl Pts',(84.4862274920782,-20.7380997739461,4.46051097954932));
#30652=CARTESIAN_POINT('Ctrl Pts',(84.605082355822,-20.3507421866508,-5.98433228399736));
#30653=CARTESIAN_POINT('Ctrl Pts',(84.7239372195658,-15.0225270055477,-14.9762686541211));
#30654=CARTESIAN_POINT('Ctrl Pts',(84.8427920833094,-6.04706564773123,-20.3321896874107));
#30655=CARTESIAN_POINT('Ctrl Pts',(84.9616469470532,4.39653333139736,-20.7517573978382));
#30656=CARTESIAN_POINT('Ctrl Pts',(85.0805018107969,13.7727193927253,-16.1331069841513));
#30657=CARTESIAN_POINT('Ctrl Pts',(85.1993566745408,19.8050939814884,-7.59757808891962));
#30658=CARTESIAN_POINT('Ctrl Pts',(85.3182115382844,21.0290862470408,2.78252979271425));
#30659=CARTESIAN_POINT('Ctrl Pts',(85.4370664020282,17.1475290676846,12.4870808160166));
#30660=CARTESIAN_POINT('Ctrl Pts',(85.5559212657719,9.102806809038,19.1599542961395));
#30661=CARTESIAN_POINT('Ctrl Pts',(85.6747761295157,-1.15194158697989,21.1810757756306));
#30662=CARTESIAN_POINT('Ctrl Pts',(85.7936309932593,-11.1270156946867,18.0597470127081));
#30663=CARTESIAN_POINT('Ctrl Pts',(85.9124858570031,-18.4006158469338,10.5537802178361));
#30664=CARTESIAN_POINT('Ctrl Pts',(86.0313407207469,-21.2068200828936,0.485512517453323));
#30665=CARTESIAN_POINT('Ctrl Pts',(86.1501955844905,-18.8643237414458,-9.70063040274928));
#30666=CARTESIAN_POINT('Ctrl Pts',(86.2690504482344,-11.9418501021132,-17.5316045064757));
#30667=CARTESIAN_POINT('Ctrl Pts',(86.387905311978,-2.12007282952809,-21.1061657254537));
#30668=CARTESIAN_POINT('Ctrl Pts',(86.5067601757219,8.21642660125285,-19.5564637483121));
#30669=CARTESIAN_POINT('Ctrl Pts',(86.6256150394655,16.558099828919,-13.2587431715217));
#30670=CARTESIAN_POINT('Ctrl Pts',(86.7444699032093,20.8797126318402,-3.74199690601068));
#30671=CARTESIAN_POINT('Ctrl Pts',(86.863324766953,20.1320416824852,6.68325056596715));
#30672=CARTESIAN_POINT('Ctrl Pts',(86.9821796306968,14.4966103697264,15.485904178354));
#30673=CARTESIAN_POINT('Ctrl Pts',(87.1010344944404,5.34161761921727,20.5288105267424));
#30674=CARTESIAN_POINT('Ctrl Pts',(87.2198893581843,-5.11024046107027,20.5876269361687));
#30675=CARTESIAN_POINT('Ctrl Pts',(87.3387442219279,-14.3214081450722,15.6480736570059));
#30676=CARTESIAN_POINT('Ctrl Pts',(87.4575990856717,-20.0555508862681,6.90940077583666));
#30677=CARTESIAN_POINT('Ctrl Pts',(87.5764539494153,-20.9205040919877,-3.50677187309764));
#30678=CARTESIAN_POINT('Ctrl Pts',(87.6953088131592,-16.7062699854633,-13.0715524558344));
#30679=CARTESIAN_POINT('Ctrl Pts',(87.8141636769028,-8.43600194342856,-19.4627544721524));
#30680=CARTESIAN_POINT('Ctrl Pts',(87.9330185406467,1.88240192978519,-21.1286891076461));
#30681=CARTESIAN_POINT('Ctrl Pts',(88.0518734043902,11.7437866051695,-17.6648922047393));
#30682=CARTESIAN_POINT('Ctrl Pts',(88.1707282681343,18.7539545192176,-9.91232214589198));
#30683=CARTESIAN_POINT('Ctrl Pts',(88.2895831318777,21.2109411413823,0.24681233687776));
#30684=CARTESIAN_POINT('Ctrl Pts',(88.4084379956217,18.5182266544175,10.3460244542741));
#30685=CARTESIAN_POINT('Ctrl Pts',(88.5272928593653,11.3295620959432,17.9333756762919));
#30686=CARTESIAN_POINT('Ctrl Pts',(88.6461477231091,1.39024832758623,21.1667699477362));
#30687=CARTESIAN_POINT('Ctrl Pts',(88.7650025868527,-8.88659706215682,19.261187219064));
#30688=CARTESIAN_POINT('Ctrl Pts',(88.8838574505966,-17.0059088260971,12.6792746413611));
#30689=CARTESIAN_POINT('Ctrl Pts',(89.0027123143402,-20.9964387995634,3.01902271757524));
#30690=CARTESIAN_POINT('Ctrl Pts',(89.1215671780841,-19.889345642897,-7.37420303018019));
#30691=CARTESIAN_POINT('Ctrl Pts',(89.2404220418276,-13.9534151124538,-15.9770819341667));
#30692=CARTESIAN_POINT('Ctrl Pts',(89.3592769055716,-4.62980287552805,-20.7009629189214));
#30693=CARTESIAN_POINT('Ctrl Pts',(89.4781317693152,5.81785665575857,-20.3989579233126));
#30694=CARTESIAN_POINT('Ctrl Pts',(89.5969866330589,14.8530271009356,-15.144389270837));
#30695=CARTESIAN_POINT('Ctrl Pts',(89.7158414968027,20.2821034254025,-6.21298809401871));
#30696=CARTESIAN_POINT('Ctrl Pts',(89.8346963605464,20.7869866274943,4.22683420357247));
#30697=CARTESIAN_POINT('Ctrl Pts',(89.9535512242901,16.2450985707107,13.6404440146805));
#30698=CARTESIAN_POINT('Ctrl Pts',(90.072406088034,7.7591421436847,19.7423568354331));
#30699=CARTESIAN_POINT('Ctrl Pts',(90.1912609517776,-2.61061862620169,21.051119004094));
#30700=CARTESIAN_POINT('Ctrl Pts',(90.3101158155214,-12.3465600002041,17.2489824530325));
#30701=CARTESIAN_POINT('Ctrl Pts',(90.428970679265,-19.0849402202106,9.25904954565997));
#30702=CARTESIAN_POINT('Ctrl Pts',(90.5478255430088,-21.1897806934203,-0.978843101674954));
#30703=CARTESIAN_POINT('Ctrl Pts',(90.6666804067526,-18.1500575946877,-10.9790868266686));
#30704=CARTESIAN_POINT('Ctrl Pts',(90.7855352704963,-10.7037702107086,-18.3137722576163));
#30705=CARTESIAN_POINT('Ctrl Pts',(90.9043901342401,-0.658766948608187,
-21.2021446656999));
#30706=CARTESIAN_POINT('Ctrl Pts',(91.0232449979838,9.54617585506875,-18.9429544462565));
#30707=CARTESIAN_POINT('Ctrl Pts',(91.1420998617275,17.4334476903006,-12.084691003795));
#30708=CARTESIAN_POINT('Ctrl Pts',(91.2609547254713,21.0881404464175,-2.29245520892303));
#30709=CARTESIAN_POINT('Ctrl Pts',(91.379809589215,19.6229407913781,8.0563761033425));
#30710=CARTESIAN_POINT('Ctrl Pts',(91.4986644529587,13.3935936805263,16.4491968686648));
#30711=CARTESIAN_POINT('Ctrl Pts',(91.6175193167025,3.9124599895233,20.8484802306535));
#30712=CARTESIAN_POINT('Ctrl Pts',(91.7363741804461,-6.51851915066736,20.1858994392144));
#30713=CARTESIAN_POINT('Ctrl Pts',(91.8552290441899,-15.3669806594123,14.6228032260118));
#30714=CARTESIAN_POINT('Ctrl Pts',(91.9740839079338,-20.4844067906062,5.50887640297662));
#30715=CARTESIAN_POINT('Ctrl Pts',(92.0929387716773,-20.6288400258807,-4.94127331311132));
#30716=CARTESIAN_POINT('Ctrl Pts',(92.2117936354212,-15.7642748668298,-14.1943159588457));
#30717=CARTESIAN_POINT('Ctrl Pts',(92.2910302112503,-9.97048019729925,-18.0613752227927));
#30718=CARTESIAN_POINT('Ctrl Pts',(92.3306484991649,-6.78625091085736,-19.1875718595368));
#30719=CARTESIAN_POINT('Ctrl Pts',(68.725,11.6491905967231,-16.3382590211968));
#30720=CARTESIAN_POINT('Ctrl Pts',(68.7646182879146,14.3605687349063,-14.4050444314105));
#30721=CARTESIAN_POINT('Ctrl Pts',(68.8438548637438,18.799624465765,-9.16469984651376));
#30722=CARTESIAN_POINT('Ctrl Pts',(68.9627097274874,20.8933712948219,0.927153582356417));
#30723=CARTESIAN_POINT('Ctrl Pts',(69.0815645912312,17.9146243999094,10.7913118927399));
#30724=CARTESIAN_POINT('Ctrl Pts',(69.200419454975,10.5864329691218,18.0367711701248));
#30725=CARTESIAN_POINT('Ctrl Pts',(69.3192743187187,0.688032188973571,20.9025284426369));
#30726=CARTESIAN_POINT('Ctrl Pts',(69.4381291824624,-9.37742221120445,18.6937889137184));
#30727=CARTESIAN_POINT('Ctrl Pts',(69.5569840462062,-17.1661730459504,11.9463094506391));
#30728=CARTESIAN_POINT('Ctrl Pts',(69.6758389099499,-20.7872348084396,2.29852811379418));
#30729=CARTESIAN_POINT('Ctrl Pts',(69.7946937736936,-19.3614637935703,-7.90734461841775));
#30730=CARTESIAN_POINT('Ctrl Pts',(69.9135486374375,-13.2350179122529,-16.1934098084835));
#30731=CARTESIAN_POINT('Ctrl Pts',(70.032403501181,-3.89530615487391,-20.5479670028002));
#30732=CARTESIAN_POINT('Ctrl Pts',(70.1512583649248,6.39012784832653,-19.9137776962236));
#30733=CARTESIAN_POINT('Ctrl Pts',(70.2701132286686,15.124133913895,-14.4448221531172));
#30734=CARTESIAN_POINT('Ctrl Pts',(70.3889680924123,20.1862251131474,-5.46887711782098));
#30735=CARTESIAN_POINT('Ctrl Pts',(70.5078229561561,20.3474010396572,4.83482921676092));
#30736=CARTESIAN_POINT('Ctrl Pts',(70.6266778198998,15.5685305420084,13.9647112886144));
#30737=CARTESIAN_POINT('Ctrl Pts',(70.7455326836435,7.00985233357066,19.7041689177776));
#30738=CARTESIAN_POINT('Ctrl Pts',(70.8643875473874,-3.25071379005506,20.6597474264871));
#30739=CARTESIAN_POINT('Ctrl Pts',(70.9832424111308,-12.7220549410739,16.599446414106));
#30740=CARTESIAN_POINT('Ctrl Pts',(71.1020972748749,-19.1046703260878,8.50904666627266));
#30741=CARTESIAN_POINT('Ctrl Pts',(71.2209521386184,-20.8489558359632,-1.64722309819828));
#30742=CARTESIAN_POINT('Ctrl Pts',(71.3398070023622,-17.5314248864508,-11.4035715815495));
#30743=CARTESIAN_POINT('Ctrl Pts',(71.458661866106,-9.95752466116282,-18.3913024557491));
#30744=CARTESIAN_POINT('Ctrl Pts',(71.5775167298497,0.0339144865576418,
-20.9138985648547));
#30745=CARTESIAN_POINT('Ctrl Pts',(71.6963715935934,10.017119701265,-18.3589110863466));
#30746=CARTESIAN_POINT('Ctrl Pts',(71.8152264573371,17.5683172038997,-11.3466529868452));
#30747=CARTESIAN_POINT('Ctrl Pts',(71.9340813210809,20.8541885247641,-1.57959626350904));
#30748=CARTESIAN_POINT('Ctrl Pts',(72.0529361848246,19.0769729670116,8.57096294462323));
#30749=CARTESIAN_POINT('Ctrl Pts',(72.1717910485684,12.6681520414353,16.640619797256));
#30750=CARTESIAN_POINT('Ctrl Pts',(72.2906459123121,3.18369217161882,20.670181603907));
#30751=CARTESIAN_POINT('Ctrl Pts',(72.4095007760559,-7.07372081696884,19.6813306761887));
#30752=CARTESIAN_POINT('Ctrl Pts',(72.5283556397995,-15.6137395751919,13.9141453154726));
#30753=CARTESIAN_POINT('Ctrl Pts',(72.6472105035434,-20.362974535936,4.76881237110371));
#30754=CARTESIAN_POINT('Ctrl Pts',(72.766065367287,-20.1683820703571,-5.5343173062329));
#30755=CARTESIAN_POINT('Ctrl Pts',(72.8849202310308,-15.0772063355693,-14.4937970351682));
#30756=CARTESIAN_POINT('Ctrl Pts',(73.0037750947745,-6.32550909580307,-19.9343983621499));
#30757=CARTESIAN_POINT('Ctrl Pts',(73.1226299585183,3.96192769410095,-20.5352241850118));
#30758=CARTESIAN_POINT('Ctrl Pts',(73.241484822262,13.2874673524912,-16.1504029280528));
#30759=CARTESIAN_POINT('Ctrl Pts',(73.3603396860058,19.3870075181409,-7.84450399155505));
#30760=CARTESIAN_POINT('Ctrl Pts',(73.4791945497494,20.7796705370668,2.36592386879463));
#30761=CARTESIAN_POINT('Ctrl Pts',(73.5980494134933,17.1273385367331,12.0019405943419));
#30762=CARTESIAN_POINT('Ctrl Pts',(73.7169042772369,9.31674341779712,18.7240646086503));
#30763=CARTESIAN_POINT('Ctrl Pts',(73.8357591409808,-0.75581846594697,20.9002641569074));
#30764=CARTESIAN_POINT('Ctrl Pts',(73.9546140047244,-10.6448788649411,18.0021903481967));
#30765=CARTESIAN_POINT('Ctrl Pts',(74.0734688684682,-17.9495209615153,10.7334524098305));
#30766=CARTESIAN_POINT('Ctrl Pts',(74.1923237322118,-20.8962862723432,0.858791829406043));
#30767=CARTESIAN_POINT('Ctrl Pts',(74.3111785959557,-18.7697439974256,-9.22437063723492));
#30768=CARTESIAN_POINT('Ctrl Pts',(74.4300334596993,-12.0861869801001,-17.0679930766342));
#30769=CARTESIAN_POINT('Ctrl Pts',(74.5488883234432,-2.46828348179083,-20.7677605926949));
#30770=CARTESIAN_POINT('Ctrl Pts',(74.6677431871868,7.74888254330118,-19.4254246468925));
#30771=CARTESIAN_POINT('Ctrl Pts',(74.7865980509306,16.0847351103166,-13.3668844467559));
#30772=CARTESIAN_POINT('Ctrl Pts',(74.9054529146743,20.5154531674799,-4.06306346429831));
#30773=CARTESIAN_POINT('Ctrl Pts',(75.024307778418,19.9653242538903,6.22720891081994));
#30774=CARTESIAN_POINT('Ctrl Pts',(75.1431626421618,14.5679114895243,15.0056075590215));
#30775=CARTESIAN_POINT('Ctrl Pts',(75.2620175059054,5.63362643574612,20.1408678205393));
#30776=CARTESIAN_POINT('Ctrl Pts',(75.3808723696493,-4.66841934638479,20.3862248635758));
#30777=CARTESIAN_POINT('Ctrl Pts',(75.499727233393,-13.8370423291352,15.6821096464633));
#30778=CARTESIAN_POINT('Ctrl Pts',(75.6185820971368,-19.6462371868223,7.17061139520864));
#30779=CARTESIAN_POINT('Ctrl Pts',(75.7374369608804,-20.6856177888931,-3.08180467807508));
#30780=CARTESIAN_POINT('Ctrl Pts',(75.8562918246243,-16.7028379804262,-12.5860044009848));
#30781=CARTESIAN_POINT('Ctrl Pts',(75.9751466883679,-8.66485747623899,-19.0345094052471));
#30782=CARTESIAN_POINT('Ctrl Pts',(76.0940015521117,1.47682157948402,-20.8617185630606));
#30783=CARTESIAN_POINT('Ctrl Pts',(76.2128564158554,11.2599503155789,-17.6240126609314));
#30784=CARTESIAN_POINT('Ctrl Pts',(76.3317112795992,18.3093305469575,-10.1074585482319));
#30785=CARTESIAN_POINT('Ctrl Pts',(76.4505661433428,20.9134775754992,-0.136963794739155));
#30786=CARTESIAN_POINT('Ctrl Pts',(76.5694210070867,18.4401432255183,9.86678373150789));
#30787=CARTESIAN_POINT('Ctrl Pts',(76.6882758708303,11.4898162994893,17.4750228837036));
#30788=CARTESIAN_POINT('Ctrl Pts',(76.8071307345741,1.74993282588505,20.8405863278091));
#30789=CARTESIAN_POINT('Ctrl Pts',(76.9259855983178,-8.41480831689548,19.1463653044614));
#30790=CARTESIAN_POINT('Ctrl Pts',(77.0448404620616,-16.5365591258767,12.8036914855974));
#30791=CARTESIAN_POINT('Ctrl Pts',(77.1636953258053,-20.6434792725082,3.35247176088037));
#30792=CARTESIAN_POINT('Ctrl Pts',(77.2825501895491,-19.7384696137938,-6.91267825718176));
#30793=CARTESIAN_POINT('Ctrl Pts',(77.4014050532927,-14.0412530376615,-15.4995327837435));
#30794=CARTESIAN_POINT('Ctrl Pts',(77.5202599170366,-4.93502901298443,-20.323331223571));
#30795=CARTESIAN_POINT('Ctrl Pts',(77.6391147807802,5.3693466737219,-20.2129270438343));
#30796=CARTESIAN_POINT('Ctrl Pts',(77.7579696445241,14.3701248285384,-15.1951247376979));
#30797=CARTESIAN_POINT('Ctrl Pts',(77.8768245082677,19.8820503542049,-6.48817209195593));
#30798=CARTESIAN_POINT('Ctrl Pts',(77.9956793720115,20.566909693682,3.79401226064252));
#30799=CARTESIAN_POINT('Ctrl Pts',(78.1145342357552,16.2584291829867,13.1550668521213));
#30800=CARTESIAN_POINT('Ctrl Pts',(78.2333890994989,8.002643824371,19.3222668235958));
#30801=CARTESIAN_POINT('Ctrl Pts',(78.3522439632428,-2.19606445801497,20.7983077263084));
#30802=CARTESIAN_POINT('Ctrl Pts',(78.4710988269864,-11.8616009447801,17.2248287773426));
#30803=CARTESIAN_POINT('Ctrl Pts',(78.5899536907302,-18.6473171004135,9.46941752900355));
#30804=CARTESIAN_POINT('Ctrl Pts',(78.7088085544739,-20.9057419437845,-0.585027488128542));
#30805=CARTESIAN_POINT('Ctrl Pts',(78.8276634182176,-18.0885635049867,-10.4974365303172));
#30806=CARTESIAN_POINT('Ctrl Pts',(78.9465182819614,-10.8797508184065,-17.8612240765116));
#30807=CARTESIAN_POINT('Ctrl Pts',(79.0653731457051,-1.02949641157685,-20.8885720076918));
#30808=CARTESIAN_POINT('Ctrl Pts',(79.1842280094488,9.07070441569705,-18.8444852618751));
#30809=CARTESIAN_POINT('Ctrl Pts',(79.3030828731926,16.9686730893506,-12.2252377060213));
#30810=CARTESIAN_POINT('Ctrl Pts',(79.4219377369363,20.7469002557211,-2.63788422057037));
#30811=CARTESIAN_POINT('Ctrl Pts',(79.5407926006801,19.488088539859,7.58990832912952));
#30812=CARTESIAN_POINT('Ctrl Pts',(79.6596474644237,13.4978587082429,15.9749839960573));
#30813=CARTESIAN_POINT('Ctrl Pts',(79.7785023281676,4.23054949116273,20.4815710917107));
#30814=CARTESIAN_POINT('Ctrl Pts',(79.8973571919112,-6.06387423543652,20.0155372807922));
#30815=CARTESIAN_POINT('Ctrl Pts',(80.0162120556551,-14.8860794655671,14.6900286428174));
#30816=CARTESIAN_POINT('Ctrl Pts',(80.1350669193987,-20.0941659527598,5.79799948645444));
#30817=CARTESIAN_POINT('Ctrl Pts',(80.2539217831425,-20.4236877405258,-4.50169773079794));
#30818=CARTESIAN_POINT('Ctrl Pts',(80.3727766468861,-15.7946418386806,-13.7084496778365));
#30819=CARTESIAN_POINT('Ctrl Pts',(80.49163151063,-7.33089175974107,-19.586993883415));
#30820=CARTESIAN_POINT('Ctrl Pts',(80.6104863743736,2.91268983041759,-20.7101072265152));
#30821=CARTESIAN_POINT('Ctrl Pts',(80.7293412381174,12.4491136405291,-16.8051144877733));
#30822=CARTESIAN_POINT('Ctrl Pts',(80.8481961018612,18.9630777731095,-8.82008983814658));
#30823=CARTESIAN_POINT('Ctrl Pts',(80.9670509656049,20.8730885973582,1.30632147223087));
#30824=CARTESIAN_POINT('Ctrl Pts',(81.0859058293486,17.7154238864056,11.1155773537385));
#30825=CARTESIAN_POINT('Ctrl Pts',(81.2047606930925,10.2567176785937,18.2261363388843));
#30826=CARTESIAN_POINT('Ctrl Pts',(81.323615556836,0.307832932572739,20.9116604378418));
#30827=CARTESIAN_POINT('Ctrl Pts',(81.44247042058,-9.71578907209836,18.5201443322797));
#30828=CARTESIAN_POINT('Ctrl Pts',(81.5613252843235,-17.3805619607799,11.6322125715389));
#30829=CARTESIAN_POINT('Ctrl Pts',(81.6801801480674,-20.8255928488529,1.92015256575688));
#30830=CARTESIAN_POINT('Ctrl Pts',(81.799035011811,-19.214479463215,-8.25809193092852));
#30831=CARTESIAN_POINT('Ctrl Pts',(81.9178898755548,-12.9383761771515,-16.4313945020042));
#30832=CARTESIAN_POINT('Ctrl Pts',(82.0367447392985,-3.52102754484433,-20.6153988176417));
#30833=CARTESIAN_POINT('Ctrl Pts',(82.1555996030423,6.75117421878302,-19.7942908448273));
#30834=CARTESIAN_POINT('Ctrl Pts',(82.274454466786,15.3842912699189,-14.1674233897442));
#30835=CARTESIAN_POINT('Ctrl Pts',(82.3933093305298,20.2823311602726,-5.10091620074396));
#30836=CARTESIAN_POINT('Ctrl Pts',(82.5121641942734,20.2561226367727,5.20401759278348));
#30837=CARTESIAN_POINT('Ctrl Pts',(82.6310190580173,15.3120287392127,14.2454932968817));
#30838=CARTESIAN_POINT('Ctrl Pts',(82.7498739217609,6.65040194880476,19.8283750544846));
#30839=CARTESIAN_POINT('Ctrl Pts',(82.8687287855047,-3.62584354539574,20.5972221905355));
#30840=CARTESIAN_POINT('Ctrl Pts',(82.9875836492484,-13.0217881419229,16.3653700529151));
#30841=CARTESIAN_POINT('Ctrl Pts',(83.1064385129922,-19.2562362074694,8.16024941433271));
#30842=CARTESIAN_POINT('Ctrl Pts',(83.2252933767359,-20.8155564559951,-2.02605844171725));
#30843=CARTESIAN_POINT('Ctrl Pts',(83.3441482404796,-17.3211691177578,-11.7204694349677));
#30844=CARTESIAN_POINT('Ctrl Pts',(83.4630031042234,-9.62145947804478,-18.5693247290879));
#30845=CARTESIAN_POINT('Ctrl Pts',(83.581857967967,0.41419745487271,-20.9098240989816));
#30846=CARTESIAN_POINT('Ctrl Pts',(83.7007128317109,10.3492934047325,-18.1737291001251));
#30847=CARTESIAN_POINT('Ctrl Pts',(83.8195676954545,17.7717348066487,-11.025322913372));
#30848=CARTESIAN_POINT('Ctrl Pts',(83.9384225591984,20.8794632575961,-1.20013226632287));
#30849=CARTESIAN_POINT('Ctrl Pts',(84.057277422942,18.9179685006256,8.91643264940149));
#30850=CARTESIAN_POINT('Ctrl Pts',(84.1761322866858,12.3634722959219,16.8682203023895));
#30851=CARTESIAN_POINT('Ctrl Pts',(84.2949871504295,2.80730885869799,20.7246548910676));
#30852=CARTESIAN_POINT('Ctrl Pts',(84.4138420141732,-7.43042742562143,19.5494514412693));
#30853=CARTESIAN_POINT('Ctrl Pts',(84.532696877917,-15.8641664191098,13.6279318757016));
#30854=CARTESIAN_POINT('Ctrl Pts',(84.6515517416607,-20.4463217011843,4.39775309375782));
#30855=CARTESIAN_POINT('Ctrl Pts',(84.7704066054045,-20.0644141045594,-5.90013474615043));
#30856=CARTESIAN_POINT('Ctrl Pts',(84.8892614691482,-14.8111651148504,-14.7655576028342));
#30857=CARTESIAN_POINT('Ctrl Pts',(85.0081163328919,-5.96198547260468,-20.0461226327294));
#30858=CARTESIAN_POINT('Ctrl Pts',(85.1269711966356,4.33467558954779,-20.4597871669124));
#30859=CARTESIAN_POINT('Ctrl Pts',(85.2458260603795,13.5789418738155,-15.9061196075446));
#30860=CARTESIAN_POINT('Ctrl Pts',(85.364680924123,19.5264429856993,-7.49068272644153));
#30861=CARTESIAN_POINT('Ctrl Pts',(85.483535787867,20.7332140926975,2.74338053655433));
#30862=CARTESIAN_POINT('Ctrl Pts',(85.6023906516105,16.9062691143363,12.3113917984773));
#30863=CARTESIAN_POINT('Ctrl Pts',(85.7212455153543,8.97473338589818,18.890380198239));
#30864=CARTESIAN_POINT('Ctrl Pts',(85.8401003790982,-1.13573415718418,20.8830651798576));
#30865=CARTESIAN_POINT('Ctrl Pts',(85.9589552428418,-10.9704623349105,17.8056524603926));
#30866=CARTESIAN_POINT('Ctrl Pts',(86.0778101065857,-18.1417253850317,10.4052920879747));
#30867=CARTESIAN_POINT('Ctrl Pts',(86.1966649703292,-20.908447273396,0.478681520004721));
#30868=CARTESIAN_POINT('Ctrl Pts',(86.3155198340731,-18.5989090657894,-9.56414580317936));
#30869=CARTESIAN_POINT('Ctrl Pts',(86.4343746978168,-11.7738322969147,-17.28494074118));
#30870=CARTESIAN_POINT('Ctrl Pts',(86.5532295615605,-2.09024411951815,-20.8092090888336));
#30871=CARTESIAN_POINT('Ctrl Pts',(86.6720844253043,8.10082424882741,-19.2813108960876));
#30872=CARTESIAN_POINT('Ctrl Pts',(86.7909392890479,16.3251329462566,-13.0721971247768));
#30873=CARTESIAN_POINT('Ctrl Pts',(86.9097941527918,20.5859421139072,-3.68934827101431));
#30874=CARTESIAN_POINT('Ctrl Pts',(87.0286490165353,19.8487906427609,6.58921948350647));
#30875=CARTESIAN_POINT('Ctrl Pts',(87.1475038802793,14.2926479488024,15.2680227270453));
#30876=CARTESIAN_POINT('Ctrl Pts',(87.2663587440228,5.26646286003707,20.2399770831349));
#30877=CARTESIAN_POINT('Ctrl Pts',(87.3852136077667,-5.03834110050527,20.2979659655083));
#30878=CARTESIAN_POINT('Ctrl Pts',(87.5040684715104,-14.1199107603864,15.4279105358017));
#30879=CARTESIAN_POINT('Ctrl Pts',(87.6229233352541,-19.7733760462607,6.81218783616099));
#30880=CARTESIAN_POINT('Ctrl Pts',(87.7417781989979,-20.6261596519617,-3.45743277501727));
#30881=CARTESIAN_POINT('Ctrl Pts',(87.8606330627416,-16.4712183986482,-12.887640119355));
#30882=CARTESIAN_POINT('Ctrl Pts',(87.9794879264853,-8.3173102399601,-19.1889200778529));
#30883=CARTESIAN_POINT('Ctrl Pts',(88.0983427902292,1.85591716921299,-20.8314155746315));
#30884=CARTESIAN_POINT('Ctrl Pts',(88.2171976539728,11.5785554866035,-17.4163531264618));
#30885=CARTESIAN_POINT('Ctrl Pts',(88.3360525177166,18.4900927013111,-9.77285911485978));
#30886=CARTESIAN_POINT('Ctrl Pts',(88.4549073814602,20.9125103499811,0.243339770501251));
#30887=CARTESIAN_POINT('Ctrl Pts',(88.5737622452041,18.2576814481021,10.2004593779692));
#30888=CARTESIAN_POINT('Ctrl Pts',(88.6926171089477,11.170158976582,17.6810591260786));
#30889=CARTESIAN_POINT('Ctrl Pts',(88.8114719726915,1.37068800228615,20.868960630139));
#30890=CARTESIAN_POINT('Ctrl Pts',(88.9303268364353,-8.76156563726881,18.9901888080648));
#30891=CARTESIAN_POINT('Ctrl Pts',(89.049181700179,-16.766641421806,12.5008815214899));
#30892=CARTESIAN_POINT('Ctrl Pts',(89.1680365639226,-20.7010259838003,2.97654608568703));
#30893=CARTESIAN_POINT('Ctrl Pts',(89.2868914276665,-19.6095092546341,-7.27045047947625));
#30894=CARTESIAN_POINT('Ctrl Pts',(89.4057462914101,-13.7570952656821,-15.7522897774154));
#30895=CARTESIAN_POINT('Ctrl Pts',(89.524601155154,-4.56466310983042,-20.4097073491906));
#30896=CARTESIAN_POINT('Ctrl Pts',(89.6434560188976,5.73600137388006,-20.1119514620605));
#30897=CARTESIAN_POINT('Ctrl Pts',(89.7623108826413,14.6440500167558,-14.9313128191482));
#30898=CARTESIAN_POINT('Ctrl Pts',(89.8811657463853,19.996741067543,-6.12557344600731));
#30899=CARTESIAN_POINT('Ctrl Pts',(90.0000206101288,20.4945207331834,4.16736407124383));
#30900=CARTESIAN_POINT('Ctrl Pts',(90.1188754738726,16.0165355102348,13.4485275657482));
#30901=CARTESIAN_POINT('Ctrl Pts',(90.2377303376165,7.64997362942123,19.4645885301395));
#30902=CARTESIAN_POINT('Ctrl Pts',(90.3565852013599,-2.57388810220134,20.7549368562865));
#30903=CARTESIAN_POINT('Ctrl Pts',(90.475440065104,-12.172848063172,17.0062950847534));
#30904=CARTESIAN_POINT('Ctrl Pts',(90.5942949288474,-18.8164215450704,9.12877783988716));
#30905=CARTESIAN_POINT('Ctrl Pts',(90.7131497925914,-20.8916476223885,-0.965071109213948));
#30906=CARTESIAN_POINT('Ctrl Pts',(90.8320046563349,-17.8946924029286,-10.8246147761969));
#30907=CARTESIAN_POINT('Ctrl Pts',(90.9508595200788,-10.5531717722109,-18.05610365574));
#30908=CARTESIAN_POINT('Ctrl Pts',(91.0697143838226,-0.649498319719339,
-20.9038376377461));
#30909=CARTESIAN_POINT('Ctrl Pts',(91.1885692475662,9.41186437891623,-18.6764334630907));
#30910=CARTESIAN_POINT('Ctrl Pts',(91.30742411131,17.1881649583186,-11.9146634752632));
#30911=CARTESIAN_POINT('Ctrl Pts',(91.4262789750537,20.7914374193968,-2.26020113694711));
#30912=CARTESIAN_POINT('Ctrl Pts',(91.5451338387974,19.3468526295679,7.94302560746775));
#30913=CARTESIAN_POINT('Ctrl Pts',(91.6639887025412,13.2051503325794,16.2177622139406));
#30914=CARTESIAN_POINT('Ctrl Pts',(91.7828435662849,3.85741299640702,20.5551491420764));
#30915=CARTESIAN_POINT('Ctrl Pts',(91.9016984300287,-6.42680578368705,19.901890639009));
#30916=CARTESIAN_POINT('Ctrl Pts',(92.0205532937724,-15.1507724219245,14.417065314141));
#30917=CARTESIAN_POINT('Ctrl Pts',(92.1394081575162,-20.1961980925971,5.43136836909382));
#30918=CARTESIAN_POINT('Ctrl Pts',(92.2582630212598,-20.3385992009415,-4.87175126335728));
#30919=CARTESIAN_POINT('Ctrl Pts',(92.3771178850036,-15.5424768337762,-13.9946067183758));
#30920=CARTESIAN_POINT('Ctrl Pts',(92.4563544608328,-9.83019890208951,-17.8072577621103));
#30921=CARTESIAN_POINT('Ctrl Pts',(92.4959727487473,-6.69077064826668,-18.9176091918295));
#30922=CARTESIAN_POINT('',(92.,-6.97721143603873,-19.7274971949513));
#30923=CARTESIAN_POINT('Ctrl Pts',(92.,-13.2939520371397,15.0312716283101));
#30924=CARTESIAN_POINT('Ctrl Pts',(92.,-13.6160698917503,14.758567432308));
#30925=CARTESIAN_POINT('Ctrl Pts',(92.,-13.9291994758583,14.475971697715));
#30926=CARTESIAN_POINT('Ctrl Pts',(92.,-14.2328195904016,14.183841939621));
#30927=CARTESIAN_POINT('Ctrl Pts',(92.,-14.3443295390009,14.0765520311168));
#30928=CARTESIAN_POINT('Ctrl Pts',(92.,-14.4545565403831,13.9679756804271));
#30929=CARTESIAN_POINT('Ctrl Pts',(92.,-14.5634738142937,13.8581291163106));
#30930=CARTESIAN_POINT('Ctrl Pts',(92.,-14.858732771742,13.5603509876831));
#30931=CARTESIAN_POINT('Ctrl Pts',(92.,-15.1443694959895,13.2532412422133));
#30932=CARTESIAN_POINT('Ctrl Pts',(92.,-15.4201237116956,12.9373782285482));
#30933=CARTESIAN_POINT('Ctrl Pts',(92.,-15.697033728144,12.6201913014671));
#30934=CARTESIAN_POINT('Ctrl Pts',(92.,-15.9639785353498,12.294177135262));
#30935=CARTESIAN_POINT('Ctrl Pts',(92.,-16.2206559670913,11.9598852286998));
#30936=CARTESIAN_POINT('Ctrl Pts',(92.,-16.4160308888044,11.7054325694582));
#30937=CARTESIAN_POINT('Ctrl Pts',(92.,-16.6054563648391,11.4461831784212));
#30938=CARTESIAN_POINT('Ctrl Pts',(92.,-16.788782522303,11.1823678395403));
#30939=CARTESIAN_POINT('Ctrl Pts',(92.,-16.8144368585662,11.1454499904528));
#30940=CARTESIAN_POINT('Ctrl Pts',(92.,-16.8399694108848,11.108446018421));
#30941=CARTESIAN_POINT('Ctrl Pts',(92.,-16.8653752109956,11.071363398425));
#30942=CARTESIAN_POINT('Ctrl Pts',(92.,-17.1037405056281,10.723442466885));
#30943=CARTESIAN_POINT('Ctrl Pts',(92.,-17.3310748449526,10.3684236388796));
#30944=CARTESIAN_POINT('Ctrl Pts',(92.,-17.5471276373729,10.0068939956817));
#30945=CARTESIAN_POINT('Ctrl Pts',(92.,-17.7684746335703,9.63650535287952));
#30946=CARTESIAN_POINT('Ctrl Pts',(92.,-17.9779808926936,9.2592825348923));
#30947=CARTESIAN_POINT('Ctrl Pts',(92.,-18.1753337935665,8.87582095352862));
#30948=CARTESIAN_POINT('Ctrl Pts',(92.,-18.3685180548043,8.50045914237103));
#30949=CARTESIAN_POINT('Ctrl Pts',(92.,-18.5500570976423,8.11911876362687));
#30950=CARTESIAN_POINT('Ctrl Pts',(92.,-18.7196128001755,7.7323317844173));
#30951=CARTESIAN_POINT('Ctrl Pts',(92.,-18.8946566564853,7.33302534175734));
#30952=CARTESIAN_POINT('Ctrl Pts',(92.,-19.0569294873076,6.92791358991489));
#30953=CARTESIAN_POINT('Ctrl Pts',(92.,-19.2060045971,6.51756051797982));
#30954=CARTESIAN_POINT('Ctrl Pts',(92.,-19.2198478928059,6.47945463345951));
#30955=CARTESIAN_POINT('Ctrl Pts',(92.,-19.2335758890648,6.4413074867314));
#30956=CARTESIAN_POINT('Ctrl Pts',(92.,-19.2471856417164,6.40312712225039));
#30957=CARTESIAN_POINT('Ctrl Pts',(92.,-19.3801360300814,6.03015235807848));
#30958=CARTESIAN_POINT('Ctrl Pts',(92.,-19.5018839462995,5.65379323102824));
#30959=CARTESIAN_POINT('Ctrl Pts',(92.,-19.612223314782,5.27451367654917));
#30960=CARTESIAN_POINT('Ctrl Pts',(92.,-19.7305593453794,4.86774646751861));
#30961=CARTESIAN_POINT('Ctrl Pts',(92.,-19.8357743611108,4.45762013617097));
#30962=CARTESIAN_POINT('Ctrl Pts',(92.,-19.92796760317,4.0447862442832));
#30963=CARTESIAN_POINT('Ctrl Pts',(92.,-20.0201788060094,3.63187192547301));
#30964=CARTESIAN_POINT('Ctrl Pts',(92.,-20.0993631833585,3.21624845084337));
#30965=CARTESIAN_POINT('Ctrl Pts',(92.,-20.1655698219861,2.79854789811281));
#30966=CARTESIAN_POINT('Ctrl Pts',(92.,-20.2320538863996,2.37909705407441));
#30967=CARTESIAN_POINT('Ctrl Pts',(92.,-20.2854512878204,1.95755114980799));
#30968=CARTESIAN_POINT('Ctrl Pts',(92.,-20.325760397772,1.53453830704263));
#30969=CARTESIAN_POINT('Ctrl Pts',(92.,-20.3660288602495,1.11195202798934));
#30970=CARTESIAN_POINT('Ctrl Pts',(92.,-20.3932354432298,0.687901217036152));
#30971=CARTESIAN_POINT('Ctrl Pts',(92.,-20.4073267612968,0.263008398905277));
#30972=CARTESIAN_POINT('Ctrl Pts',(92.,-20.421342781554,-0.159613978774176));
#30973=CARTESIAN_POINT('Ctrl Pts',(92.,-20.4223833262527,-0.583069928986948));
#30974=CARTESIAN_POINT('Ctrl Pts',(92.,-20.4103444698736,-1.00674237530884));
#30975=CARTESIAN_POINT('Ctrl Pts',(92.,-20.408349887765,-1.076935876648));
#30976=CARTESIAN_POINT('Ctrl Pts',(92.,-20.4059961685756,-1.14713530012027));
#30977=CARTESIAN_POINT('Ctrl Pts',(92.,-20.4032827023909,-1.21733781136343));
#30978=CARTESIAN_POINT('Ctrl Pts',(92.,-20.4013287910156,-1.26788920060626));
#30979=CARTESIAN_POINT('Ctrl Pts',(92.,-20.3991881262455,-1.31844611013296));
#30980=CARTESIAN_POINT('Ctrl Pts',(92.,-20.3968618361394,-1.36898023731617));
#30981=CARTESIAN_POINT('Ctrl Pts',(92.,-20.377197273692,-1.79615460269462));
#30982=CARTESIAN_POINT('Ctrl Pts',(92.,-20.3442608580358,-2.22206346610525));
#30983=CARTESIAN_POINT('Ctrl Pts',(92.,-20.2981227972436,-2.64607409640738));
#30984=CARTESIAN_POINT('Ctrl Pts',(92.,-20.2518214654591,-3.07158519368148));
#30985=CARTESIAN_POINT('Ctrl Pts',(92.,-20.1922249321044,-3.4951851506192));
#30986=CARTESIAN_POINT('Ctrl Pts',(92.,-20.1193523275807,-3.91624204251575));
#30987=CARTESIAN_POINT('Ctrl Pts',(92.,-20.069345617195,-4.20518011720942));
#30988=CARTESIAN_POINT('Ctrl Pts',(92.,-20.013086138115,-4.4929208214171));
#30989=CARTESIAN_POINT('Ctrl Pts',(92.,-19.9505658664369,-4.77925995369804));
#30990=CARTESIAN_POINT('Ctrl Pts',(92.,-19.8594604469175,-5.19651736591093));
#30991=CARTESIAN_POINT('Ctrl Pts',(92.,-19.7550627546659,-5.61079923843387));
#30992=CARTESIAN_POINT('Ctrl Pts',(92.,-19.6377077496538,-6.02155968710754));
#30993=CARTESIAN_POINT('Ctrl Pts',(92.,-19.5203692827226,-6.43226224997153));
#30994=CARTESIAN_POINT('Ctrl Pts',(92.,-19.3900769227109,-6.83944488042613));
#30995=CARTESIAN_POINT('Ctrl Pts',(92.,-19.2471147713027,-7.24254753502617));
#30996=CARTESIAN_POINT('Ctrl Pts',(92.,-19.1398755268731,-7.54492423879746));
#30997=CARTESIAN_POINT('Ctrl Pts',(92.,-19.0255061208544,-7.84500495401166));
#30998=CARTESIAN_POINT('Ctrl Pts',(92.,-18.9041089056825,-8.14254540778852));
#30999=CARTESIAN_POINT('Ctrl Pts',(92.,-18.7978863424071,-8.40289330484327));
#31000=CARTESIAN_POINT('Ctrl Pts',(92.,-18.6862828670782,-8.6612962612323));
#31001=CARTESIAN_POINT('Ctrl Pts',(92.,-18.5693581238797,-8.91758517612054));
#31002=CARTESIAN_POINT('Ctrl Pts',(92.,-18.5532381230933,-8.95291882233212));
#31003=CARTESIAN_POINT('Ctrl Pts',(92.,-18.5370157670781,-8.9882148657338));
#31004=CARTESIAN_POINT('Ctrl Pts',(92.,-18.5206952618725,-9.02346409661682));
#31005=CARTESIAN_POINT('Ctrl Pts',(92.,-18.3411773006904,-9.41118923022199));
#31006=CARTESIAN_POINT('Ctrl Pts',(92.,-18.1499874366914,-9.79282687859415));
#31007=CARTESIAN_POINT('Ctrl Pts',(92.,-17.9475101887474,-10.1678622906306));
#31008=CARTESIAN_POINT('Ctrl Pts',(92.,-17.7429704910178,-10.5467178440062));
#31009=CARTESIAN_POINT('Ctrl Pts',(92.,-17.5269121246835,-10.9188364850125));
#31010=CARTESIAN_POINT('Ctrl Pts',(92.,-17.299679928222,-11.2836750922875));
#31011=CARTESIAN_POINT('Ctrl Pts',(92.,-17.0722860038054,-11.6487733661187));
#31012=CARTESIAN_POINT('Ctrl Pts',(92.,-16.8337020963105,-12.0065817412458));
#31013=CARTESIAN_POINT('Ctrl Pts',(92.,-16.58422560562,-12.3565359028326));
#31014=CARTESIAN_POINT('Ctrl Pts',(92.,-16.3362967632301,-12.7043190944734));
#31015=CARTESIAN_POINT('Ctrl Pts',(92.,-16.0776097838226,-13.044345683683));
#31016=CARTESIAN_POINT('Ctrl Pts',(92.,-15.8084129870003,-13.3760348394112));
#31017=CARTESIAN_POINT('Ctrl Pts',(92.,-15.6746083502117,-13.5409013888383));
#31018=CARTESIAN_POINT('Ctrl Pts',(92.,-15.5382065058082,-13.7037076289432));
#31019=CARTESIAN_POINT('Ctrl Pts',(92.,-15.3992342253977,-13.8643791870089));
#31020=CARTESIAN_POINT('Ctrl Pts',(92.,-15.1170023822946,-14.1906790061758));
#31021=CARTESIAN_POINT('Ctrl Pts',(92.,-14.8241712853989,-14.508177194315));
#31022=CARTESIAN_POINT('Ctrl Pts',(92.,-14.5212455312031,-14.8165114420203));
#31023=CARTESIAN_POINT('Ctrl Pts',(92.,-14.3887155137425,-14.9514076753914));
#31024=CARTESIAN_POINT('Ctrl Pts',(92.,-14.2542528654501,-15.084549356486));
#31025=CARTESIAN_POINT('Ctrl Pts',(92.,-14.1178978857168,-15.2159036206765));
#31026=CARTESIAN_POINT('Ctrl Pts',(92.,-14.0488781796834,-15.2823920812989));
#31027=CARTESIAN_POINT('Ctrl Pts',(92.,-13.9793736127407,-15.3484225538464));
#31028=CARTESIAN_POINT('Ctrl Pts',(92.,-13.9093893078444,-15.4139906160304));
#31029=CARTESIAN_POINT('Ctrl Pts',(92.,-13.8830137967218,-15.438701744561));
#31030=CARTESIAN_POINT('Ctrl Pts',(92.,-13.8565693542944,-15.4633479251348));
#31031=CARTESIAN_POINT('Ctrl Pts',(92.,-13.8300587085628,-15.4879266405824));
#31032=CARTESIAN_POINT('Ctrl Pts',(92.,-13.5167319996439,-15.7784200558922));
#31033=CARTESIAN_POINT('Ctrl Pts',(92.,-13.1948692359732,-16.058836627676));
#31034=CARTESIAN_POINT('Ctrl Pts',(92.,-12.8650638961591,-16.3289305947836));
#31035=CARTESIAN_POINT('Ctrl Pts',(92.,-12.5319527241127,-16.6017318720359));
#31036=CARTESIAN_POINT('Ctrl Pts',(92.,-12.1907385840942,-16.8640029162961));
#31037=CARTESIAN_POINT('Ctrl Pts',(92.,-11.8419899279349,-17.115458924327));
#31038=CARTESIAN_POINT('Ctrl Pts',(92.,-11.4912672606211,-17.3683382409669));
#31039=CARTESIAN_POINT('Ctrl Pts',(92.,-11.1329241297363,-17.6102800876755));
#31040=CARTESIAN_POINT('Ctrl Pts',(92.,-10.76750130731,-17.8409578158456));
#31041=CARTESIAN_POINT('Ctrl Pts',(92.,-10.4024136912143,-18.0714239408261));
#31042=CARTESIAN_POINT('Ctrl Pts',(92.,-10.0302589179817,-18.2906469148638));
#31043=CARTESIAN_POINT('Ctrl Pts',(92.,-9.65154557559993,-18.4982593079888));
#31044=CARTESIAN_POINT('Ctrl Pts',(92.,-9.27493495961211,-18.7047189768501));
#31045=CARTESIAN_POINT('Ctrl Pts',(92.,-8.8918379483303,-18.8996969149001));
#31046=CARTESIAN_POINT('Ctrl Pts',(92.,-8.50273110093215,-19.0827861959131));
#31047=CARTESIAN_POINT('Ctrl Pts',(92.,-8.11885407809306,-19.2634146494574));
#31048=CARTESIAN_POINT('Ctrl Pts',(92.,-7.72912723839731,-19.432472082855));
#31049=CARTESIAN_POINT('Ctrl Pts',(92.,-7.33399185124482,-19.5895198058331));
#31050=CARTESIAN_POINT('Ctrl Pts',(92.,-7.21554722023826,-19.6365959731504));
#31051=CARTESIAN_POINT('Ctrl Pts',(92.,-7.09661652008284,-19.6825926742559));
#31052=CARTESIAN_POINT('Ctrl Pts',(92.,-6.97721143603873,-19.7274971949513));
#31053=CARTESIAN_POINT('Ctrl Pts',(92.,-6.97721143603902,-19.7274971949512));
#31054=CARTESIAN_POINT('Ctrl Pts',(91.9603817120854,-10.2510427877189,-18.5696101441574));
#31055=CARTESIAN_POINT('Ctrl Pts',(91.9207634241708,-13.229456860328,-16.5816722919714));
#31056=CARTESIAN_POINT('Ctrl Pts',(91.8811451362562,-15.5522390204362,-14.0021338613507));
#31057=CARTESIAN_POINT('Ctrl Pts',(91.8415268483417,-17.8750211805444,-11.4225954307301));
#31058=CARTESIAN_POINT('Ctrl Pts',(91.8019085604271,-19.5421714281517,-8.25145642167493));
#31059=CARTESIAN_POINT('Ctrl Pts',(91.7622902725125,-20.350996970433,-4.87518526992051));
#31060=CARTESIAN_POINT('Ctrl Pts',(91.7435791307256,-20.7329935230127,-3.28062145717681));
#31061=CARTESIAN_POINT('Ctrl Pts',(91.7248679889387,-20.923537688795,-1.64030218838607));
#31062=CARTESIAN_POINT('Ctrl Pts',(91.7061568471519,-20.9232794228044,4.20060754047213E-5));
#31063=CARTESIAN_POINT('Origin',(101.6,4.3,25.25));
#31064=CARTESIAN_POINT('',(101.,4.3,34.));
#31065=CARTESIAN_POINT('',(101.6,4.9,36.8354893757516));
#31066=CARTESIAN_POINT('Ctrl Pts',(101.,4.3,34.));
#31067=CARTESIAN_POINT('Ctrl Pts',(101.,4.44326450824761,34.4893414541742));
#31068=CARTESIAN_POINT('Ctrl Pts',(101.064916666253,4.61344480367674,35.0734607689975));
#31069=CARTESIAN_POINT('Ctrl Pts',(101.268537390365,4.81706552778855,35.9649713605754));
#31070=CARTESIAN_POINT('Ctrl Pts',(101.427042536443,4.9,36.4451060520726));
#31071=CARTESIAN_POINT('Ctrl Pts',(101.6,4.9,36.8354893757516));
#31072=CARTESIAN_POINT('',(101.6,4.9,25.5340948537441));
#31073=CARTESIAN_POINT('',(101.6,4.9,25.25));
#31074=CARTESIAN_POINT('',(101.,4.3,25.6419578035687));
#31075=CARTESIAN_POINT('Ctrl Pts',(101.,4.3,25.6419578035687));
#31076=CARTESIAN_POINT('Ctrl Pts',(101.,4.37551113136118,25.6292950471856));
#31077=CARTESIAN_POINT('Ctrl Pts',(101.015114297469,4.45605670300991,25.6154099532735));
#31078=CARTESIAN_POINT('Ctrl Pts',(101.076714673797,4.60433114552009,25.5891735528367));
#31079=CARTESIAN_POINT('Ctrl Pts',(101.123204104127,4.67206195455091,25.5768410722651));
#31080=CARTESIAN_POINT('Ctrl Pts',(101.230018577124,4.7782143249361,25.5572207559602));
#31081=CARTESIAN_POINT('Ctrl Pts',(101.297146680589,4.82405550675615,25.5485703918952));
#31082=CARTESIAN_POINT('Ctrl Pts',(101.44448562384,4.88495263372662,25.5369966591618));
#31083=CARTESIAN_POINT('Ctrl Pts',(101.524701702258,4.9,25.5340948537441));
#31084=CARTESIAN_POINT('Ctrl Pts',(101.6,4.9,25.5340948537441));
#31085=CARTESIAN_POINT('',(101.,4.3,25.25));
#31086=CARTESIAN_POINT('Origin',(108.,-4.9,34.));
#31087=CARTESIAN_POINT('',(101.,-4.3,34.));
#31088=CARTESIAN_POINT('',(101.,-4.9,34.));
#31089=CARTESIAN_POINT('',(101.6,-4.9,36.8354893757516));
#31090=CARTESIAN_POINT('Ctrl Pts',(101.6,-4.9,36.8354893757516));
#31091=CARTESIAN_POINT('Ctrl Pts',(101.427042536443,-4.9,36.4451060520726));
#31092=CARTESIAN_POINT('Ctrl Pts',(101.268537390365,-4.81706552778855,35.9649713605754));
#31093=CARTESIAN_POINT('Ctrl Pts',(101.064916666253,-4.61344480367674,35.0734607689975));
#31094=CARTESIAN_POINT('Ctrl Pts',(101.,-4.44326450824761,34.4893414541742));
#31095=CARTESIAN_POINT('Ctrl Pts',(101.,-4.3,34.));
#31096=CARTESIAN_POINT('',(114.402897902826,-4.9,36.8289394560486));
#31097=CARTESIAN_POINT('Origin',(108.,-4.9,34.));
#31098=CARTESIAN_POINT('',(115.,-4.35889894354063,34.));
#31099=CARTESIAN_POINT('Ctrl Pts',(115.,-4.35889894354085,34.));
#31100=CARTESIAN_POINT('Ctrl Pts',(115.,-4.35889894354085,34.1229692605315));
#31101=CARTESIAN_POINT('Ctrl Pts',(114.996901424204,-4.39006230423687,34.2401264537803));
#31102=CARTESIAN_POINT('Ctrl Pts',(114.984616986144,-4.45009707127197,34.4790000665593));
#31103=CARTESIAN_POINT('Ctrl Pts',(114.975348582715,-4.48313072407473,34.5996468313749));
#31104=CARTESIAN_POINT('Ctrl Pts',(114.937384384277,-4.58154753518053,34.9658966690121));
#31105=CARTESIAN_POINT('Ctrl Pts',(114.898348782177,-4.64734858287202,35.2151996628246));
#31106=CARTESIAN_POINT('Ctrl Pts',(114.745032017671,-4.81487871806176,35.9328510722238));
#31107=CARTESIAN_POINT('Ctrl Pts',(114.592738308154,-4.90000000000001,36.3992629811611));
#31108=CARTESIAN_POINT('Ctrl Pts',(114.402897902826,-4.90000000000001,36.8289394560486));
#31109=CARTESIAN_POINT('Ctrl Pts',(115.,-4.35889894354063,34.));
#31110=CARTESIAN_POINT('Ctrl Pts',(115.,-4.35889894354063,34.4224068534569));
#31111=CARTESIAN_POINT('Ctrl Pts',(114.958162834155,-4.27540728759944,34.8694586605386));
#31112=CARTESIAN_POINT('Ctrl Pts',(114.806829998337,-3.93948854882627,35.6849438766281));
#31113=CARTESIAN_POINT('Ctrl Pts',(114.699216397495,-3.68627980790566,36.0534032907636));
#31114=CARTESIAN_POINT('Ctrl Pts',(114.552214908899,-3.27956064047775,36.4668024429472));
#31115=CARTESIAN_POINT('Ctrl Pts',(114.504985020473,-3.14149575848544,36.5883975490726));
#31116=CARTESIAN_POINT('Ctrl Pts',(114.458327956987,-2.99274032010601,36.6999999999994));
#31117=CARTESIAN_POINT('',(115.,4.35889894354063,34.));
#31118=CARTESIAN_POINT('Ctrl Pts',(114.458327956987,2.99274032010601,36.6999999999995));
#31119=CARTESIAN_POINT('Ctrl Pts',(114.504985020473,3.14149575848544,36.5883975490726));
#31120=CARTESIAN_POINT('Ctrl Pts',(114.552214908899,3.27956064047774,36.4668024429472));
#31121=CARTESIAN_POINT('Ctrl Pts',(114.699216397495,3.68627980790566,36.0534032907636));
#31122=CARTESIAN_POINT('Ctrl Pts',(114.806829998337,3.93948854882627,35.6849438766281));
#31123=CARTESIAN_POINT('Ctrl Pts',(114.958162834155,4.27540728759944,34.8694586605386));
#31124=CARTESIAN_POINT('Ctrl Pts',(115.,4.35889894354063,34.4224068534569));
#31125=CARTESIAN_POINT('Ctrl Pts',(115.,4.35889894354063,34.));
#31126=CARTESIAN_POINT('',(114.402897902826,4.9,36.8289394560486));
#31127=CARTESIAN_POINT('Ctrl Pts',(114.402897902826,4.90000000000001,36.8289394560486));
#31128=CARTESIAN_POINT('Ctrl Pts',(114.592738308154,4.90000000000001,36.3992629811611));
#31129=CARTESIAN_POINT('Ctrl Pts',(114.745032017671,4.81487871806176,35.9328510722238));
#31130=CARTESIAN_POINT('Ctrl Pts',(114.898348782177,4.64734858287202,35.2151996628246));
#31131=CARTESIAN_POINT('Ctrl Pts',(114.937384384277,4.58154753518053,34.9658966690121));
#31132=CARTESIAN_POINT('Ctrl Pts',(114.975348582715,4.48313072407473,34.5996468313749));
#31133=CARTESIAN_POINT('Ctrl Pts',(114.984616986144,4.45009707127197,34.4790000665593));
#31134=CARTESIAN_POINT('Ctrl Pts',(114.996901424204,4.39006230423687,34.2401264537803));
#31135=CARTESIAN_POINT('Ctrl Pts',(115.,4.35889894354085,34.1229692605315));
#31136=CARTESIAN_POINT('Ctrl Pts',(115.,4.35889894354085,34.));
#31137=CARTESIAN_POINT('Origin',(108.,4.9,34.));
#31138=CARTESIAN_POINT('Origin',(101.,-4.9,20.));
#31139=CARTESIAN_POINT('',(101.,-4.3,25.6419578035687));
#31140=CARTESIAN_POINT('Origin',(101.,0.,0.));
#31141=CARTESIAN_POINT('',(101.,-4.3,25.25));
#31142=CARTESIAN_POINT('Origin',(101.6,-4.3,25.25));
#31143=CARTESIAN_POINT('',(101.6,-4.9,25.5340948537441));
#31144=CARTESIAN_POINT('Ctrl Pts',(101.6,-4.9,25.5340948537441));
#31145=CARTESIAN_POINT('Ctrl Pts',(101.524701702258,-4.9,25.5340948537441));
#31146=CARTESIAN_POINT('Ctrl Pts',(101.44448562384,-4.88495263372662,25.5369966591618));
#31147=CARTESIAN_POINT('Ctrl Pts',(101.297146680589,-4.82405550675615,25.5485703918952));
#31148=CARTESIAN_POINT('Ctrl Pts',(101.230018577124,-4.7782143249361,25.5572207559602));
#31149=CARTESIAN_POINT('Ctrl Pts',(101.123204104127,-4.67206195455091,25.5768410722651));
#31150=CARTESIAN_POINT('Ctrl Pts',(101.076714673797,-4.60433114552009,25.5891735528367));
#31151=CARTESIAN_POINT('Ctrl Pts',(101.015114297469,-4.4560567030099,25.6154099532735));
#31152=CARTESIAN_POINT('Ctrl Pts',(101.,-4.37551113136118,25.6292950471856));
#31153=CARTESIAN_POINT('Ctrl Pts',(101.,-4.3,25.6419578035687));
#31154=CARTESIAN_POINT('',(101.6,-4.9,25.25));
#31155=CARTESIAN_POINT('Origin',(114.402897902826,4.3,10.));
#31156=CARTESIAN_POINT('',(114.402897902826,4.9,25.5340948537441));
#31157=CARTESIAN_POINT('',(115.,4.35889894354067,25.6320112359526));
#31158=CARTESIAN_POINT('Ctrl Pts',(114.402897902826,4.9,25.5340948537441));
#31159=CARTESIAN_POINT('Ctrl Pts',(114.478511084744,4.90000000000001,25.5340948537441));
#31160=CARTESIAN_POINT('Ctrl Pts',(114.559040039281,4.88482760707762,25.5370208646519));
#31161=CARTESIAN_POINT('Ctrl Pts',(114.706854852562,4.82346334338894,25.5486824859048));
#31162=CARTESIAN_POINT('Ctrl Pts',(114.774145994538,4.77728004571152,25.5573962293562));
#31163=CARTESIAN_POINT('Ctrl Pts',(114.880625044276,4.67080099597391,25.5770712542939));
#31164=CARTESIAN_POINT('Ctrl Pts',(114.926771808833,4.60323529106133,25.5893699985255));
#31165=CARTESIAN_POINT('Ctrl Pts',(114.980036874495,4.47446184335992,25.6121513464705));
#31166=CARTESIAN_POINT('Ctrl Pts',(114.994355992236,4.4161164192633,25.6222810125931));
#31167=CARTESIAN_POINT('Ctrl Pts',(115.,4.35889894354067,25.6320112359526));
#31168=CARTESIAN_POINT('',(114.402897902826,4.9,10.));
#31169=CARTESIAN_POINT('',(115.,4.35889894354067,10.));
#31170=CARTESIAN_POINT('Origin',(114.402897902826,-4.3,10.));
#31171=CARTESIAN_POINT('',(114.402897902826,-4.9,25.5340948537441));
#31172=CARTESIAN_POINT('',(114.402897902826,-4.9,10.));
#31173=CARTESIAN_POINT('',(115.,-4.35889894354067,25.6320112359526));
#31174=CARTESIAN_POINT('Ctrl Pts',(115.,-4.35889894354067,25.6320112359526));
#31175=CARTESIAN_POINT('Ctrl Pts',(114.994326080485,-4.41641965677671,25.6222294449785));
#31176=CARTESIAN_POINT('Ctrl Pts',(114.979885641476,-4.47506740166339,25.6120461078662));
#31177=CARTESIAN_POINT('Ctrl Pts',(114.926183229029,-4.60433114552009,25.5891735528367));
#31178=CARTESIAN_POINT('Ctrl Pts',(114.879693798699,-4.67206195455091,25.5768410722651));
#31179=CARTESIAN_POINT('Ctrl Pts',(114.772879325702,-4.7782143249361,25.5572207559602));
#31180=CARTESIAN_POINT('Ctrl Pts',(114.705751222236,-4.82405550675616,25.5485703918952));
#31181=CARTESIAN_POINT('Ctrl Pts',(114.558412278986,-4.88495263372663,25.5369966591618));
#31182=CARTESIAN_POINT('Ctrl Pts',(114.478196200568,-4.9,25.5340948537441));
#31183=CARTESIAN_POINT('Ctrl Pts',(114.402897902826,-4.9,25.5340948537441));
#31184=CARTESIAN_POINT('',(115.,-4.35889894354067,10.));
#31185=CARTESIAN_POINT('Origin',(136.,-29.8,0.));
#31186=CARTESIAN_POINT('',(130.55,-30.,-6.67432505535307E-16));
#31187=CARTESIAN_POINT('Origin',(136.,-30.,0.));
#31188=CARTESIAN_POINT('',(130.95,-29.6,6.18446633569414E-16));
#31189=CARTESIAN_POINT('',(130.75,-29.8,-6.42939569552361E-16));
#31190=CARTESIAN_POINT('Origin',(136.,-29.6,0.));
#31191=CARTESIAN_POINT('Origin',(136.,-30.,0.));
#31192=CARTESIAN_POINT('',(123.8,-30.,1.49406909495977E-15));
#31193=CARTESIAN_POINT('Origin',(136.,-30.,0.));
#31194=CARTESIAN_POINT('Origin',(136.,-30.,0.));
#31195=CARTESIAN_POINT('',(130.95,-14.,6.18446633569414E-16));
#31196=CARTESIAN_POINT('',(130.95,-30.,6.18446633569414E-16));
#31197=CARTESIAN_POINT('Origin',(136.,-14.,0.));
#31198=CARTESIAN_POINT('Origin',(124.,0.,37.8));
#31199=CARTESIAN_POINT('',(119.99,4.91083366458088E-16,37.6));
#31200=CARTESIAN_POINT('',(119.79,-5.15576302441035E-16,37.8));
#31201=CARTESIAN_POINT('Origin',(124.,0.,37.6));
#31202=CARTESIAN_POINT('Origin',(124.,0.,38.));
#31203=CARTESIAN_POINT('',(119.99,-4.91083366458088E-16,14.));
#31204=CARTESIAN_POINT('',(119.99,4.91083366458088E-16,38.));
#31205=CARTESIAN_POINT('Origin',(124.,0.,14.));
#31206=CARTESIAN_POINT('Origin',(136.,-29.6,0.));
#31207=CARTESIAN_POINT('',(123.,-29.2,-1.59204083889156E-15));
#31208=CARTESIAN_POINT('',(123.4,-29.6,-1.54305496692567E-15));
#31209=CARTESIAN_POINT('Origin',(136.,-29.2,0.));
#31210=CARTESIAN_POINT('Origin',(136.,-10.,0.));
#31211=CARTESIAN_POINT('',(123.,-26.,1.75424727101232E-16));
#31212=CARTESIAN_POINT('',(123.,-10.,-1.59204083889156E-15));
#31213=CARTESIAN_POINT('Ctrl Pts',(149.,-26.,2.22044604925031E-15));
#31214=CARTESIAN_POINT('Ctrl Pts',(149.,-26.,-0.831709457206476));
#31215=CARTESIAN_POINT('Ctrl Pts',(148.918892814918,-25.9591289790221,-1.68724313385081));
#31216=CARTESIAN_POINT('Ctrl Pts',(148.582552741345,-25.7933948769122,-3.37993305619291));
#31217=CARTESIAN_POINT('Ctrl Pts',(148.327434591979,-25.6686324247972,-4.21712194988806));
#31218=CARTESIAN_POINT('Ctrl Pts',(147.32514603902,-25.1974429335132,-6.61362985548687));
#31219=CARTESIAN_POINT('Ctrl Pts',(146.328719603369,-24.7502659309165,-8.05605670748142));
#31220=CARTESIAN_POINT('Ctrl Pts',(144.052950545147,-23.8901060781349,-10.3318257657034));
#31221=CARTESIAN_POINT('Ctrl Pts',(142.611570673602,-23.4155481619888,-11.325973226571));
#31222=CARTESIAN_POINT('Ctrl Pts',(140.218494030717,-22.8951850410383,-12.3268777552912));
#31223=CARTESIAN_POINT('Ctrl Pts',(139.382475328567,-22.7537733940447,-12.5818558368984));
#31224=CARTESIAN_POINT('Ctrl Pts',(137.690251278654,-22.5643527281993,-12.9184862150897));
#31225=CARTESIAN_POINT('Ctrl Pts',(136.833982935243,-22.5166604983954,-13.));
#31226=CARTESIAN_POINT('Ctrl Pts',(136.,-22.5166604983954,-13.));
#31227=CARTESIAN_POINT('Ctrl Pts',(135.166017064757,-22.5166604983954,-13.));
#31228=CARTESIAN_POINT('Ctrl Pts',(134.309748721346,-22.5643527281993,-12.9184862150897));
#31229=CARTESIAN_POINT('Ctrl Pts',(132.617524671433,-22.7537733940447,-12.5818558368984));
#31230=CARTESIAN_POINT('Ctrl Pts',(131.781505969283,-22.8951850410383,-12.3268777552912));
#31231=CARTESIAN_POINT('Ctrl Pts',(129.388429326398,-23.4155481619888,-11.325973226571));
#31232=CARTESIAN_POINT('Ctrl Pts',(127.947049454853,-23.8901060781349,-10.3318257657035));
#31233=CARTESIAN_POINT('Ctrl Pts',(125.671280396631,-24.7502659309165,-8.05605670748142));
#31234=CARTESIAN_POINT('Ctrl Pts',(124.67485396098,-25.1974429335132,-6.61362985548688));
#31235=CARTESIAN_POINT('Ctrl Pts',(123.672565408021,-25.6686324247972,-4.21712194988807));
#31236=CARTESIAN_POINT('Ctrl Pts',(123.417447258655,-25.7933948769122,-3.37993305619291));
#31237=CARTESIAN_POINT('Ctrl Pts',(123.081107185082,-25.9591289790221,-1.68724313385082));
#31238=CARTESIAN_POINT('Ctrl Pts',(123.,-26.,-0.831709457206481));
#31239=CARTESIAN_POINT('Ctrl Pts',(123.,-26.,1.38777878078145E-15));
#31240=CARTESIAN_POINT('Ctrl Pts',(123.,-26.,1.94289029309402E-15));
#31241=CARTESIAN_POINT('Ctrl Pts',(123.,-26.,0.831709457206478));
#31242=CARTESIAN_POINT('Ctrl Pts',(123.081107185082,-25.9591289790221,1.68724313385081));
#31243=CARTESIAN_POINT('Ctrl Pts',(123.417447258655,-25.7933948769122,3.37993305619291));
#31244=CARTESIAN_POINT('Ctrl Pts',(123.672565408021,-25.6686324247972,4.21712194988806));
#31245=CARTESIAN_POINT('Ctrl Pts',(124.67485396098,-25.1974429335132,6.61362985548687));
#31246=CARTESIAN_POINT('Ctrl Pts',(125.671280396631,-24.7502659309165,8.05605670748142));
#31247=CARTESIAN_POINT('Ctrl Pts',(127.947049454853,-23.8901060781349,10.3318257657034));
#31248=CARTESIAN_POINT('Ctrl Pts',(129.388429326398,-23.4155481619888,11.325973226571));
#31249=CARTESIAN_POINT('Ctrl Pts',(131.781505969283,-22.8951850410383,12.3268777552912));
#31250=CARTESIAN_POINT('Ctrl Pts',(132.617524671433,-22.7537733940447,12.5818558368984));
#31251=CARTESIAN_POINT('Ctrl Pts',(134.309748721346,-22.5643527281993,12.9184862150897));
#31252=CARTESIAN_POINT('Ctrl Pts',(135.166017064757,-22.5166604983954,13.));
#31253=CARTESIAN_POINT('Ctrl Pts',(136.833982935243,-22.5166604983954,13.));
#31254=CARTESIAN_POINT('Ctrl Pts',(137.690251278654,-22.5643527281993,12.9184862150897));
#31255=CARTESIAN_POINT('Ctrl Pts',(139.382475328567,-22.7537733940447,12.5818558368984));
#31256=CARTESIAN_POINT('Ctrl Pts',(140.218494030717,-22.8951850410383,12.3268777552912));
#31257=CARTESIAN_POINT('Ctrl Pts',(142.611570673602,-23.4155481619888,11.325973226571));
#31258=CARTESIAN_POINT('Ctrl Pts',(144.052950545147,-23.8901060781349,10.3318257657035));
#31259=CARTESIAN_POINT('Ctrl Pts',(146.328719603369,-24.7502659309165,8.05605670748142));
#31260=CARTESIAN_POINT('Ctrl Pts',(147.32514603902,-25.1974429335132,6.61362985548688));
#31261=CARTESIAN_POINT('Ctrl Pts',(148.327434591979,-25.6686324247972,4.21712194988807));
#31262=CARTESIAN_POINT('Ctrl Pts',(148.582552741345,-25.7933948769122,3.37993305619291));
#31263=CARTESIAN_POINT('Ctrl Pts',(148.918892814918,-25.9591289790221,1.68724313385082));
#31264=CARTESIAN_POINT('Ctrl Pts',(149.,-26.,0.831709457206481));
#31265=CARTESIAN_POINT('Ctrl Pts',(149.,-26.,2.22044604925031E-15));
#31266=CARTESIAN_POINT('Origin',(124.,0.,10.));
#31267=CARTESIAN_POINT('Ctrl Pts',(115.,4.35889894354066,25.6320112359526));
#31268=CARTESIAN_POINT('Ctrl Pts',(115.497714669606,5.38655112921263,25.4572519482316));
#31269=CARTESIAN_POINT('Ctrl Pts',(116.172977789672,6.31511341340259,25.2336373509982));
#31270=CARTESIAN_POINT('Ctrl Pts',(117.809882463292,7.9520180870225,24.7710207384202));
#31271=CARTESIAN_POINT('Ctrl Pts',(118.925456325839,8.7191257276253,24.500550059198));
#31272=CARTESIAN_POINT('Ctrl Pts',(121.384603519825,9.74339902991552,24.1115387621796));
#31273=CARTESIAN_POINT('Ctrl Pts',(122.729514475929,10.,24.));
#31274=CARTESIAN_POINT('Ctrl Pts',(125.270485524071,10.,24.));
#31275=CARTESIAN_POINT('Ctrl Pts',(126.615396480175,9.74339902991553,24.1115387621796));
#31276=CARTESIAN_POINT('Ctrl Pts',(129.074543674161,8.71912572762531,24.500550059198));
#31277=CARTESIAN_POINT('Ctrl Pts',(130.190117536708,7.9520180870225,24.7710207384202));
#31278=CARTESIAN_POINT('Ctrl Pts',(131.95126588442,6.19086973931097,25.2687506893427));
#31279=CARTESIAN_POINT('Ctrl Pts',(132.718946209375,5.07500736860867,25.5302046420434));
#31280=CARTESIAN_POINT('Ctrl Pts',(133.743654926725,2.61474940838325,25.8980720227517));
#31281=CARTESIAN_POINT('Ctrl Pts',(134.,1.2694007153771,26.));
#31282=CARTESIAN_POINT('Ctrl Pts',(134.,-1.26940071537709,26.));
#31283=CARTESIAN_POINT('Ctrl Pts',(133.743654926725,-2.61474940838325,25.8980720227516));
#31284=CARTESIAN_POINT('Ctrl Pts',(132.718946209375,-5.07500736860866,25.5302046420434));
#31285=CARTESIAN_POINT('Ctrl Pts',(131.95126588442,-6.19086973931097,25.2687506893427));
#31286=CARTESIAN_POINT('Ctrl Pts',(130.190117536708,-7.95201808702249,24.7710207384202));
#31287=CARTESIAN_POINT('Ctrl Pts',(129.074543674161,-8.7191257276253,24.500550059198));
#31288=CARTESIAN_POINT('Ctrl Pts',(126.615396480175,-9.74339902991553,24.1115387621796));
#31289=CARTESIAN_POINT('Ctrl Pts',(125.270485524071,-10.,24.));
#31290=CARTESIAN_POINT('Ctrl Pts',(124.,-10.,24.));
#31291=CARTESIAN_POINT('Ctrl Pts',(122.729514475929,-10.,24.));
#31292=CARTESIAN_POINT('Ctrl Pts',(121.384603519825,-9.74339902991552,24.1115387621796));
#31293=CARTESIAN_POINT('Ctrl Pts',(118.925456325839,-8.7191257276253,24.500550059198));
#31294=CARTESIAN_POINT('Ctrl Pts',(117.809882463292,-7.9520180870225,24.7710207384202));
#31295=CARTESIAN_POINT('Ctrl Pts',(116.172977789672,-6.31511341340259,25.2336373509982));
#31296=CARTESIAN_POINT('Ctrl Pts',(115.497714669606,-5.38655112921264,25.4572519482316));
#31297=CARTESIAN_POINT('Ctrl Pts',(115.,-4.35889894354067,25.6320112359526));
#31298=CARTESIAN_POINT('Origin',(136.,-14.,0.));
#31299=CARTESIAN_POINT('Origin',(124.,0.,14.));
#31300=CARTESIAN_POINT('Origin',(108.,-5.5,34.));
#31301=CARTESIAN_POINT('',(104.95,-4.9,34.));
#31302=CARTESIAN_POINT('Origin',(108.,-4.9,34.));
#31303=CARTESIAN_POINT('',(104.95,4.9,34.));
#31304=CARTESIAN_POINT('',(104.95,-5.5,34.));
#31305=CARTESIAN_POINT('Origin',(108.,4.9,34.));
#31306=CARTESIAN_POINT('Origin',(121.,0.,0.));
#31307=CARTESIAN_POINT('',(93.,-26.,-3.18408167778312E-15));
#31308=CARTESIAN_POINT('',(121.,-26.,-3.18408167778312E-15));
#31309=CARTESIAN_POINT('Origin',(93.,0.,0.));
#31310=CARTESIAN_POINT('',(121.,-4.9,25.5340948537441));
#31311=CARTESIAN_POINT('',(121.,4.9,25.5340948537441));
#31312=CARTESIAN_POINT('Origin',(108.,-4.9,30.5));
#31313=CARTESIAN_POINT('Origin',(108.,4.9,30.5));
#31314=CARTESIAN_POINT('Origin',(89.,0.,0.));
#31315=CARTESIAN_POINT('',(68.,-18.,-2.20436423846524E-15));
#31316=CARTESIAN_POINT('',(89.,-18.,-2.20436423846524E-15));
#31317=CARTESIAN_POINT('Origin',(68.,0.,0.));
#31318=CARTESIAN_POINT('Origin',(68.,20.2,0.));
#31319=CARTESIAN_POINT('',(68.,-20.2,-2.47378653427765E-15));
#31320=CARTESIAN_POINT('Origin',(68.,0.,0.));
#31321=CARTESIAN_POINT('Origin',(68.4,0.,0.));
#31322=CARTESIAN_POINT('',(68.4,-20.6,-2.52277240624355E-15));
#31323=CARTESIAN_POINT('Origin',(80.4,0.,0.));
#31324=CARTESIAN_POINT('Origin',(92.,0.,0.));
#31325=CARTESIAN_POINT('Origin',(92.,25.,0.));
#31326=CARTESIAN_POINT('',(92.,-25.,-3.06161699786838E-15));
#31327=CARTESIAN_POINT('Origin',(92.,0.,0.));
#31328=CARTESIAN_POINT('Origin',(92.5,0.,0.));
#31329=CARTESIAN_POINT('',(92.5,-25.5,-3.12284933782575E-15));
#31330=CARTESIAN_POINT('Origin',(165.6,0.,0.));
#31331=CARTESIAN_POINT('',(165.6,-16.1,-1.97168134662724E-15));
#45195=UNCERTAINTY_MEASURE_WITH_UNIT(LENGTH_MEASURE(0.01),#45237,
'DISTANCE_ACCURACY_VALUE',
'Maximum model space distance between geometric entities at asserted c
onnectivities');
#45214=UNCERTAINTY_MEASURE_WITH_UNIT(LENGTH_MEASURE(0.01),#45237,
'DISTANCE_ACCURACY_VALUE',
'Maximum model space distance between geometric entities at asserted c
onnectivities');
#45217=(
GEOMETRIC_REPRESENTATION_CONTEXT(3)
GLOBAL_UNCERTAINTY_ASSIGNED_CONTEXT((#45195))
GLOBAL_UNIT_ASSIGNED_CONTEXT((#45237,#45239,#45240))
REPRESENTATION_CONTEXT('','3D')
);
#45236=(
GEOMETRIC_REPRESENTATION_CONTEXT(3)
GLOBAL_UNCERTAINTY_ASSIGNED_CONTEXT((#45214))
GLOBAL_UNIT_ASSIGNED_CONTEXT((#45237,#45239,#45240))
REPRESENTATION_CONTEXT('','3D')
);
#45237=(
LENGTH_UNIT()
NAMED_UNIT(*)
SI_UNIT(.MILLI.,.METRE.)
);
#45239=(
NAMED_UNIT(*)
PLANE_ANGLE_UNIT()
SI_UNIT($,.RADIAN.)
);
#45240=(
NAMED_UNIT(*)
SI_UNIT($,.STERADIAN.)
SOLID_ANGLE_UNIT()
);
#45243=SHAPE_DEFINITION_REPRESENTATION(#45264,#45315);
#45264=PRODUCT_DEFINITION_SHAPE('',$,#45337);
#45315=SHAPE_REPRESENTATION('',(#16969),#45217);
#45334=PRODUCT_DEFINITION_CONTEXT('part definition',#45399,'design');
#45337=PRODUCT_DEFINITION('2026-10-25-23-38-13-511',
'02_Hydraulic_Cylinder_Body',#45358,#45334);
#45358=PRODUCT_DEFINITION_FORMATION('',$,#45403);
#45399=APPLICATION_CONTEXT(
'Core Data for Automotive Mechanical Design Process');
#45400=PRODUCT_CONTEXT('part definition',#45399,'mechanical');
#45403=PRODUCT('2026-10-25-23-38-13-511','02_Hydraulic_Cylinder_Body',$,
(#45400));
#45457=COLOUR_RGB('Dark Blue',0.08,0.2,0.34);
#45458=FILL_AREA_STYLE_COLOUR('',#45457);
#45459=FILL_AREA_STYLE('',(#45458));
#45460=SURFACE_STYLE_FILL_AREA(#45459);
#45461=SURFACE_SIDE_STYLE('',(#45460));
#45462=SURFACE_STYLE_USAGE(.BOTH.,#45461);
#45463=PRESENTATION_STYLE_ASSIGNMENT((#45462));
ENDSEC;
END-ISO-10303-21;
